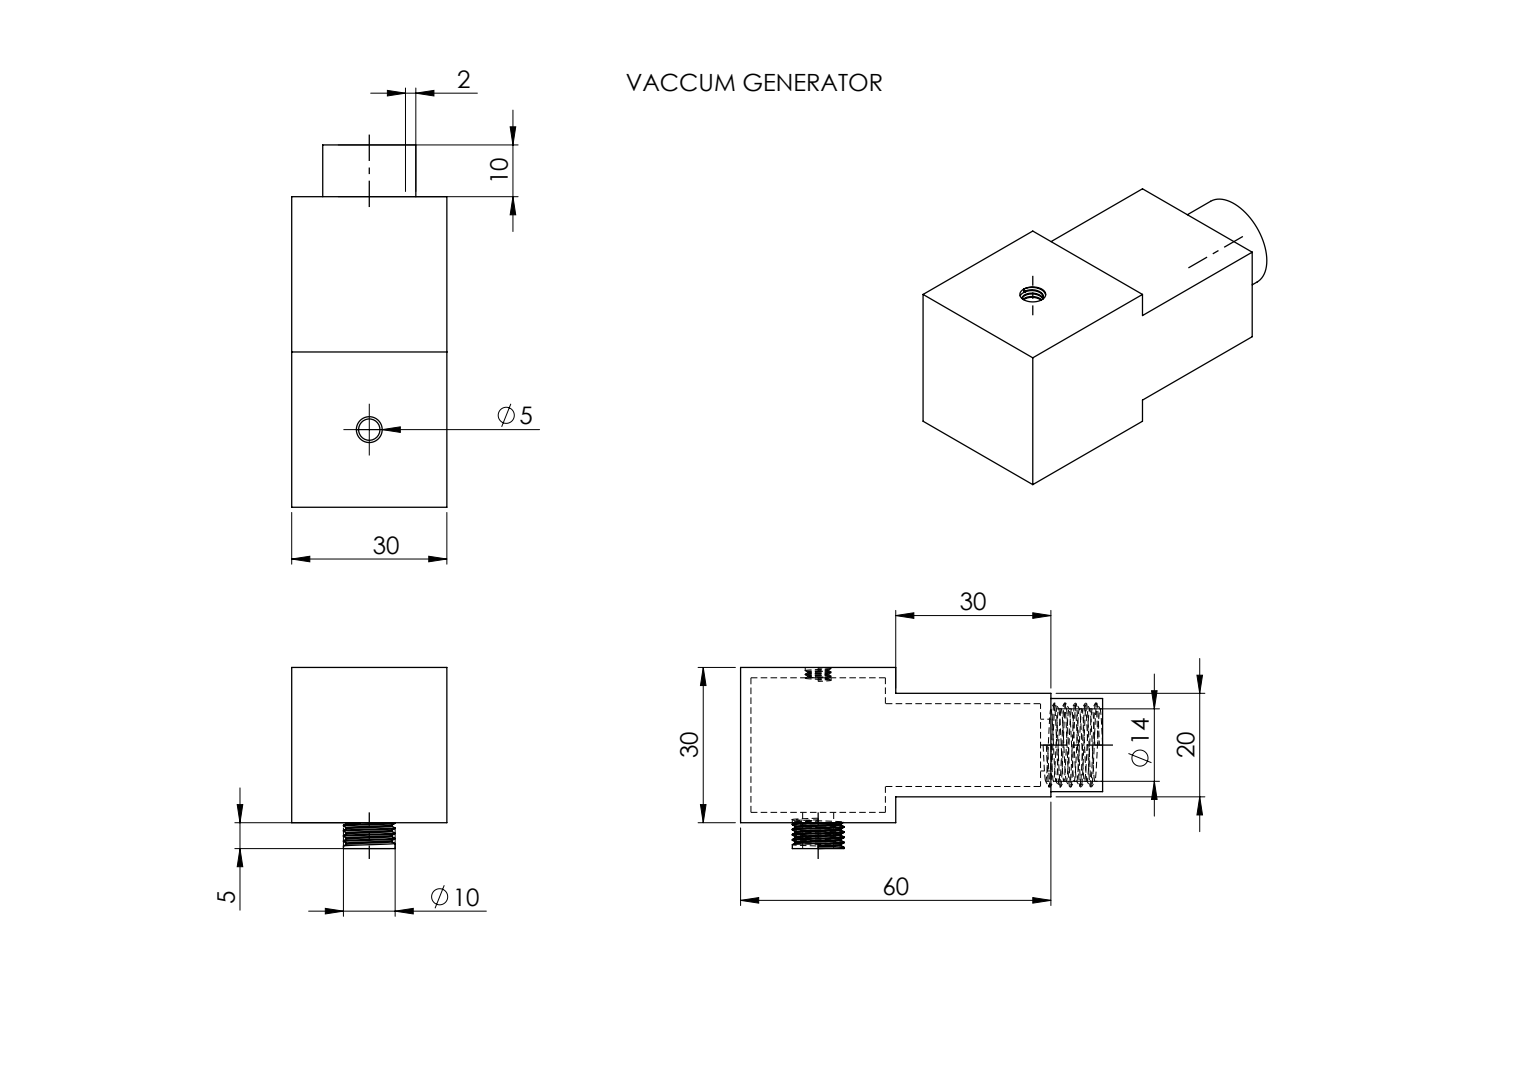
ISO-10303-21;
HEADER;
FILE_DESCRIPTION (('STEP AP214'),
    '1' );
FILE_NAME ('vaccum generator.step',
    '2026-10-01T14:18:43',
    ( '' ),
    ( '' ),
    'SwSTEP 2.0',
    'SolidWorks 2026',
    '' );
FILE_SCHEMA (( 'AUTOMOTIVE_DESIGN' ));
ENDSEC;

DATA;
#3=CARTESIAN_POINT ( 'NONE',  ( 103.1528011352953484, 93.43749999863440792, -3.152801135295366208 ) ) ;
#11=VERTEX_POINT ( 'NONE', #12909 ) ;
#21=VECTOR ( 'NONE', #21803, 1000.000000000000000 ) ;
#28=CARTESIAN_POINT ( 'NONE',  ( 104.9952793366501851, 116.8754121666685393, -49.82500000273120122 ) ) ;
#37=CARTESIAN_POINT ( 'NONE',  ( 102.0669872999999797, 123.3500000010924680, -9.794112055954760458E-15 ) ) ;
#38=LINE ( 'NONE', #22552, #12466 ) ;
#44=EDGE_CURVE ( 'NONE', #13519, #7822, #26113, .T. ) ;
#46=CARTESIAN_POINT ( 'NONE',  ( 93.00000000000001421, 112.2744378736303332, -50.10000000000000142 ) ) ;
#49=CARTESIAN_POINT ( 'NONE',  ( 97.93301269999999192, 123.9000000010924794, -0.8561741729129505041 ) ) ;
#53=CARTESIAN_POINT ( 'NONE',  ( 103.5355339059327235, 93.74999999726881583, 3.535533905932724874 ) ) ;
#67=( BOUNDED_CURVE ( )  B_SPLINE_CURVE ( 2, ( #19739, #26449, #6767, #8908, #2228, #15452, #13444, #6906, #10892, #17316, #24023, #2505, #15595, #2083, #2648, #15160, #20032, #19600, #512, #9193, #17887, #26593, #10752, #19463, #28160, #8627, #4357, #13014, #83, #8766, #26155, #15308, #18836, #13875, #8143, #13592, #5879, #15877, #16700, #11735, #22314, #20460, #11453, #942, #10262, #12398, #21119, #26883, #22601, #3070, #26736, #2788, #23265, #20986, #13733, #1606, #24872, #14549, #18972, #27680, #27543, #16017, #5355, #24587, #4929, #7329, #18022, #20174, #9613, #9328, #8000, #3738, #7180, #1467, #25399, #5069, #16837, #655, #16165, #22457, #2923, #10123, #18316, #14410, #27025, #11593, #20313, #7470, #800, #9469, #23126, #18171, #3601, #24731, #5211, #12261, #10683, #8842, #23398, #23956, #8558 ),
 .UNSPECIFIED., .F., .F. ) 
 B_SPLINE_CURVE_WITH_KNOTS ( ( 3, 2, 2, 2, 2, 2, 2, 2, 2, 2, 2, 2, 2, 2, 2, 2, 2, 2, 2, 2, 2, 2, 2, 2, 2, 2, 2, 2, 2, 2, 2, 2, 2, 2, 2, 2, 2, 2, 2, 2, 2, 2, 2, 2, 2, 2, 2, 2, 2, 2, 3 ),
 ( 0.000000000000000000, 0.02000000000000000042, 0.04000000000000000083, 0.05999999999999999778, 0.08000000000000000167, 0.1000000000000000056, 0.1199999999999999956, 0.1400000000000000133, 0.1600000000000000033, 0.1799999999999999933, 0.2000000000000000111, 0.2200000000000000011, 0.2399999999999999911, 0.2600000000000000089, 0.2800000000000000266, 0.2999999999999999889, 0.3200000000000000067, 0.3400000000000000244, 0.3599999999999999867, 0.3800000000000000044, 0.4000000000000000222, 0.4199999999999999845, 0.4400000000000000022, 0.4600000000000000200, 0.4799999999999999822, 0.5000000000000000000, 0.5200000000000000178, 0.5400000000000000355, 0.5600000000000000533, 0.5799999999999999600, 0.5999999999999999778, 0.6199999999999999956, 0.6400000000000000133, 0.6600000000000000311, 0.6800000000000000488, 0.6999999999999999556, 0.7199999999999999734, 0.7399999999999999911, 0.7600000000000000089, 0.7800000000000000266, 0.8000000000000000444, 0.8199999999999999512, 0.8399999999999999689, 0.8599999999999999867, 0.8800000000000000044, 0.9000000000000000222, 0.9200000000000000400, 0.9399999999999999467, 0.9599999999999999645, 0.9799999999999999822, 1.000000000000000000 ),
 .UNSPECIFIED. ) 
 CURVE ( )  GEOMETRIC_REPRESENTATION_ITEM ( )  RATIONAL_B_SPLINE_CURVE ( ( 1.000000000000000000, 0.9510565162951535312, 1.000000000000000000, 0.9510565162951535312, 1.000000000000000000, 0.9510565162951535312, 1.000000000000000000, 0.9510565162951535312, 1.000000000000000000, 0.9510565162951535312, 1.000000000000000000, 0.9510565162951535312, 1.000000000000000000, 0.9510565162951535312, 1.000000000000000000, 0.9510565162951535312, 1.000000000000000000, 0.9510565162951535312, 1.000000000000000000, 0.9510565162951535312, 1.000000000000000000, 0.9510565162951535312, 1.000000000000000000, 0.9510565162951535312, 1.000000000000000000, 0.9510565162951535312, 1.000000000000000000, 0.9510565162951535312, 1.000000000000000000, 0.9510565162951535312, 1.000000000000000000, 0.9510565162951535312, 1.000000000000000000, 0.9510565162951535312, 1.000000000000000000, 0.9510565162951535312, 1.000000000000000000, 0.9510565162951535312, 1.000000000000000000, 0.9510565162951535312, 1.000000000000000000, 0.9510565162951535312, 1.000000000000000000, 0.9510565162951535312, 1.000000000000000000, 0.9510565162951535312, 1.000000000000000000, 0.9510565162951535312, 1.000000000000000000, 0.9510565162951535312, 1.000000000000000000, 0.9510565162951535312, 1.000000000000000000, 0.9510565162951535312, 1.000000000000000000, 0.9510565162951535312, 1.000000000000000000, 0.9510565162951535312, 1.000000000000000000, 0.9510565162951535312, 1.000000000000000000, 0.9510565162951535312, 1.000000000000000000, 0.9510565162951535312, 1.000000000000000000, 0.9510565162951535312, 1.000000000000000000, 0.9510565162951535312, 1.000000000000000000, 0.9510565162951535312, 1.000000000000000000, 0.9510565162951535312, 1.000000000000000000, 0.9510565162951535312, 1.000000000000000000, 0.9510565162951535312, 1.000000000000000000, 0.9510565162951535312, 1.000000000000000000, 0.9510565162951535312, 1.000000000000000000, 0.9510565162951535312, 1.000000000000000000, 0.9510565162951535312, 1.000000000000000000, 0.9510565162951535312, 1.000000000000000000, 0.9510565162951535312, 1.000000000000000000, 0.9510565162951535312, 1.000000000000000000, 0.9510565162951535312, 1.000000000000000000, 0.9510565162951535312, 1.000000000000000000, 0.9510565162951535312, 1.000000000000000000, 0.9510565162951535312, 1.000000000000000000, 0.9510565162951535312, 1.000000000000000000 ) ) 
 REPRESENTATION_ITEM ( '' )  );
#71=EDGE_CURVE ( 'NONE', #7474, #9199, #1741, .T. ) ;
#83=CARTESIAN_POINT ( 'NONE',  ( 93.46109445667491400, 114.7507929638356785, -51.32500000273120122 ) ) ;
#86=CARTESIAN_POINT ( 'NONE',  ( 84.99999999999998579, 100.0000000000000000, -15.00000000000000533 ) ) ;
#87=CARTESIAN_POINT ( 'NONE',  ( 101.7677669529663547, 123.8000000021849587, 1.767766952966350891 ) ) ;
#93=CARTESIAN_POINT ( 'NONE',  ( 102.0669872999999797, 122.5500000010924850, -9.794112055954760458E-15 ) ) ;
#95=LINE ( 'NONE', #11320, #20973 ) ;
#101=CARTESIAN_POINT ( 'NONE',  ( 108.0825317500000011, 112.6261737610028320, -50.02500000273118275 ) ) ;
#116=EDGE_CURVE ( 'NONE', #24967, #25660, #21271, .T. ) ;
#120=CARTESIAN_POINT ( 'NONE',  ( 104.9999999999999716, 92.93749999999998579, 2.071067811865467956 ) ) ;
#125=CARTESIAN_POINT ( 'NONE',  ( 99.99999999999998579, 117.3602355696678643, -54.50000000000000000 ) ) ;
#129=CARTESIAN_POINT ( 'NONE',  ( 106.5389055433251002, 105.2492070361643215, -44.57500000273119412 ) ) ;
#130=CARTESIAN_POINT ( 'NONE',  ( 104.3262379212492590, 115.9545556584642867, -45.20000000546237828 ) ) ;
#133=CARTESIAN_POINT ( 'NONE',  ( 102.1631189606246295, 116.6573956140660897, -45.10000000546238397 ) ) ;
#134=CARTESIAN_POINT ( 'NONE',  ( 98.15313185440925281, 94.99999999863439371, 4.458734124999979898 ) ) ;
#142=CARTESIAN_POINT ( 'NONE',  ( 96.84719886470463734, 92.93749999863440792, 3.152801135295351997 ) ) ;
#155=UNCERTAINTY_MEASURE_WITH_UNIT (LENGTH_MEASURE( 1.000000000000000082E-05 ), #20072, 'distance_accuracy_value', 'NONE');
#159=CARTESIAN_POINT ( 'NONE',  ( 103.5355338419364699, 95.00000000000001421, -3.535533969929001596 ) ) ;
#171=CARTESIAN_POINT ( 'NONE',  ( 93.46109445667491400, 114.7507929638356785, -51.32500000273120122 ) ) ;
#179=CARTESIAN_POINT ( 'NONE',  ( 84.99999999999998579, 120.0000000000000000, -45.00000000000000711 ) ) ;
#182=EDGE_LOOP ( 'NONE', ( #354, #23980, #3469, #3062 ) ) ;
#187=CARTESIAN_POINT ( 'NONE',  ( 97.83688103937538472, 116.6573956140660897, -48.40000000000000568 ) ) ;
#189=FACE_OUTER_BOUND ( 'NONE', #22000, .T. ) ;
#192=CARTESIAN_POINT ( 'NONE',  ( 95.00000000000000000, 93.31249999726880162, -2.071067811865479058 ) ) ;
#196=ORIENTED_EDGE ( 'NONE', *, *, #21889, .T. ) ;
#210=VERTEX_POINT ( 'NONE', #12459 ) ;
#213=ORIENTED_EDGE ( 'NONE', *, *, #13961, .F. ) ;
#221=DIRECTION ( 'NONE',  ( 1.000000000000000000, 0.000000000000000000, 0.000000000000000000 ) ) ;
#225=CARTESIAN_POINT ( 'NONE',  ( 97.50000000000000000, 124.3184775928351655, 0.3826834323650784575 ) ) ;
#230=CARTESIAN_POINT ( 'NONE',  ( 101.0355339059327378, 122.4500000021849502, -2.499999999999997780 ) ) ;
#237=CARTESIAN_POINT ( 'NONE',  ( 91.91746824999998466, 107.3738262389971538, -51.02500000273119696 ) ) ;
#245=CARTESIAN_POINT ( 'NONE',  ( 112.9999999999999858, 120.0000000000000000, -43.00000000000000000 ) ) ;
#255=LINE ( 'NONE', #20201, #25320 ) ;
#264=DIRECTION ( 'NONE',  ( 0.000000000000000000, -1.000000000000000000, 0.000000000000000000 ) ) ;
#275=CARTESIAN_POINT ( 'NONE',  ( 102.4999999999999858, 123.0000000000000000, -8.724596124144689908E-15 ) ) ;
#276=ORIENTED_EDGE ( 'NONE', *, *, #2418, .F. ) ;
#286=CARTESIAN_POINT ( 'NONE',  ( 98.15313185440925281, 92.99999999863439371, 4.458734124999979898 ) ) ;
#288=EDGE_CURVE ( 'NONE', #11725, #11898, #16264, .T. ) ;
#312=CARTESIAN_POINT ( 'NONE',  ( 102.4976396683250925, 102.3130555110000159, -44.52500000273119696 ) ) ;
#314=FACE_OUTER_BOUND ( 'NONE', #8408, .T. ) ;
#322=CARTESIAN_POINT ( 'NONE',  ( 102.0669872999999797, 122.5500000010924850, -9.794112055954760458E-15 ) ) ;
#323=FACE_OUTER_BOUND ( 'NONE', #26669, .T. ) ;
#330=CARTESIAN_POINT ( 'NONE',  ( 95.00472066334982912, 116.8754121666685393, -51.67500000273118133 ) ) ;
#332=CARTESIAN_POINT ( 'NONE',  ( 101.4615807364564546, 122.8500000010924680, -1.461580736456474794 ) ) ;
#335=CARTESIAN_POINT ( 'NONE',  ( 96.46446609406726225, 92.24999999726880162, -3.535533905932738197 ) ) ;
#341=ORIENTED_EDGE ( 'NONE', *, *, #1476, .T. ) ;
#354=ORIENTED_EDGE ( 'NONE', *, *, #7968, .T. ) ;
#359=AXIS2_PLACEMENT_3D ( 'NONE', #24146, #26286, #22010 ) ;
#370=VERTEX_POINT ( 'NONE', #20912 ) ;
#372=CARTESIAN_POINT ( 'NONE',  ( 102.4999999999999858, 122.2813376356282191, 0.3865102666887284544 ) ) ;
#377=CARTESIAN_POINT ( 'NONE',  ( 99.99999999999998579, 122.9000000021849530, 2.499999999999978684 ) ) ;
#379=AXIS2_PLACEMENT_3D ( 'NONE', #4372, #22042, #19613 ) ;
#381=CARTESIAN_POINT ( 'NONE',  ( 84.99999999999998579, 99.99999999999998579, -45.00000000000000711 ) ) ;
#384=CARTESIAN_POINT ( 'NONE',  ( 99.99999999999998579, 118.4984768113314004, -53.62500000273119127 ) ) ;
#387=DIRECTION ( 'NONE',  ( 0.000000000000000000, 0.000000000000000000, -1.000000000000000000 ) ) ;
#419=CARTESIAN_POINT ( 'NONE',  ( 100.8031273896213378, 123.0000000000000000, 2.371931796629188405 ) ) ;
#420=CARTESIAN_POINT ( 'NONE',  ( 99.99999999999998579, 92.12499999726880162, -4.999999999999997335 ) ) ;
#427=CARTESIAN_POINT ( 'NONE',  ( 96.84719886470463734, 94.68749999863440792, -3.152801135295366208 ) ) ;
#429=CARTESIAN_POINT ( 'NONE',  ( 95.54126587499999346, 94.99999999863439371, -1.846868145590737864 ) ) ;
#434=DIRECTION ( 'NONE',  ( 0.000000000000000000, 1.000000000000000000, -1.156482317317871478E-16 ) ) ;
#446=EDGE_CURVE ( 'NONE', #27429, #27080, #21214, .T. ) ;
#455=CARTESIAN_POINT ( 'NONE',  ( 99.99999999999998579, 118.4984768113314004, -45.62500000273118417 ) ) ;
#464=CARTESIAN_POINT ( 'NONE',  ( 102.0669873000000081, 123.3000000010924850, 0.8561741729129311862 ) ) ;
#465=DIRECTION ( 'NONE',  ( 0.000000000000000000, 0.000000000000000000, 1.000000000000000000 ) ) ;
#471=VECTOR ( 'NONE', #27075, 1000.000000000000000 ) ;
#473=CARTESIAN_POINT ( 'NONE',  ( 107.0000000000000142, 110.0000000000000000, -47.00000000000000711 ) ) ;
#475=CARTESIAN_POINT ( 'NONE',  ( 101.0355339059327378, 123.1499999999999915, -2.499999999999997780 ) ) ;
#476=EDGE_CURVE ( 'NONE', #26599, #20388, #21898, .T. ) ;
#480=CARTESIAN_POINT ( 'NONE',  ( 104.9999999999999716, 94.81249999726880162, 2.071067811865467956 ) ) ;
#483=CARTESIAN_POINT ( 'NONE',  ( 108.0825317500000153, 110.0000000000000000, -52.37500000273119838 ) ) ;
#484=EDGE_CURVE ( 'NONE', #26503, #20101, #13985, .T. ) ;
#486=CARTESIAN_POINT ( 'NONE',  ( 102.4999999999999858, 123.1000000021849416, -9.847140817659276890E-15 ) ) ;
#490=( BOUNDED_CURVE ( )  B_SPLINE_CURVE ( 2, ( #3629, #3902, #12290, #3485, #23428, #25141, #19000, #10438, #9887 ),
 .UNSPECIFIED., .F., .F. ) 
 B_SPLINE_CURVE_WITH_KNOTS ( ( 3, 2, 2, 2, 3 ),
 ( 0.4500000000000003997, 0.4750000000000003664, 0.5000000000000004441, 0.5250000000000004663, 0.5500000000000004885 ),
 .UNSPECIFIED. ) 
 CURVE ( )  GEOMETRIC_REPRESENTATION_ITEM ( )  RATIONAL_B_SPLINE_CURVE ( ( 0.9999999999999987788, 0.9238795325112879597, 1.000000000000000000, 0.9238795325112867385, 1.000000000000000000, 0.9238795325112867385, 1.000000000000000000, 0.9238795325112854062, 1.000000000000001332 ) ) 
 REPRESENTATION_ITEM ( '' )  );
#493=EDGE_LOOP ( 'NONE', ( #21611, #13258, #8930, #18827, #22732, #24894, #25682, #24306 ) ) ;
#510=AXIS2_PLACEMENT_3D ( 'NONE', #5908, #18592, #16158 ) ;
#512=CARTESIAN_POINT ( 'NONE',  ( 106.5389055433251002, 105.2492070361643215, -52.32500000273119412 ) ) ;
#516=VECTOR ( 'NONE', #15597, 1000.000000000000000 ) ;
#519=CARTESIAN_POINT ( 'NONE',  ( 102.0669872999999797, 123.3500000010924680, -9.794112055954760458E-15 ) ) ;
#524=CARTESIAN_POINT ( 'NONE',  ( 93.00000000000000000, 110.0000000000000000, -52.50000000546237544 ) ) ;
#526=CARTESIAN_POINT ( 'NONE',  ( 108.0825317500000153, 110.0000000000000000, -46.12500000273119838 ) ) ;
#544=CARTESIAN_POINT ( 'NONE',  ( 102.4999999999999858, 123.9000000021849530, -9.847140817659276890E-15 ) ) ;
#545=DIRECTION ( 'NONE',  ( 0.000000000000000000, 0.000000000000000000, 1.000000000000000000 ) ) ;
#546=DIRECTION ( 'NONE',  ( 1.000000000000000000, 0.000000000000000000, -5.782411586589357392E-17 ) ) ;
#549=CARTESIAN_POINT ( 'NONE',  ( 102.4999999999999716, 124.5569999999781601, 1.035533905932722876 ) ) ;
#551=CARTESIAN_POINT ( 'NONE',  ( 95.00000000000000000, 94.43749999726878741, 2.071067811865463959 ) ) ;
#560=DIRECTION ( 'NONE',  ( 5.782411586589357392E-17, -0.000000000000000000, 1.000000000000000000 ) ) ;
#561=CARTESIAN_POINT ( 'NONE',  ( 84.99999999999998579, 102.0000000000000000, -43.00000000000000000 ) ) ;
#574=CARTESIAN_POINT ( 'NONE',  ( 99.99999999999998579, 93.25000000000000000, -4.999999999999997335 ) ) ;
#575=CARTESIAN_POINT ( 'NONE',  ( 104.4587341249999923, 94.62499999863439371, -1.846868145590737198 ) ) ;
#578=ORIENTED_EDGE ( 'NONE', *, *, #27721, .F. ) ;
#588=LINE ( 'NONE', #8843, #28012 ) ;
#592=DIRECTION ( 'NONE',  ( -5.782411586589357392E-17, 0.000000000000000000, -1.000000000000000000 ) ) ;
#597=CARTESIAN_POINT ( 'NONE',  ( 91.91746824999998466, 107.3738262389971538, -45.02500000273118985 ) ) ;
#598=CARTESIAN_POINT ( 'NONE',  ( 98.15313185440925281, 91.24999999863439371, 4.458734124999979898 ) ) ;
#602=VECTOR ( 'NONE', #8159, 1000.000000000000000 ) ;
#605=CARTESIAN_POINT ( 'NONE',  ( 104.4587341249999781, 90.56249999863440792, -6.938893903907228378E-15 ) ) ;
#606=EDGE_CURVE ( 'NONE', #15224, #13309, #67, .T. ) ;
#607=CARTESIAN_POINT ( 'NONE',  ( 99.99999999999998579, 123.7000000021849502, 2.499999999999978684 ) ) ;
#613=VERTEX_POINT ( 'NONE', #17102 ) ;
#614=CARTESIAN_POINT ( 'NONE',  ( 102.1631189606246295, 116.6573956140660897, -46.60000000000000142 ) ) ;
#616=CARTESIAN_POINT ( 'NONE',  ( 98.23223304703363112, 124.1000000000000085, -1.767766952966370209 ) ) ;
#622=( BOUNDED_CURVE ( )  B_SPLINE_CURVE ( 2, ( #23987, #4050, #21858, #21436, #25840, #8308, #4465, #8730, #16998 ),
 .UNSPECIFIED., .F., .T. ) 
 B_SPLINE_CURVE_WITH_KNOTS ( ( 3, 2, 2, 2, 3 ),
 ( 0.3500000000000003109, 0.3750000000000003331, 0.4000000000000003553, 0.4250000000000003775, 0.4500000000000003997 ),
 .UNSPECIFIED. ) 
 CURVE ( )  GEOMETRIC_REPRESENTATION_ITEM ( )  RATIONAL_B_SPLINE_CURVE ( ( 0.9999999999999990008, 0.9238795325112877377, 1.000000000000000000, 0.9238795325112867385, 1.000000000000000000, 0.9238795325112867385, 1.000000000000000000, 0.9238795325112855172, 1.000000000000001110 ) ) 
 REPRESENTATION_ITEM ( '' )  );
#623=CARTESIAN_POINT ( 'NONE',  ( 97.92893218813452449, 95.56249999726883004, 4.999999999999983125 ) ) ;
#626=CARTESIAN_POINT ( 'NONE',  ( 104.9952793366501709, 103.1245878333314465, -50.67500000273119554 ) ) ;
#628=DIRECTION ( 'NONE',  ( 0.000000000000000000, -1.000000000000000000, 0.000000000000000000 ) ) ;
#638=CARTESIAN_POINT ( 'NONE',  ( 99.99999999999998579, 91.31249999863440792, 4.458734124999981674 ) ) ;
#641=ORIENTED_EDGE ( 'NONE', *, *, #1027, .F. ) ;
#650=ORIENTED_EDGE ( 'NONE', *, *, #4627, .F. ) ;
#655=CARTESIAN_POINT ( 'NONE',  ( 104.9952793366501709, 103.1245878333314465, -46.42500000273119554 ) ) ;
#670=CARTESIAN_POINT ( 'NONE',  ( 96.84719886470463734, 92.68749999863440792, -3.152801135295366208 ) ) ;
#671=CARTESIAN_POINT ( 'NONE',  ( 108.0825317500000153, 110.0000000000000000, -48.12500000273119838 ) ) ;
#678=ORIENTED_EDGE ( 'NONE', *, *, #24104, .F. ) ;
#685=CYLINDRICAL_SURFACE ( 'NONE', #17971, 7.000000000000006217 ) ;
#689=AXIS2_PLACEMENT_3D ( 'NONE', #15191, #26185, #8519 ) ;
#693=CARTESIAN_POINT ( 'NONE',  ( 98.96446609406727646, 124.3569999999781430, 2.499999999999977796 ) ) ;
#697=DIRECTION ( 'NONE',  ( 0.000000000000000000, 0.000000000000000000, -1.000000000000000000 ) ) ;
#704=DIRECTION ( 'NONE',  ( 0.000000000000000000, 0.000000000000000000, 1.000000000000000000 ) ) ;
#706=CARTESIAN_POINT ( 'NONE',  ( 106.5389055433251002, 105.2492070361643215, -52.57500000273119412 ) ) ;
#716=CARTESIAN_POINT ( 'NONE',  ( 96.46446609406726225, 91.62500000000000000, 3.535533905932723986 ) ) ;
#723=CARTESIAN_POINT ( 'NONE',  ( 96.46446609406726225, 95.24999999726881583, -3.535533905932738197 ) ) ;
#724=B_SPLINE_CURVE_WITH_KNOTS ( 'NONE', 3,
 ( #27392, #24818, #7851, #20969 ),
 .UNSPECIFIED., .F., .F.,
 ( 4, 4 ),
 ( 0.000000000000000000, 1.000000000000000000 ),
 .UNSPECIFIED. ) ;
#730=LINE ( 'NONE', #20110, #16690 ) ;
#734=CARTESIAN_POINT ( 'NONE',  ( 107.0000000000000142, 110.0000000000000000, -49.50000000546238255 ) ) ;
#735=CARTESIAN_POINT ( 'NONE',  ( 101.8468681455907330, 91.49999999863440792, -4.458734124999994997 ) ) ;
#741=CARTESIAN_POINT ( 'NONE',  ( 93.00000000000000000, 110.0000000000000000, -52.50000000546237544 ) ) ;
#744=DIRECTION ( 'NONE',  ( -5.782411586589357392E-17, -0.000000000000000000, -1.000000000000000000 ) ) ;
#749=( BOUNDED_CURVE ( )  B_SPLINE_CURVE ( 2, ( #24281, #4762, #20290, #13422, #20439 ),
 .UNSPECIFIED., .F., .F. ) 
 B_SPLINE_CURVE_WITH_KNOTS ( ( 3, 2, 3 ),
 ( 0.000000000000000000, 0.02500000000000002220, 0.05000000000000004441 ),
 .UNSPECIFIED. ) 
 CURVE ( )  GEOMETRIC_REPRESENTATION_ITEM ( )  RATIONAL_B_SPLINE_CURVE ( ( 1.000000000000000000, 0.9238795325112867385, 1.000000000000000000, 0.9238795325112866275, 1.000000000000000222 ) ) 
 REPRESENTATION_ITEM ( '' )  );
#751=CARTESIAN_POINT ( 'NONE',  ( 97.50000000000000000, 123.4500000021849502, -1.035533905932742416 ) ) ;
#756=VERTEX_POINT ( 'NONE', #28095 ) ;
#757=CARTESIAN_POINT ( 'NONE',  ( 93.46109445667491400, 105.2492070361643215, -51.17500000273119554 ) ) ;
#760=CARTESIAN_POINT ( 'NONE',  ( 101.0355339059327378, 123.6500000000000199, 2.499999999999977796 ) ) ;
#761=CARTESIAN_POINT ( 'NONE',  ( 99.99999999999998579, 94.75000000000000000, 4.999999999999984013 ) ) ;
#765=CARTESIAN_POINT ( 'NONE',  ( 95.54126587499999346, 93.99999999863439371, -1.846868145590737864 ) ) ;
#767=CARTESIAN_POINT ( 'NONE',  ( 91.91746824999998466, 112.6261737610028320, -53.47500000273119980 ) ) ;
#776=CARTESIAN_POINT ( 'NONE',  ( 99.99999999999998579, 124.7999999999999972, -2.499999999999997780 ) ) ;
#783=CARTESIAN_POINT ( 'NONE',  ( 95.54126587500000767, 92.06249999863440792, -7.484931351350258973E-15 ) ) ;
#796=CARTESIAN_POINT ( 'NONE',  ( 99.99999999999998579, 91.62499999726880162, 4.999999999999984013 ) ) ;
#798=AXIS2_PLACEMENT_3D ( 'NONE', #21029, #12723, #5784 ) ;
#800=CARTESIAN_POINT ( 'NONE',  ( 93.46109445667491400, 114.7507929638356785, -45.32500000273119412 ) ) ;
#802=EDGE_CURVE ( 'NONE', #24847, #3863, #10819, .T. ) ;
#816=CARTESIAN_POINT ( 'NONE',  ( 99.99999999999998579, 118.4984768113314004, -47.62500000273119127 ) ) ;
#818=AXIS2_PLACEMENT_3D ( 'NONE', #8800, #11063, #545 ) ;
#821=CARTESIAN_POINT ( 'NONE',  ( 102.0710678118654613, 91.06249999726880162, -4.999999999999997335 ) ) ;
#823=ORIENTED_EDGE ( 'NONE', *, *, #16054, .F. ) ;
#850=EDGE_CURVE ( 'NONE', #21579, #8168, #25534, .T. ) ;
#855=DIRECTION ( 'NONE',  ( 1.000000000000000000, 0.000000000000000000, -5.782411586589357392E-17 ) ) ;
#856=CARTESIAN_POINT ( 'NONE',  ( 102.1049798866730214, 123.0000000000000284, -1.357224074530030800 ) ) ;
#857=EDGE_LOOP ( 'NONE', ( #26118, #7258, #9956, #20270 ) ) ;
#858=CARTESIAN_POINT ( 'NONE',  ( 102.0669872999999797, 124.1500000010924794, -9.794112055954760458E-15 ) ) ;
#865=CARTESIAN_POINT ( 'NONE',  ( 99.99999999999998579, 92.75000000000000000, 4.999999999999984013 ) ) ;
#867=VECTOR ( 'NONE', #8438, 1000.000000000000000 ) ;
#882=CARTESIAN_POINT ( 'NONE',  ( 93.00000000000000000, 110.0000000000000000, -50.50000000546237544 ) ) ;
#886=CARTESIAN_POINT ( 'NONE',  ( 99.99999999999998579, 124.3999999999999915, 2.499999999999978684 ) ) ;
#890=CARTESIAN_POINT ( 'NONE',  ( 104.9952793366501851, 116.8754121666685393, -45.82500000273119412 ) ) ;
#892=CARTESIAN_POINT ( 'NONE',  ( 104.4587341249999923, 91.49999999863440792, 1.846868145590726318 ) ) ;
#897=CARTESIAN_POINT ( 'NONE',  ( 102.3917468249999700, 122.9375000002731184, -9.833883627233146598E-15 ) ) ;
#905=CARTESIAN_POINT ( 'NONE',  ( 106.5389055433251002, 114.7507929638356785, -52.17500000273119554 ) ) ;
#913=CARTESIAN_POINT ( 'NONE',  ( 104.4587341249999781, 92.56249999863440792, -6.938893903907228378E-15 ) ) ;
#915=CARTESIAN_POINT ( 'NONE',  ( 108.0825317500000011, 107.3738262389971680, -48.47500000273118559 ) ) ;
#919=( BOUNDED_CURVE ( )  B_SPLINE_CURVE ( 2, ( #11916, #9919, #25049, #22918, #18636, #14478, #15162, #6218, #16897 ),
 .UNSPECIFIED., .F., .F. ) 
 B_SPLINE_CURVE_WITH_KNOTS ( ( 3, 2, 2, 2, 3 ),
 ( 0.2499999999999998335, 0.2916666666666665741, 0.3333333333333332593, 0.3750000000000000000, 0.4166666666666667407 ),
 .UNSPECIFIED. ) 
 CURVE ( )  GEOMETRIC_REPRESENTATION_ITEM ( )  RATIONAL_B_SPLINE_CURVE ( ( 1.000000000000000222, 0.9238795325112864054, 1.000000000000000000, 0.9238795325112867385, 1.000000000000000000, 0.9238795325112867385, 1.000000000000000000, 0.9238795325112866275, 1.000000000000000000 ) ) 
 REPRESENTATION_ITEM ( '' )  );
#923=VERTEX_POINT ( 'NONE', #159 ) ;
#926=DIRECTION ( 'NONE',  ( 0.000000000000000000, -1.000000000000000000, 0.000000000000000000 ) ) ;
#938=LINE ( 'NONE', #9609, #7507 ) ;
#942=CARTESIAN_POINT ( 'NONE',  ( 104.9952793366501709, 116.8754121666685393, -49.82500000273120122 ) ) ;
#953=CARTESIAN_POINT ( 'NONE',  ( 104.9999999999999716, 94.93749999726880162, -2.071067811865478170 ) ) ;
#955=FACE_OUTER_BOUND ( 'NONE', #4282, .T. ) ;
#957=CARTESIAN_POINT ( 'NONE',  ( 99.99999999999998579, 101.5015231886685854, -46.62500000273119838 ) ) ;
#966=( BOUNDED_CURVE ( )  B_SPLINE_CURVE ( 2, ( #4156, #10263, #18973, #1885, #12817, #21539, #27681, #2016, #10684, #19391, #25951 ),
 .UNSPECIFIED., .F., .F. ) 
 B_SPLINE_CURVE_WITH_KNOTS ( ( 3, 2, 2, 2, 2, 3 ),
 ( 0.3000000000000002109, 0.3200000000000002287, 0.3400000000000003020, 0.3600000000000002642, 0.3800000000000003375, 0.4000000000000003553 ),
 .UNSPECIFIED. ) 
 CURVE ( )  GEOMETRIC_REPRESENTATION_ITEM ( )  RATIONAL_B_SPLINE_CURVE ( ( 0.9999999999999994449, 0.9510565162951540863, 1.000000000000000000, 0.9510565162951535312, 1.000000000000000000, 0.9510565162951535312, 1.000000000000000000, 0.9510565162951535312, 1.000000000000000000, 0.9510565162951527540, 1.000000000000000888 ) ) 
 REPRESENTATION_ITEM ( '' )  );
#986=LINE ( 'NONE', #24204, #26829 ) ;
#997=CARTESIAN_POINT ( 'NONE',  ( 99.99999999999998579, 118.4984768113314004, -53.87500000273118417 ) ) ;
#1003=EDGE_CURVE ( 'NONE', #11898, #11725, #6213, .T. ) ;
#1004=EDGE_LOOP ( 'NONE', ( #28123, #4594, #14143, #20923 ) ) ;
#1005=CARTESIAN_POINT ( 'NONE',  ( 99.99999999999998579, 117.3602355696678643, -50.49999999999999289 ) ) ;
#1008=CARTESIAN_POINT ( 'NONE',  ( 104.9999999999999858, 93.00000000000000000, -6.938893903907228378E-15 ) ) ;
#1026=CARTESIAN_POINT ( 'NONE',  ( 98.15313185440923860, 92.62499999863439371, -4.458734124999994997 ) ) ;
#1027=EDGE_CURVE ( 'NONE', #12839, #23013, #730, .T. ) ;
#1033=CARTESIAN_POINT ( 'NONE',  ( 104.3262379212492590, 104.0454443415356991, -49.80000000546237970 ) ) ;
#1047=CARTESIAN_POINT ( 'NONE',  ( 104.9952793366501851, 116.8754121666685393, -46.07500000273119412 ) ) ;
#1054=CARTESIAN_POINT ( 'NONE',  ( 96.84719886470463734, 93.18749999863440792, 3.152801135295351997 ) ) ;
#1055=FACE_OUTER_BOUND ( 'NONE', #17673, .T. ) ;
#1056=CARTESIAN_POINT ( 'NONE',  ( 104.9952793366501709, 116.8754121666685393, -50.07500000273120122 ) ) ;
#1077=CARTESIAN_POINT ( 'NONE',  ( 99.99999999999998579, 122.9500000010924765, -2.066987299999998751 ) ) ;
#1082=CARTESIAN_POINT ( 'NONE',  ( 95.00000000000000000, 91.37499999726880162, -7.551217303480904118E-15 ) ) ;
#1087=FACE_OUTER_BOUND ( 'NONE', #25613, .T. ) ;
#1091=ORIENTED_EDGE ( 'NONE', *, *, #15947, .T. ) ;
#1104=CARTESIAN_POINT ( 'NONE',  ( 104.9999999999999716, 90.93749999726880162, -2.071067811865478170 ) ) ;
#1127=CARTESIAN_POINT ( 'NONE',  ( 97.71650635000000307, 124.8750000005462368, -9.540979117872439019E-15 ) ) ;
#1140=CARTESIAN_POINT ( 'NONE',  ( 104.4587341249999781, 95.31249999863440792, -6.938893903907228378E-15 ) ) ;
#1142=CARTESIAN_POINT ( 'NONE',  ( 97.93301269999999192, 123.7000000010924765, -0.8561741729129505041 ) ) ;
#1150=CARTESIAN_POINT ( 'NONE',  ( 104.9999999999999716, 91.06249999999997158, -2.071067811865478170 ) ) ;
#1167=CARTESIAN_POINT ( 'NONE',  ( 101.8468681455907330, 91.12499999863439371, 4.458734124999980786 ) ) ;
#1175=CARTESIAN_POINT ( 'NONE',  ( 102.1631189606246295, 116.6573956140660897, -49.10000000546237686 ) ) ;
#1176=CARTESIAN_POINT ( 'NONE',  ( 104.4587341249999923, 93.49999999863442213, 1.846868145590726318 ) ) ;
#1178=LINE ( 'NONE', #18689, #2546 ) ;
#1189=VERTEX_POINT ( 'NONE', #19650 ) ;
#1190=CARTESIAN_POINT ( 'NONE',  ( 108.0825317500000153, 110.0000000000000000, -48.37500000273119838 ) ) ;
#1192=DIRECTION ( 'NONE',  ( 0.000000000000000000, 0.000000000000000000, 1.000000000000000000 ) ) ;
#1197=CARTESIAN_POINT ( 'NONE',  ( 101.8468681455907330, 90.74999999863439371, -4.458734124999994997 ) ) ;
#1208=ORIENTED_EDGE ( 'NONE', *, *, #12780, .T. ) ;
#1211=CARTESIAN_POINT ( 'NONE',  ( 103.1528011352953484, 93.68749999863440792, -3.152801135295366208 ) ) ;
#1214=DIRECTION ( 'NONE',  ( 0.000000000000000000, -1.000000000000000000, 3.469446951953611231E-16 ) ) ;
#1216=VECTOR ( 'NONE', #28178, 999.9999999999998863 ) ;
#1220=CARTESIAN_POINT ( 'NONE',  ( 108.0825317500000153, 110.0000000000000000, -54.25000000273119838 ) ) ;
#1232=( NAMED_UNIT ( * ) SI_UNIT ( $, .STERADIAN. ) SOLID_ANGLE_UNIT ( ) );
#1239=CARTESIAN_POINT ( 'NONE',  ( 87.00000000000000000, 123.0000000000000000, 14.99999999999999112 ) ) ;
#1243=ORIENTED_EDGE ( 'NONE', *, *, #7208, .F. ) ;
#1251=ADVANCED_FACE ( 'NONE', ( #2837, #13927 ), #2972, .F. ) ;
#1254=CARTESIAN_POINT ( 'NONE',  ( 107.0000000000000142, 110.0000000000000000, -47.00000000000000711 ) ) ;
#1259=CARTESIAN_POINT ( 'NONE',  ( 102.4999999999999858, 123.0000000000000000, -9.847140817659276890E-15 ) ) ;
#1273=CARTESIAN_POINT ( 'NONE',  ( 97.50236033167492167, 117.6869444889999841, -47.77500000273119696 ) ) ;
#1275=CARTESIAN_POINT ( 'NONE',  ( 97.93301269999999192, 124.5000000010924879, -0.8561741729129505041 ) ) ;
#1281=DIRECTION ( 'NONE',  ( 0.000000000000000000, 1.000000000000000000, 0.000000000000000000 ) ) ;
#1287=VERTEX_POINT ( 'NONE', #1140 ) ;
#1305=CARTESIAN_POINT ( 'NONE',  ( 107.0000000000000142, 107.7255621263696526, -49.60000000546238397 ) ) ;
#1306=CARTESIAN_POINT ( 'NONE',  ( 95.54126587500000767, 93.06249999863440792, -7.484931351350258973E-15 ) ) ;
#1318=EDGE_CURVE ( 'NONE', #3280, #28194, #19784, .T. ) ;
#1322=EDGE_LOOP ( 'NONE', ( #4647, #13285, #16586, #4240 ) ) ;
#1323=CARTESIAN_POINT ( 'NONE',  ( 93.46109445667491400, 105.2492070361643215, -49.17500000273119554 ) ) ;
#1332=CARTESIAN_POINT ( 'NONE',  ( 104.4587341249999923, 92.49999999863442213, 1.846868145590726318 ) ) ;
#1335=DIRECTION ( 'NONE',  ( 0.000000000000000000, 0.000000000000000000, -1.000000000000000000 ) ) ;
#1349=ADVANCED_FACE ( 'NONE', ( #7672 ), #27789, .T. ) ;
#1351=DIRECTION ( 'NONE',  ( 1.000000000000000000, 0.000000000000000000, 0.000000000000000000 ) ) ;
#1352=ORIENTED_EDGE ( 'NONE', *, *, #16537, .F. ) ;
#1360=CARTESIAN_POINT ( 'NONE',  ( 95.67376207875072680, 115.9545556584642867, -54.30000000000001137 ) ) ;
#1362=DIRECTION ( 'NONE',  ( 0.000000000000000000, -0.000000000000000000, 1.000000000000000000 ) ) ;
#1373=CARTESIAN_POINT ( 'NONE',  ( 104.3262379212492590, 104.0454443415356991, -51.80000000546237970 ) ) ;
#1375=CARTESIAN_POINT ( 'NONE',  ( 102.0710678118654613, 91.68749999726880162, 4.999999999999974243 ) ) ;
#1381=ORIENTED_EDGE ( 'NONE', *, *, #16100, .T. ) ;
#1382=VECTOR ( 'NONE', #2864, 1000.000000000000000 ) ;
#1383=VERTEX_POINT ( 'NONE', #1545 ) ;
#1399=CARTESIAN_POINT ( 'NONE',  ( 99.99999999999998579, 124.7999999999999972, -2.499999999999997780 ) ) ;
#1411=DIRECTION ( 'NONE',  ( 5.782411586589357392E-17, 0.000000000000000000, 1.000000000000000000 ) ) ;
#1414=CARTESIAN_POINT ( 'NONE',  ( 91.91746824999998466, 112.6261737610028320, -51.47500000273119980 ) ) ;
#1415=CARTESIAN_POINT ( 'NONE',  ( 104.9999999999999716, 94.06250000000000000, -2.071067811865478170 ) ) ;
#1417=CARTESIAN_POINT ( 'NONE',  ( 99.99999999999998579, 123.3500000010924680, 2.066987299999980099 ) ) ;
#1430=ORIENTED_EDGE ( 'NONE', *, *, #18321, .F. ) ;
#1440=CARTESIAN_POINT ( 'NONE',  ( 95.54126587499999346, 93.74999999863439371, -1.846868145590737864 ) ) ;
#1444=CARTESIAN_POINT ( 'NONE',  ( 100.0000000000000000, 110.0000000000000000, -55.00000000000000711 ) ) ;
#1449=CARTESIAN_POINT ( 'NONE',  ( 99.99999999999998579, 102.6397644303321215, -46.00000000546238255 ) ) ;
#1450=CARTESIAN_POINT ( 'NONE',  ( 104.4587341249999923, 90.37499999863440792, -1.846868145590737198 ) ) ;
#1452=LINE ( 'NONE', #25516, #24843 ) ;
#1454=ORIENTED_EDGE ( 'NONE', *, *, #17510, .T. ) ;
#1456=CARTESIAN_POINT ( 'NONE',  ( 114.9999999999999858, 99.99999999999998579, -45.00000000000000711 ) ) ;
#1462=CARTESIAN_POINT ( 'NONE',  ( 108.0825317500000153, 110.0000000000000000, -44.37500000273119838 ) ) ;
#1463=( BOUNDED_CURVE ( )  B_SPLINE_CURVE ( 2, ( #3272, #22370, #11799, #20523, #11941, #1005, #20662, #22231, #2710, #12486, #18925 ),
 .UNSPECIFIED., .F., .F. ) 
 B_SPLINE_CURVE_WITH_KNOTS ( ( 3, 2, 2, 2, 2, 3 ),
 ( 0.4000000000000003553, 0.4200000000000002065, 0.4400000000000000577, 0.4599999999999999645, 0.4799999999999997602, 0.4999999999999996669 ),
 .UNSPECIFIED. ) 
 CURVE ( )  GEOMETRIC_REPRESENTATION_ITEM ( )  RATIONAL_B_SPLINE_CURVE ( ( 0.9999999999999992228, 0.9510565162951543083, 1.000000000000000000, 0.9510565162951535312, 1.000000000000000000, 0.9510565162951535312, 1.000000000000000000, 0.9510565162951535312, 1.000000000000000000, 0.9510565162951543083, 0.9999999999999992228 ) ) 
 REPRESENTATION_ITEM ( '' )  );
#1467=CARTESIAN_POINT ( 'NONE',  ( 95.00472066334981491, 103.1245878333314465, -46.82500000273118701 ) ) ;
#1476=EDGE_CURVE ( 'NONE', #8561, #27429, #3939, .T. ) ;
#1484=CARTESIAN_POINT ( 'NONE',  ( 97.93301270000000613, 123.8000000010924566, 0.8561741729129328515 ) ) ;
#1485=CARTESIAN_POINT ( 'NONE',  ( 99.99999999999998579, 95.31249999863440792, 4.458734124999981674 ) ) ;
#1502=CARTESIAN_POINT ( 'NONE',  ( 104.9999999999999716, 90.06249999999998579, -2.071067811865478170 ) ) ;
#1505=EDGE_CURVE ( 'NONE', #756, #13519, #5408, .T. ) ;
#1510=EDGE_CURVE ( 'NONE', #3788, #10198, #24708, .T. ) ;
#1512=CARTESIAN_POINT ( 'NONE',  ( 102.0669872999999797, 122.7500000010924737, -9.794112055954760458E-15 ) ) ;
#1514=DIRECTION ( 'NONE',  ( 1.000000000000000000, -0.000000000000000000, -5.782411586589357392E-17 ) ) ;
#1516=CARTESIAN_POINT ( 'NONE',  ( 103.5355339059327235, 93.99999999726881583, -3.535533905932738197 ) ) ;
#1524=ORIENTED_EDGE ( 'NONE', *, *, #2921, .T. ) ;
#1538=CARTESIAN_POINT ( 'NONE',  ( 98.23223304703363112, 123.3069999999781459, -1.767766952966370209 ) ) ;
#1540=CARTESIAN_POINT ( 'NONE',  ( 101.4615807364564546, 124.4500000010924765, -1.461580736456474794 ) ) ;
#1542=( BOUNDED_CURVE ( )  B_SPLINE_CURVE ( 2, ( #3779, #12436, #18609, #21027, #7771, #19010, #8743, #12991, #15573 ),
 .UNSPECIFIED., .F., .F. ) 
 B_SPLINE_CURVE_WITH_KNOTS ( ( 3, 2, 2, 2, 3 ),
 ( 0.1500000000000001332, 0.1750000000000001554, 0.2000000000000001776, 0.2250000000000001998, 0.2500000000000002220 ),
 .UNSPECIFIED. ) 
 CURVE ( )  GEOMETRIC_REPRESENTATION_ITEM ( )  RATIONAL_B_SPLINE_CURVE ( ( 0.9999999999999995559, 0.9238795325112871826, 1.000000000000000000, 0.9238795325112867385, 1.000000000000000000, 0.9238795325112867385, 1.000000000000000000, 0.9238795325112860723, 1.000000000000000666 ) ) 
 REPRESENTATION_ITEM ( '' )  );
#1545=CARTESIAN_POINT ( 'NONE',  ( 107.0000000000000142, 110.0000000000000000, -51.00000000000000711 ) ) ;
#1555=CARTESIAN_POINT ( 'NONE',  ( 95.00472066334982912, 103.1245878333314323, -51.07500000273118701 ) ) ;
#1556=CARTESIAN_POINT ( 'NONE',  ( 102.0710678118655039, 93.81250000000000000, 4.999999999999940492 ) ) ;
#1557=CARTESIAN_POINT ( 'NONE',  ( 99.99999999999998579, 124.5500000010924708, -2.066987299999998751 ) ) ;
#1558=DIRECTION ( 'NONE',  ( 0.000000000000000000, 0.000000000000000000, 1.000000000000000000 ) ) ;
#1579=CARTESIAN_POINT ( 'NONE',  ( 104.4587341249999781, 93.31249999863440792, -6.938893903907228378E-15 ) ) ;
#1588=CARTESIAN_POINT ( 'NONE',  ( 102.1631189606246295, 103.3426043859339103, -51.90000000546238113 ) ) ;
#1589=CARTESIAN_POINT ( 'NONE',  ( 104.4587341249999781, 94.56249999863440792, -6.938893903907228378E-15 ) ) ;
#1595=CARTESIAN_POINT ( 'NONE',  ( 101.8468681455907330, 91.12499999863439371, 4.458734124999979898 ) ) ;
#1597=ORIENTED_EDGE ( 'NONE', *, *, #44, .F. ) ;
#1602=CARTESIAN_POINT ( 'NONE',  ( 106.5389055433251002, 114.7507929638356785, -46.17500000273119554 ) ) ;
#1606=CARTESIAN_POINT ( 'NONE',  ( 99.99999999999998579, 101.5015231886685712, -48.62500000273119838 ) ) ;
#1608=CIRCLE ( 'NONE', #13387, 4.999999999999989342 ) ;
#1611=FACE_OUTER_BOUND ( 'NONE', #17106, .T. ) ;
#1619=DIRECTION ( 'NONE',  ( 1.000000000000000000, -0.000000000000000000, -5.782411586589357392E-17 ) ) ;
#1622=CARTESIAN_POINT ( 'NONE',  ( 101.4615807364564546, 124.2500000010924879, -1.461580736456474794 ) ) ;
#1634=VECTOR ( 'NONE', #11959, 1000.000000000000114 ) ;
#1647=DIRECTION ( 'NONE',  ( 0.000000000000000000, -1.000000000000000000, -0.000000000000000000 ) ) ;
#1653=EDGE_CURVE ( 'NONE', #19205, #1889, #9028, .T. ) ;
#1673=CARTESIAN_POINT ( 'NONE',  ( 87.00000000000000000, 97.00000000000000000, 14.99999999999999467 ) ) ;
#1674=CARTESIAN_POINT ( 'NONE',  ( 98.96446609406727646, 123.5569999999781459, 2.499999999999977796 ) ) ;
#1676=CARTESIAN_POINT ( 'NONE',  ( 100.8561741729129437, 123.4000000010924509, 2.066987299999979655 ) ) ;
#1685=DIRECTION ( 'NONE',  ( 0.000000000000000000, 0.000000000000000000, 1.000000000000000000 ) ) ;
#1688=CARTESIAN_POINT ( 'NONE',  ( 106.5389055433251002, 114.7507929638356785, -48.17500000273120264 ) ) ;
#1692=CARTESIAN_POINT ( 'NONE',  ( 97.93301270000000613, 123.9500000010924765, -9.540979117872439019E-15 ) ) ;
#1700=CARTESIAN_POINT ( 'NONE',  ( 102.0710678118654613, 94.81249999999998579, 4.999999999999983125 ) ) ;
#1708=( BOUNDED_CURVE ( )  B_SPLINE_CURVE ( 2, ( #10650, #19637, #12913, #120, #4534, #13197, #2408, #11068, #8945 ),
 .UNSPECIFIED., .F., .F. ) 
 B_SPLINE_CURVE_WITH_KNOTS ( ( 3, 2, 2, 2, 3 ),
 ( 0.5500000000000004885, 0.5750000000000003997, 0.6000000000000005329, 0.6250000000000005551, 0.6500000000000005773 ),
 .UNSPECIFIED. ) 
 CURVE ( )  GEOMETRIC_REPRESENTATION_ITEM ( )  RATIONAL_B_SPLINE_CURVE ( ( 0.9999999999999986677, 0.9238795325112880708, 1.000000000000000000, 0.9238795325112867385, 1.000000000000000000, 0.9238795325112867385, 1.000000000000000000, 0.9238795325112850731, 1.000000000000001776 ) ) 
 REPRESENTATION_ITEM ( '' )  );
#1714=CARTESIAN_POINT ( 'NONE',  ( 99.99999999999998579, 93.56249999863440792, -4.458734124999994997 ) ) ;
#1723=CARTESIAN_POINT ( 'NONE',  ( 96.84719886470463734, 94.18749999863440792, 3.152801135295351997 ) ) ;
#1726=CARTESIAN_POINT ( 'NONE',  ( 93.00000000000000000, 110.0000000000000000, -46.00000000000000711 ) ) ;
#1727=ORIENTED_EDGE ( 'NONE', *, *, #14552, .F. ) ;
#1730=CARTESIAN_POINT ( 'NONE',  ( 103.1528011352953484, 91.43749999863440792, -3.152801135295366208 ) ) ;
#1741=( BOUNDED_CURVE ( )  B_SPLINE_CURVE ( 2, ( #23362, #21084, #12781, #16798, #25630, #3703, #6111, #16665, #12365, #3834, #25361 ),
 .UNSPECIFIED., .F., .F. ) 
 B_SPLINE_CURVE_WITH_KNOTS ( ( 3, 2, 2, 2, 2, 3 ),
 ( 0.2000000000000001776, 0.2200000000000001676, 0.2400000000000001854, 0.2600000000000002309, 0.2800000000000002487, 0.3000000000000002109 ),
 .UNSPECIFIED. ) 
 CURVE ( )  GEOMETRIC_REPRESENTATION_ITEM ( )  RATIONAL_B_SPLINE_CURVE ( ( 0.9999999999999995559, 0.9510565162951539753, 1.000000000000000000, 0.9510565162951535312, 1.000000000000000000, 0.9510565162951535312, 1.000000000000000000, 0.9510565162951535312, 1.000000000000000000, 0.9510565162951529761, 1.000000000000000444 ) ) 
 REPRESENTATION_ITEM ( '' )  );
#1751=CARTESIAN_POINT ( 'NONE',  ( 102.1631189606246295, 116.6573956140660897, -46.60000000000000142 ) ) ;
#1759=ORIENTED_EDGE ( 'NONE', *, *, #25499, .F. ) ;
#1760=LINE ( 'NONE', #12550, #16351 ) ;
#1762=CARTESIAN_POINT ( 'NONE',  ( 104.4587341249999923, 94.49999999863439371, 1.846868145590726318 ) ) ;
#1765=CARTESIAN_POINT ( 'NONE',  ( 87.00000000000000000, 125.0000000000000000, -13.00000000000000888 ) ) ;
#1766=ORIENTED_EDGE ( 'NONE', *, *, #21989, .F. ) ;
#1775=CIRCLE ( 'NONE', #2235, 2.999999999999989786 ) ;
#1789=CARTESIAN_POINT ( 'NONE',  ( 102.4999999999999858, 123.0500000000000114, -1.035533905932742638 ) ) ;
#1805=CARTESIAN_POINT ( 'NONE',  ( 99.99999999999998579, 90.00000000000000000, -6.938893903907228378E-15 ) ) ;
#1810=CARTESIAN_POINT ( 'NONE',  ( 97.50000000000000000, 124.2000000000000028, -9.540979117872439019E-15 ) ) ;
#1813=CARTESIAN_POINT ( 'NONE',  ( 99.14382582708708469, 123.3000000010924708, 2.066987299999979655 ) ) ;
#1825=CARTESIAN_POINT ( 'NONE',  ( 91.91746824999998466, 107.3738262389971538, -47.27500000273118275 ) ) ;
#1830=CARTESIAN_POINT ( 'NONE',  ( 97.93301269999999192, 122.9000000010924936, -0.8561741729129505041 ) ) ;
#1834=ORIENTED_EDGE ( 'NONE', *, *, #7584, .T. ) ;
#1837=DIRECTION ( 'NONE',  ( 0.000000000000000000, -1.000000000000000000, 0.000000000000000000 ) ) ;
#1846=ADVANCED_FACE ( 'NONE', ( #10130 ), #18842, .F. ) ;
#1847=CARTESIAN_POINT ( 'NONE',  ( 99.99999999999998579, 117.3602355696678643, -47.00000000546238255 ) ) ;
#1853=CARTESIAN_POINT ( 'NONE',  ( 98.15313185440923860, 92.99999999863439371, 4.458734124999980786 ) ) ;
#1857=PRODUCT_CONTEXT ( 'NONE', #6415, 'mechanical' ) ;
#1862=CARTESIAN_POINT ( 'NONE',  ( 99.99999999999998579, 117.3602355696678501, -45.00000000546238255 ) ) ;
#1863=CARTESIAN_POINT ( 'NONE',  ( 103.1528011352953484, 94.18749999863440792, 3.152801135295352886 ) ) ;
#1866=CARTESIAN_POINT ( 'NONE',  ( 105.6631189606246295, 105.8855032339526758, -45.20000000000000284 ) ) ;
#1885=CARTESIAN_POINT ( 'NONE',  ( 95.67376207875072680, 104.0454443415356991, -51.70000000000001705 ) ) ;
#1889=VERTEX_POINT ( 'NONE', #21693 ) ;
#1891=DIRECTION ( 'NONE',  ( 0.000000000000000000, -1.000000000000000000, 3.469446951953611231E-16 ) ) ;
#1894=CARTESIAN_POINT ( 'NONE',  ( 108.0825317500000011, 107.3738262389971538, -50.22500000273118559 ) ) ;
#1903=CARTESIAN_POINT ( 'NONE',  ( 99.14382582708708469, 123.9000000010924794, 2.066987299999979655 ) ) ;
#1914=CARTESIAN_POINT ( 'NONE',  ( 105.6631189606246295, 105.8855032339526758, -51.20000000000000995 ) ) ;
#1916=CARTESIAN_POINT ( 'NONE',  ( 98.53841926354351699, 124.6500000010924651, -1.461580736456474794 ) ) ;
#1921=ORIENTED_EDGE ( 'NONE', *, *, #18755, .F. ) ;
#1929=PLANE ( 'NONE',  #20036 ) ;
#1945=EDGE_CURVE ( 'NONE', #5360, #20854, #20129, .T. ) ;
#1948=CARTESIAN_POINT ( 'NONE',  ( 102.4999999999999858, 123.1000000021849416, -9.847140817659276890E-15 ) ) ;
#1951=CARTESIAN_POINT ( 'NONE',  ( 105.6631189606246295, 105.8855032339526758, -47.70000000546237828 ) ) ;
#1952=ORIENTED_EDGE ( 'NONE', *, *, #18274, .F. ) ;
#1953=CARTESIAN_POINT ( 'NONE',  ( 97.50000000000000000, 123.4500000021849502, -1.035533905932742416 ) ) ;
#1961=CARTESIAN_POINT ( 'NONE',  ( 91.91746824999998466, 112.6261737610028320, -51.22500000273119980 ) ) ;
#1963=ORIENTED_EDGE ( 'NONE', *, *, #22425, .T. ) ;
#1991=CARTESIAN_POINT ( 'NONE',  ( 102.4976396683250925, 102.3130555110000159, -44.77500000273119696 ) ) ;
#1995=FACE_OUTER_BOUND ( 'NONE', #27457, .T. ) ;
#1996=CARTESIAN_POINT ( 'NONE',  ( 95.54126587499999346, 92.74999999863439371, -1.846868145590737864 ) ) ;
#2003=CARTESIAN_POINT ( 'NONE',  ( 95.54126587499999346, 94.74999999863440792, -1.846868145590737864 ) ) ;
#2004=ORIENTED_EDGE ( 'NONE', *, *, #25146, .F. ) ;
#2013=ADVANCED_FACE ( 'NONE', ( #23687 ), #17400, .F. ) ;
#2016=CARTESIAN_POINT ( 'NONE',  ( 104.3262379212492590, 104.0454443415356991, -51.29999999999999716 ) ) ;
#2022=EDGE_CURVE ( 'NONE', #19200, #27429, #21550, .T. ) ;
#2024=CARTESIAN_POINT ( 'NONE',  ( 97.71650635000000307, 124.8750000005462368, -9.540979117872439019E-15 ) ) ;
#2027=CARTESIAN_POINT ( 'NONE',  ( 106.5389055433251002, 105.2492070361643215, -52.32500000273119412 ) ) ;
#2034=ORIENTED_EDGE ( 'NONE', *, *, #20288, .F. ) ;
#2038=CYLINDRICAL_SURFACE ( 'NONE', #23496, 7.000000000000006217 ) ;
#2046=CARTESIAN_POINT ( 'NONE',  ( 93.00000000000001421, 107.7255621263696668, -53.90000000000000568 ) ) ;
#2056=VERTEX_POINT ( 'NONE', #9275 ) ;
#2057=ORIENTED_EDGE ( 'NONE', *, *, #17510, .F. ) ;
#2064=LINE ( 'NONE', #4200, #25387 ) ;
#2083=CARTESIAN_POINT ( 'NONE',  ( 95.00472066334981491, 103.1245878333314465, -52.82500000273118701 ) ) ;
#2086=CARTESIAN_POINT ( 'NONE',  ( 97.50000000000000000, 122.6500000021849530, -1.035533905932742416 ) ) ;
#2090=ORIENTED_EDGE ( 'NONE', *, *, #5433, .T. ) ;
#2091=FACE_OUTER_BOUND ( 'NONE', #20465, .T. ) ;
#2098=CARTESIAN_POINT ( 'NONE',  ( 93.46109445667491400, 105.2492070361643215, -50.92500000273119554 ) ) ;
#2120=ORIENTED_EDGE ( 'NONE', *, *, #20253, .T. ) ;
#2131=CARTESIAN_POINT ( 'NONE',  ( 99.99999999999998579, 118.4984768113314146, -45.87500000273119127 ) ) ;
#2135=DIRECTION ( 'NONE',  ( 5.782411586589357392E-17, -0.000000000000000000, 1.000000000000000000 ) ) ;
#2136=CARTESIAN_POINT ( 'NONE',  ( 104.4587341249999923, 93.24999999863439371, 1.846868145590726318 ) ) ;
#2137=AXIS2_PLACEMENT_3D ( 'NONE', #22959, #12369, #3421 ) ;
#2145=CARTESIAN_POINT ( 'NONE',  ( 95.54126587499999346, 91.87499999863439371, 1.846868145590722543 ) ) ;
#2150=DIRECTION ( 'NONE',  ( 0.000000000000000000, 0.000000000000000000, 1.000000000000000000 ) ) ;
#2166=CARTESIAN_POINT ( 'NONE',  ( 93.00000000000000000, 112.2744378736303190, -46.10000000000000142 ) ) ;
#2169=CARTESIAN_POINT ( 'NONE',  ( 93.46109445667491400, 105.2492070361643215, -50.92500000273119554 ) ) ;
#2177=FACE_OUTER_BOUND ( 'NONE', #4881, .T. ) ;
#2178=CARTESIAN_POINT ( 'NONE',  ( 101.4615807364564546, 123.4500000010924765, -1.461580736456474794 ) ) ;
#2189=CARTESIAN_POINT ( 'NONE',  ( 95.67376207875072680, 115.9545556584642867, -52.30000000000001137 ) ) ;
#2191=CARTESIAN_POINT ( 'NONE',  ( 97.93301270000000613, 123.9500000010924765, -9.540979117872439019E-15 ) ) ;
#2192=EDGE_CURVE ( 'NONE', #923, #14907, #3043, .T. ) ;
#2195=CARTESIAN_POINT ( 'NONE',  ( 103.5355339059327235, 92.74999999726881583, 3.535533905932724874 ) ) ;
#2221=EDGE_CURVE ( 'NONE', #7002, #12839, #26826, .T. ) ;
#2223=CARTESIAN_POINT ( 'NONE',  ( 97.83688103937537051, 103.3426043859339103, -46.10000000546238397 ) ) ;
#2228=CARTESIAN_POINT ( 'NONE',  ( 102.4976396683250925, 117.6869444889999841, -53.72500000273119980 ) ) ;
#2235=AXIS2_PLACEMENT_3D ( 'NONE', #6523, #264, #15201 ) ;
#2238=CARTESIAN_POINT ( 'NONE',  ( 98.53841926354351699, 122.8500000010924680, -1.461580736456474794 ) ) ;
#2245=CARTESIAN_POINT ( 'NONE',  ( 97.50236033167492167, 117.6869444889999841, -51.52500000273119696 ) ) ;
#2246=CARTESIAN_POINT ( 'NONE',  ( 108.0825317500000153, 110.0000000000000000, -44.37500000273119838 ) ) ;
#2249=CARTESIAN_POINT ( 'NONE',  ( 104.7293670624999748, 95.71874999795160477, -6.938893903907228378E-15 ) ) ;
#2259=VERTEX_POINT ( 'NONE', #9559 ) ;
#2269=CARTESIAN_POINT ( 'NONE',  ( 98.23223304703363112, 122.8000000021849587, 1.767766952966351557 ) ) ;
#2270=CARTESIAN_POINT ( 'NONE',  ( 99.99999999999998579, 123.6000000000000085, 2.499999999999978684 ) ) ;
#2277=DIRECTION ( 'NONE',  ( 0.000000000000000000, 0.000000000000000000, -1.000000000000000000 ) ) ;
#2281=CARTESIAN_POINT ( 'NONE',  ( 93.00000000000001421, 112.2744378736303332, -44.60000000546238397 ) ) ;
#2282=CARTESIAN_POINT ( 'NONE',  ( 95.54126587499999346, 91.87499999863439371, 1.846868145590722543 ) ) ;
#2287=VERTEX_POINT ( 'NONE', #24953 ) ;
#2290=CARTESIAN_POINT ( 'NONE',  ( 96.84719886470463734, 93.68749999863440792, -3.152801135295366208 ) ) ;
#2308=EDGE_CURVE ( 'NONE', #6173, #370, #16868, .T. ) ;
#2313=CARTESIAN_POINT ( 'NONE',  ( 84.99999999999998579, 125.0000000000000000, 14.99999999999999112 ) ) ;
#2331=CARTESIAN_POINT ( 'NONE',  ( 105.6631189606246295, 114.1144967660473242, -48.80000000000001137 ) ) ;
#2336=CARTESIAN_POINT ( 'NONE',  ( 103.5355339059327235, 95.74999999726881583, 3.535533905932724874 ) ) ;
#2338=EDGE_CURVE ( 'NONE', #27581, #18466, #22719, .T. ) ;
#2379=CARTESIAN_POINT ( 'NONE',  ( 97.93301269999999192, 123.8000000010924850, 0.8561741729129329626 ) ) ;
#2384=CARTESIAN_POINT ( 'NONE',  ( 108.0825317500000153, 110.0000000000000000, -54.25000000273119838 ) ) ;
#2387=CARTESIAN_POINT ( 'NONE',  ( 97.50236033167492167, 102.3130555110000159, -48.72500000273119269 ) ) ;
#2406=CARTESIAN_POINT ( 'NONE',  ( 99.99999999999998579, 90.00000000000000000, -6.938893903907228378E-15 ) ) ;
#2407=CIRCLE ( 'NONE', #6944, 2.499999999999995115 ) ;
#2408=CARTESIAN_POINT ( 'NONE',  ( 103.5355339059327235, 93.12500000000000000, -3.535533905932738197 ) ) ;
#2410=VERTEX_POINT ( 'NONE', #24605 ) ;
#2418=EDGE_CURVE ( 'NONE', #13118, #24171, #10114, .T. ) ;
#2419=CARTESIAN_POINT ( 'NONE',  ( 99.99999999999998579, 101.5015231886685712, -44.87500000273119838 ) ) ;
#2423=CARTESIAN_POINT ( 'NONE',  ( 97.64864547061532107, 122.9999999999999858, 0.8612512827582227137 ) ) ;
#2430=CARTESIAN_POINT ( 'NONE',  ( 99.99999999999998579, 94.06249999863440792, 4.458734124999981674 ) ) ;
#2452=CARTESIAN_POINT ( 'NONE',  ( 108.0825317500000011, 112.6261737610028320, -54.02500000273118275 ) ) ;
#2453=CARTESIAN_POINT ( 'NONE',  ( 99.99999999999998579, 124.0000000000000000, -2.499999999999997780 ) ) ;
#2458=CARTESIAN_POINT ( 'NONE',  ( 104.3262379212492590, 115.9545556584642867, -51.20000000546237118 ) ) ;
#2468=CARTESIAN_POINT ( 'NONE',  ( 94.33688103937537051, 114.1144967660473242, -52.20000000000000995 ) ) ;
#2470=CARTESIAN_POINT ( 'NONE',  ( 101.0355339059327378, 124.4500000000000028, 2.499999999999977796 ) ) ;
#2473=CARTESIAN_POINT ( 'NONE',  ( 95.00000000000000000, 94.31249999726880162, -2.071067811865479058 ) ) ;
#2477=CARTESIAN_POINT ( 'NONE',  ( 102.4999999999999858, 123.1500000021849672, -1.035533905932742638 ) ) ;
#2487=PLANE ( 'NONE',  #359 ) ;
#2495=ORIENTED_EDGE ( 'NONE', *, *, #12780, .F. ) ;
#2500=EDGE_LOOP ( 'NONE', ( #23716, #19526, #11070, #26522 ) ) ;
#2501=CARTESIAN_POINT ( 'NONE',  ( 87.00000000000000000, 118.0000000000000000, -13.00000000000000711 ) ) ;
#2504=CARTESIAN_POINT ( 'NONE',  ( 99.99999999999998579, 124.7999999999999972, -2.499999999999997780 ) ) ;
#2505=CARTESIAN_POINT ( 'NONE',  ( 91.91746824999998466, 107.3738262389971680, -53.02500000273119696 ) ) ;
#2507=CARTESIAN_POINT ( 'NONE',  ( 102.4999999999999716, 122.3500000021849701, -1.035533905932742638 ) ) ;
#2513=CARTESIAN_POINT ( 'NONE',  ( 98.53841926354351699, 123.6500000010924794, -1.461580736456474794 ) ) ;
#2521=CARTESIAN_POINT ( 'NONE',  ( 108.0825317500000011, 107.3738262389971538, -44.47500000273118559 ) ) ;
#2534=ADVANCED_FACE ( 'NONE', ( #10595 ), #21164, .F. ) ;
#2543=CARTESIAN_POINT ( 'NONE',  ( 99.99999999999998579, 123.7000000021849502, 2.499999999999978684 ) ) ;
#2546=VECTOR ( 'NONE', #16546, 1000.000000000000000 ) ;
#2547=EDGE_CURVE ( 'NONE', #7547, #15121, #21253, .T. ) ;
#2549=DIRECTION ( 'NONE',  ( -1.000000000000000000, 0.000000000000000000, 0.000000000000000000 ) ) ;
#2557=CARTESIAN_POINT ( 'NONE',  ( 91.91746824999998466, 107.3738262389971680, -47.27500000273118985 ) ) ;
#2558=CARTESIAN_POINT ( 'NONE',  ( 107.0000000000000142, 110.0000000000000000, -45.50000000546238255 ) ) ;
#2561=CARTESIAN_POINT ( 'NONE',  ( 97.80124048048590168, 123.0000000000000142, -1.224358067407148587 ) ) ;
#2562=LINE ( 'NONE', #15654, #15728 ) ;
#2571=CARTESIAN_POINT ( 'NONE',  ( 101.8468681455907330, 94.49999999863442213, -4.458734124999994997 ) ) ;
#2576=ORIENTED_EDGE ( 'NONE', *, *, #6335, .F. ) ;
#2579=ADVANCED_FACE ( 'NONE', ( #27726 ), #25713, .F. ) ;
#2584=VECTOR ( 'NONE', #16967, 1000.000000000000000 ) ;
#2592=CARTESIAN_POINT ( 'NONE',  ( 104.9999999999999858, 92.00000000000000000, -6.938893903907228378E-15 ) ) ;
#2596=CARTESIAN_POINT ( 'NONE',  ( 108.0825317500000011, 107.3738262389971538, -46.22500000273118559 ) ) ;
#2597=CARTESIAN_POINT ( 'NONE',  ( 99.99999999999998579, 123.6000000000000085, 2.499999999999978684 ) ) ;
#2603=DIRECTION ( 'NONE',  ( -0.000000000000000000, 1.000000000000000000, -0.000000000000000000 ) ) ;
#2604=CARTESIAN_POINT ( 'NONE',  ( 99.99999999999998579, 122.7500000010924879, -2.066987299999998751 ) ) ;
#2610=ORIENTED_EDGE ( 'NONE', *, *, #10957, .F. ) ;
#2611=CARTESIAN_POINT ( 'NONE',  ( 93.00000000000001421, 112.2744378736303332, -46.10000000000000142 ) ) ;
#2613=CARTESIAN_POINT ( 'NONE',  ( 101.7677669529663547, 123.8999999999999915, -1.767766952966370209 ) ) ;
#2617=CARTESIAN_POINT ( 'NONE',  ( 96.46446609406726225, 93.24999999726881583, -3.535533905932738197 ) ) ;
#2623=ORIENTED_EDGE ( 'NONE', *, *, #44, .T. ) ;
#2629=DIRECTION ( 'NONE',  ( 0.000000000000000000, 1.000000000000000000, -1.156482317317871478E-16 ) ) ;
#2631=EDGE_LOOP ( 'NONE', ( #21780, #2090, #21677 ) ) ;
#2633=CARTESIAN_POINT ( 'NONE',  ( 104.4587341249999923, 91.49999999863440792, 1.846868145590726318 ) ) ;
#2639=EDGE_LOOP ( 'NONE', ( #2576, #13038, #22128 ) ) ;
#2648=CARTESIAN_POINT ( 'NONE',  ( 97.50236033167492167, 102.3130555110000159, -52.72500000273119980 ) ) ;
#2654=EDGE_LOOP ( 'NONE', ( #25934, #10017, #11980, #12718 ) ) ;
#2657=CARTESIAN_POINT ( 'NONE',  ( 101.4615807364564546, 124.2500000010924879, -1.461580736456474794 ) ) ;
#2660=VECTOR ( 'NONE', #560, 1000.000000000000000 ) ;
#2665=CARTESIAN_POINT ( 'NONE',  ( 102.4976396683250925, 117.6869444889999841, -45.72500000273119269 ) ) ;
#2671=ORIENTED_EDGE ( 'NONE', *, *, #23773, .T. ) ;
#2672=ORIENTED_EDGE ( 'NONE', *, *, #14123, .F. ) ;
#2684=FACE_OUTER_BOUND ( 'NONE', #18957, .T. ) ;
#2685=AXIS2_PLACEMENT_3D ( 'NONE', #17965, #26674, #7121 ) ;
#2702=EDGE_CURVE ( 'NONE', #4367, #24513, #21664, .T. ) ;
#2710=CARTESIAN_POINT ( 'NONE',  ( 94.33688103937537051, 114.1144967660473242, -50.20000000000000995 ) ) ;
#2713=CARTESIAN_POINT ( 'NONE',  ( 96.46446609406726225, 92.37500000000000000, -3.535533905932738197 ) ) ;
#2720=CARTESIAN_POINT ( 'NONE',  ( 95.00000000000000000, 95.31249999726880162, -2.071067811865479058 ) ) ;
#2722=ORIENTED_EDGE ( 'NONE', *, *, #23773, .F. ) ;
#2735=CARTESIAN_POINT ( 'NONE',  ( 97.83688103937538472, 116.6573956140660897, -52.90000000546237402 ) ) ;
#2741=CIRCLE ( 'NONE', #3651, 9.000000000000007105 ) ;
#2753=CARTESIAN_POINT ( 'NONE',  ( 108.0825317500000153, 110.0000000000000000, -54.37500000273119838 ) ) ;
#2755=CARTESIAN_POINT ( 'NONE',  ( 102.4999999999999716, 123.8500000000000085, -1.035533905932742638 ) ) ;
#2757=CARTESIAN_POINT ( 'NONE',  ( 107.0000000000000142, 110.0000000000000000, -43.50000000546237544 ) ) ;
#2760=CARTESIAN_POINT ( 'NONE',  ( 99.99999999999998579, 93.62499999726881583, 4.999999999999984013 ) ) ;
#2763=CARTESIAN_POINT ( 'NONE',  ( 108.0825317500000011, 112.6261737610028320, -54.27500000273118985 ) ) ;
#2788=CARTESIAN_POINT ( 'NONE',  ( 91.91746824999998466, 107.3738262389971680, -49.02500000273119696 ) ) ;
#2794=CARTESIAN_POINT ( 'NONE',  ( 101.4615807364564546, 122.6500000010924794, -1.461580736456474794 ) ) ;
#2798=CARTESIAN_POINT ( 'NONE',  ( 103.5355338419364699, 95.00000000000001421, -3.535533969929001596 ) ) ;
#2800=CARTESIAN_POINT ( 'NONE',  ( 101.8468681455907330, 94.12499999863439371, 4.458734124999979898 ) ) ;
#2807=ORIENTED_EDGE ( 'NONE', *, *, #10525, .T. ) ;
#2823=( NAMED_UNIT ( * ) SI_UNIT ( $, .STERADIAN. ) SOLID_ANGLE_UNIT ( ) );
#2837=FACE_BOUND ( 'NONE', #27498, .T. ) ;
#2838=CARTESIAN_POINT ( 'NONE',  ( 102.3057342235964882, 122.9999999999999858, -0.9766400096817489107 ) ) ;
#2839=CARTESIAN_POINT ( 'NONE',  ( 101.4615807364564546, 124.2500000010924879, -1.461580736456474794 ) ) ;
#2846=CARTESIAN_POINT ( 'NONE',  ( 103.5355339059327235, 91.12500000000000000, -3.535533905932738197 ) ) ;
#2850=EDGE_LOOP ( 'NONE', ( #21299, #23566, #9122, #16662 ) ) ;
#2860=CARTESIAN_POINT ( 'NONE',  ( 107.5412658750000077, 110.0000000000000000, -43.81250000409678336 ) ) ;
#2863=CARTESIAN_POINT ( 'NONE',  ( 96.84719886470463734, 90.93749999863440792, 3.152801135295351997 ) ) ;
#2864=DIRECTION ( 'NONE',  ( -0.000000000000000000, 1.000000000000000000, -0.000000000000000000 ) ) ;
#2868=CARTESIAN_POINT ( 'NONE',  ( 107.0000000000000142, 112.2744378736303332, -53.40000000546237402 ) ) ;
#2871=CARTESIAN_POINT ( 'NONE',  ( 107.0000000000000142, 110.0000000000000000, -49.50000000546238255 ) ) ;
#2875=CARTESIAN_POINT ( 'NONE',  ( 99.99999999999998579, 95.12499999726881583, -4.999999999999997335 ) ) ;
#2884=CARTESIAN_POINT ( 'NONE',  ( 108.0825317500000011, 112.6261737610028320, -52.27500000273118985 ) ) ;
#2886=CARTESIAN_POINT ( 'NONE',  ( 99.99999999999998579, 124.7999999999999972, -2.499999999999997780 ) ) ;
#2893=CARTESIAN_POINT ( 'NONE',  ( 104.4587341249999923, 93.49999999863442213, 1.846868145590726318 ) ) ;
#2895=CARTESIAN_POINT ( 'NONE',  ( 97.50236033167492167, 117.6869444889999841, -53.77500000273119696 ) ) ;
#2903=DIRECTION ( 'NONE',  ( -5.782411586589357392E-17, -1.156482317317871478E-16, -1.000000000000000000 ) ) ;
#2907=CARTESIAN_POINT ( 'NONE',  ( 101.8468681455907330, 91.37499999863442213, 4.458734124999980786 ) ) ;
#2910=VERTEX_POINT ( 'NONE', #3855 ) ;
#2921=EDGE_CURVE ( 'NONE', #20854, #7547, #13184, .T. ) ;
#2923=CARTESIAN_POINT ( 'NONE',  ( 108.0825317500000153, 110.0000000000000000, -46.12500000273119838 ) ) ;
#2935=CARTESIAN_POINT ( 'NONE',  ( 102.4976396683250925, 102.3130555110000159, -44.52500000273119696 ) ) ;
#2938=DIRECTION ( 'NONE',  ( 0.000000000000000000, -1.000000000000000000, 0.000000000000000000 ) ) ;
#2940=CARTESIAN_POINT ( 'NONE',  ( 97.92893218813452449, 91.18749999726880162, -4.999999999999997335 ) ) ;
#2957=CARTESIAN_POINT ( 'NONE',  ( 101.0355339059327378, 124.7569999999781629, -2.499999999999997780 ) ) ;
#2972=PLANE ( 'NONE',  #9401 ) ;
#2980=AXIS2_PLACEMENT_3D ( 'NONE', #8296, #4034, #16985 ) ;
#2981=CARTESIAN_POINT ( 'NONE',  ( 96.46446609406726225, 94.62500000000000000, 3.535533905932723986 ) ) ;
#2984=CARTESIAN_POINT ( 'NONE',  ( 96.46446609406726225, 90.62500000000000000, 3.535533905932723986 ) ) ;
#2985=DIRECTION ( 'NONE',  ( 0.000000000000000000, 4.625929269271485914E-16, 1.000000000000000000 ) ) ;
#2994=ORIENTED_EDGE ( 'NONE', *, *, #17554, .F. ) ;
#3011=CARTESIAN_POINT ( 'NONE',  ( 97.50236033167492167, 102.3130555110000159, -46.72500000273119269 ) ) ;
#3012=CARTESIAN_POINT ( 'NONE',  ( 100.0000000000000000, 110.0000000000000000, -55.00000000000000711 ) ) ;
#3017=ORIENTED_EDGE ( 'NONE', *, *, #12292, .T. ) ;
#3020=CARTESIAN_POINT ( 'NONE',  ( 98.23223304703363112, 123.4000000021849530, -1.767766952966370209 ) ) ;
#3023=AXIS2_PLACEMENT_3D ( 'NONE', #19045, #7939, #21194 ) ;
#3027=CARTESIAN_POINT ( 'NONE',  ( 95.00472066334982912, 116.8754121666685393, -53.67500000273118843 ) ) ;
#3030=CARTESIAN_POINT ( 'NONE',  ( 99.99999999999998579, 123.2000000000000028, -2.499999999999997780 ) ) ;
#3036=CARTESIAN_POINT ( 'NONE',  ( 96.84719886470463734, 92.18749999863440792, 3.152801135295351997 ) ) ;
#3038=CARTESIAN_POINT ( 'NONE',  ( 102.4976396683250925, 102.3130555110000159, -50.77500000273119696 ) ) ;
#3043=CIRCLE ( 'NONE', #20812, 4.999999999999989342 ) ;
#3046=CARTESIAN_POINT ( 'NONE',  ( 101.7677669529663547, 124.5000000000000000, 1.767766952966350891 ) ) ;
#3059=ORIENTED_EDGE ( 'NONE', *, *, #11234, .F. ) ;
#3062=ORIENTED_EDGE ( 'NONE', *, *, #25549, .T. ) ;
#3065=EDGE_LOOP ( 'NONE', ( #7385, #8947, #22450, #3017 ) ) ;
#3070=CARTESIAN_POINT ( 'NONE',  ( 91.91746824999998466, 112.6261737610028320, -49.22500000273119269 ) ) ;
#3104=CARTESIAN_POINT ( 'NONE',  ( 93.00000000000002842, 112.2744378736303474, -48.10000000000000142 ) ) ;
#3126=CARTESIAN_POINT ( 'NONE',  ( 101.5628473693180069, 123.0000000000000000, 1.972588198814292593 ) ) ;
#3134=CARTESIAN_POINT ( 'NONE',  ( 99.99999999999998579, 94.25000000000000000, -4.999999999999997335 ) ) ;
#3136=VECTOR ( 'NONE', #19620, 999.9999999999998863 ) ;
#3145=ORIENTED_EDGE ( 'NONE', *, *, #25061, .T. ) ;
#3152=CARTESIAN_POINT ( 'NONE',  ( 104.4587341249999923, 92.24999999863439371, 1.846868145590726318 ) ) ;
#3158=CARTESIAN_POINT ( 'NONE',  ( 102.4976396683250925, 102.3130555110000159, -48.52500000273119696 ) ) ;
#3159=CARTESIAN_POINT ( 'NONE',  ( 104.4587341249999781, 90.56249999863440792, -6.938893903907228378E-15 ) ) ;
#3165=CARTESIAN_POINT ( 'NONE',  ( 98.23223304703363112, 123.6000000021849416, 1.767766952966351557 ) ) ;
#3167=ORIENTED_EDGE ( 'NONE', *, *, #13236, .F. ) ;
#3172=CARTESIAN_POINT ( 'NONE',  ( 99.99999999999998579, 101.5015231886685854, -46.87500000273119838 ) ) ;
#3175=CARTESIAN_POINT ( 'NONE',  ( 99.99999999999998579, 90.00000000000000000, -6.938893903907228378E-15 ) ) ;
#3181=CARTESIAN_POINT ( 'NONE',  ( 104.4587341249999781, 91.56249999863440792, -6.938893903907228378E-15 ) ) ;
#3182=PLANE ( 'NONE',  #8234 ) ;
#3183=CARTESIAN_POINT ( 'NONE',  ( 91.91746824999998466, 107.3738262389971680, -51.27500000273119696 ) ) ;
#3184=DIRECTION ( 'NONE',  ( 0.000000000000000000, -1.000000000000000000, -0.000000000000000000 ) ) ;
#3192=CARTESIAN_POINT ( 'NONE',  ( 95.54126587499999346, 90.99999999863439371, -1.846868145590737864 ) ) ;
#3201=CARTESIAN_POINT ( 'NONE',  ( 102.0669873000000081, 122.8000000010924708, -0.8561741729129508371 ) ) ;
#3205=CARTESIAN_POINT ( 'NONE',  ( 96.46446609406726225, 91.49999999726880162, 3.535533905932723986 ) ) ;
#3207=ADVANCED_FACE ( 'NONE', ( #323 ), #17413, .F. ) ;
#3213=ORIENTED_EDGE ( 'NONE', *, *, #2418, .T. ) ;
#3220=ADVANCED_FACE ( 'NONE', ( #28116 ), #21564, .F. ) ;
#3221=CARTESIAN_POINT ( 'NONE',  ( 104.9999999999999858, 94.87499999726881583, -6.938893903907228378E-15 ) ) ;
#3223=CARTESIAN_POINT ( 'NONE',  ( 99.99999999999998579, 92.12499999726880162, -4.999999999999997335 ) ) ;
#3224=CARTESIAN_POINT ( 'NONE',  ( 91.91746824999998466, 112.6261737610028320, -45.22500000273119980 ) ) ;
#3225=CARTESIAN_POINT ( 'NONE',  ( 99.99999999999998579, 123.2000000000000028, -2.499999999999997780 ) ) ;
#3239=CARTESIAN_POINT ( 'NONE',  ( 102.0669872999999797, 122.7500000010924737, -9.794112055954760458E-15 ) ) ;
#3242=ADVANCED_FACE ( 'NONE', ( #15548 ), #6718, .F. ) ;
#3244=CARTESIAN_POINT ( 'NONE',  ( 94.33688103937537051, 114.1144967660473242, -48.20000000000000995 ) ) ;
#3246=VECTOR ( 'NONE', #5356, 1000.000000000000000 ) ;
#3252=FILL_AREA_STYLE ('',( #15779 ) ) ;
#3254=CARTESIAN_POINT ( 'NONE',  ( 97.83688103937537051, 103.3426043859339103, -47.60000000000000142 ) ) ;
#3272=CARTESIAN_POINT ( 'NONE',  ( 107.0000000000000142, 110.0000000000000000, -51.00000000000000711 ) ) ;
#3275=CARTESIAN_POINT ( 'NONE',  ( 96.46446609406726225, 91.37500000000000000, -3.535533905932738197 ) ) ;
#3276=CARTESIAN_POINT ( 'NONE',  ( 87.00000000000000000, 102.0000000000000142, -15.00000000000000711 ) ) ;
#3280=VERTEX_POINT ( 'NONE', #10981 ) ;
#3297=CARTESIAN_POINT ( 'NONE',  ( 102.1631189606246295, 116.6573956140660897, -53.10000000546238397 ) ) ;
#3299=CARTESIAN_POINT ( 'NONE',  ( 104.3262379212492590, 104.0454443415356991, -47.80000000546237970 ) ) ;
#3300=CARTESIAN_POINT ( 'NONE',  ( 95.54126587499999346, 92.12499999863437949, 1.846868145590722543 ) ) ;
#3312=ORIENTED_EDGE ( 'NONE', *, *, #1027, .T. ) ;
#3313=CARTESIAN_POINT ( 'NONE',  ( 104.9952793366501851, 103.1245878333314323, -44.67500000273118843 ) ) ;
#3316=DIRECTION ( 'NONE',  ( 5.782411586589357392E-17, -0.000000000000000000, 1.000000000000000000 ) ) ;
#3320=CARTESIAN_POINT ( 'NONE',  ( 99.99999999999998579, 93.81249999863440792, -4.458734124999994997 ) ) ;
#3333=CARTESIAN_POINT ( 'NONE',  ( 99.99999999999998579, 93.31249999863440792, 4.458734124999981674 ) ) ;
#3336=CYLINDRICAL_SURFACE ( 'NONE', #25938, 9.000000000000007105 ) ;
#3338=DIRECTION ( 'NONE',  ( -0.000000000000000000, 1.000000000000000000, -0.000000000000000000 ) ) ;
#3349=CARTESIAN_POINT ( 'NONE',  ( 99.99999999999998579, 90.25000000000000000, -4.999999999999997335 ) ) ;
#3361=DIRECTION ( 'NONE',  ( 0.000000000000000000, 0.000000000000000000, 1.000000000000000000 ) ) ;
#3363=ORIENTED_EDGE ( 'NONE', *, *, #15545, .T. ) ;
#3375=CARTESIAN_POINT ( 'NONE',  ( 99.99999999999998579, 117.3602355696678643, -48.49999999999999289 ) ) ;
#3380=CARTESIAN_POINT ( 'NONE',  ( 101.7677669529663547, 123.0999999999999943, -1.767766952966370209 ) ) ;
#3399=EDGE_CURVE ( 'NONE', #8723, #14157, #38, .T. ) ;
#3400=CARTESIAN_POINT ( 'NONE',  ( 100.8561741729129153, 123.5000000010924737, -2.066987299999999195 ) ) ;
#3410=EDGE_CURVE ( 'NONE', #2056, #3788, #24873, .T. ) ;
#3411=AXIS2_PLACEMENT_3D ( 'NONE', #10151, #18732, #5632 ) ;
#3421=DIRECTION ( 'NONE',  ( 0.000000000000000000, 0.000000000000000000, 1.000000000000000000 ) ) ;
#3426=CARTESIAN_POINT ( 'NONE',  ( 99.99999999999998579, 91.06249999863440792, 4.458734124999981674 ) ) ;
#3432=CARTESIAN_POINT ( 'NONE',  ( 93.00000000000000000, 112.2744378736303190, -52.60000000546237686 ) ) ;
#3433=VECTOR ( 'NONE', #27349, 1000.000000000000000 ) ;
#3435=CARTESIAN_POINT ( 'NONE',  ( 94.33688103937537051, 105.8855032339526758, -50.30000000546237970 ) ) ;
#3436=CARTESIAN_POINT ( 'NONE',  ( 104.4587341249999923, 91.37499999863439371, -1.846868145590737198 ) ) ;
#3440=EDGE_CURVE ( 'NONE', #5694, #9247, #27121, .T. ) ;
#3441=EDGE_LOOP ( 'NONE', ( #21249, #25162, #12942, #26071 ) ) ;
#3445=CARTESIAN_POINT ( 'NONE',  ( 96.46446609406726225, 91.37500000000000000, -3.535533905932738197 ) ) ;
#3452=CARTESIAN_POINT ( 'NONE',  ( 104.9952793366501851, 103.1245878333314323, -48.67500000273119554 ) ) ;
#3459=CARTESIAN_POINT ( 'NONE',  ( 95.54126587499999346, 92.99999999863439371, -1.846868145590737864 ) ) ;
#3469=ORIENTED_EDGE ( 'NONE', *, *, #802, .F. ) ;
#3473=CARTESIAN_POINT ( 'NONE',  ( 104.9999999999999858, 90.87499999726880162, -6.938893903907228378E-15 ) ) ;
#3475=EDGE_CURVE ( 'NONE', #24171, #14907, #20413, .T. ) ;
#3477=CARTESIAN_POINT ( 'NONE',  ( 100.0000000000000000, 110.0000000000000000, -55.00000000000000711 ) ) ;
#3481=EDGE_LOOP ( 'NONE', ( #8727, #14805 ) ) ;
#3484=EDGE_LOOP ( 'NONE', ( #27907, #10636, #20606, #21114 ) ) ;
#3485=CARTESIAN_POINT ( 'NONE',  ( 95.00000000000000000, 92.43750000000000000, -2.071067811865479058 ) ) ;
#3486=DIRECTION ( 'NONE',  ( 0.000000000000000000, 1.000000000000000000, 0.000000000000000000 ) ) ;
#3495=ORIENTED_EDGE ( 'NONE', *, *, #4985, .T. ) ;
#3531=CARTESIAN_POINT ( 'NONE',  ( 101.7677669529663547, 123.1069999999781572, -1.767766952966370209 ) ) ;
#3543=CARTESIAN_POINT ( 'NONE',  ( 84.99999999999998579, 100.0000000000000000, -13.00000000000000533 ) ) ;
#3546=CARTESIAN_POINT ( 'NONE',  ( 106.5389055433251002, 105.2492070361643215, -50.57500000273120122 ) ) ;
#3547=FACE_OUTER_BOUND ( 'NONE', #8301, .T. ) ;
#3548=CARTESIAN_POINT ( 'NONE',  ( 101.4615807364564546, 123.6500000010924651, -1.461580736456474794 ) ) ;
#3554=FACE_OUTER_BOUND ( 'NONE', #2631, .T. ) ;
#3572=CARTESIAN_POINT ( 'NONE',  ( 104.4587341249999923, 93.37499999863440792, -1.846868145590737198 ) ) ;
#3573=( BOUNDED_CURVE ( )  B_SPLINE_CURVE ( 2, ( #15155, #8905, #17593 ),
 .UNSPECIFIED., .F., .T. ) 
 B_SPLINE_CURVE_WITH_KNOTS ( ( 3, 3 ),
 ( 0.8250000005912483392, 0.8500000000000007550 ),
 .UNSPECIFIED. ) 
 CURVE ( )  GEOMETRIC_REPRESENTATION_ITEM ( )  RATIONAL_B_SPLINE_CURVE ( ( 1.000000000000000000, 0.9238795325112844070, 1.000000000000002442 ) ) 
 REPRESENTATION_ITEM ( '' )  );
#3580=CARTESIAN_POINT ( 'NONE',  ( 93.00000000000001421, 107.7255621263696668, -46.40000000546238113 ) ) ;
#3581=CARTESIAN_POINT ( 'NONE',  ( 104.4587341249999781, 95.56249999863440792, -6.938893903907228378E-15 ) ) ;
#3585=AXIS2_PLACEMENT_3D ( 'NONE', #2384, #11042, #25894 ) ;
#3587=ORIENTED_EDGE ( 'NONE', *, *, #2192, .F. ) ;
#3597=CARTESIAN_POINT ( 'NONE',  ( 95.00472066334982912, 103.1245878333314323, -45.07500000273119412 ) ) ;
#3601=CARTESIAN_POINT ( 'NONE',  ( 93.46109445667491400, 105.2492070361643215, -44.92500000273119554 ) ) ;
#3615=VERTEX_POINT ( 'NONE', #14259 ) ;
#3617=CARTESIAN_POINT ( 'NONE',  ( 98.53841926354351699, 123.8500000010924680, 1.461580736456455920 ) ) ;
#3618=CARTESIAN_POINT ( 'NONE',  ( 95.54126587499999346, 92.99999999863439371, -1.846868145590737864 ) ) ;
#3621=LINE ( 'NONE', #1765, #27610 ) ;
#3629=CARTESIAN_POINT ( 'NONE',  ( 99.99999999999998579, 92.25000000000000000, -4.999999999999997335 ) ) ;
#3635=ADVANCED_FACE ( 'NONE', ( #9422 ), #27120, .F. ) ;
#3651=AXIS2_PLACEMENT_3D ( 'NONE', #1444, #7844, #18682 ) ;
#3673=CARTESIAN_POINT ( 'NONE',  ( 97.50000000000000000, 124.9500000000000028, -1.035533905932742416 ) ) ;
#3685=CARTESIAN_POINT ( 'NONE',  ( 91.91746824999999887, 110.0000000000000000, -47.37500000273119838 ) ) ;
#3687=CARTESIAN_POINT ( 'NONE',  ( 98.53841926354351699, 123.2500000010924737, 1.461580736456455920 ) ) ;
#3691=ORIENTED_EDGE ( 'NONE', *, *, #8997, .F. ) ;
#3693=EDGE_CURVE ( 'NONE', #4535, #20388, #22882, .T. ) ;
#3698=AXIS2_PLACEMENT_3D ( 'NONE', #7625, #16317, #4471 ) ;
#3703=CARTESIAN_POINT ( 'NONE',  ( 99.99999999999998579, 117.3602355696678643, -52.50000000000000000 ) ) ;
#3711=CARTESIAN_POINT ( 'NONE',  ( 95.54126587499999346, 93.87499999863439371, 1.846868145590722543 ) ) ;
#3712=CARTESIAN_POINT ( 'NONE',  ( 106.5389055433251002, 105.2492070361643215, -52.57500000273119412 ) ) ;
#3720=CARTESIAN_POINT ( 'NONE',  ( 94.33688103937537051, 114.1144967660473242, -48.70000000546237828 ) ) ;
#3721=CARTESIAN_POINT ( 'NONE',  ( 95.54126587499999346, 92.99999999863439371, -1.846868145590737864 ) ) ;
#3727=CARTESIAN_POINT ( 'NONE',  ( 101.8468681455907330, 91.49999999863440792, -4.458734124999994997 ) ) ;
#3730=ORIENTED_EDGE ( 'NONE', *, *, #288, .F. ) ;
#3731=CARTESIAN_POINT ( 'NONE',  ( 99.99999999999998579, 90.00000000000000000, -6.938893903907228378E-15 ) ) ;
#3734=CARTESIAN_POINT ( 'NONE',  ( 106.5389055433251002, 105.2492070361643215, -48.57500000273119412 ) ) ;
#3736=FACE_OUTER_BOUND ( 'NONE', #14946, .T. ) ;
#3738=CARTESIAN_POINT ( 'NONE',  ( 91.91746824999998466, 107.3738262389971680, -47.02500000273118985 ) ) ;
#3743=CYLINDRICAL_SURFACE ( 'NONE', #4130, 4.999999999999989342 ) ;
#3755=CARTESIAN_POINT ( 'NONE',  ( 97.93301270000000613, 124.5000000010924879, -0.8561741729129506151 ) ) ;
#3767=ORIENTED_EDGE ( 'NONE', *, *, #27102, .T. ) ;
#3774=FACE_OUTER_BOUND ( 'NONE', #5831, .T. ) ;
#3779=CARTESIAN_POINT ( 'NONE',  ( 99.99999999999998579, 90.75000000000000000, 4.999999999999984013 ) ) ;
#3780=CARTESIAN_POINT ( 'NONE',  ( 102.1631189606246295, 103.3426043859339103, -51.90000000546238113 ) ) ;
#3782=DIRECTION ( 'NONE',  ( 0.000000000000000000, 0.000000000000000000, -1.000000000000000000 ) ) ;
#3788=VERTEX_POINT ( 'NONE', #9983 ) ;
#3798=DIRECTION ( 'NONE',  ( -0.000000000000000000, 1.000000000000000000, -0.000000000000000000 ) ) ;
#3803=CARTESIAN_POINT ( 'NONE',  ( 101.0355339059327378, 124.7500000000000142, -2.499999999999997780 ) ) ;
#3805=CARTESIAN_POINT ( 'NONE',  ( 98.53841926354351699, 124.0500000010924708, 1.461580736456455920 ) ) ;
#3810=VERTEX_POINT ( 'NONE', #1456 ) ;
#3811=CARTESIAN_POINT ( 'NONE',  ( 98.23223304703363112, 123.6000000021849416, 1.767766952966351557 ) ) ;
#3815=DIRECTION ( 'NONE',  ( -0.000000000000000000, 1.000000000000000000, -0.000000000000000000 ) ) ;
#3818=CARTESIAN_POINT ( 'NONE',  ( 91.91746824999998466, 107.3738262389971538, -49.27500000273118985 ) ) ;
#3820=CARTESIAN_POINT ( 'NONE',  ( 100.8561741729129153, 124.5000000010924737, -2.066987299999999195 ) ) ;
#3832=ORIENTED_EDGE ( 'NONE', *, *, #13926, .T. ) ;
#3834=CARTESIAN_POINT ( 'NONE',  ( 93.00000000000000000, 112.2744378736303190, -52.10000000000000142 ) ) ;
#3837=LINE ( 'NONE', #18674, #6926 ) ;
#3839=CARTESIAN_POINT ( 'NONE',  ( 102.4999999999999858, 122.3500000021849701, -1.035533905932742638 ) ) ;
#3843=DIRECTION ( 'NONE',  ( -0.000000000000000000, 1.000000000000000000, -0.000000000000000000 ) ) ;
#3851=CARTESIAN_POINT ( 'NONE',  ( 102.1631189606246295, 103.3426043859339103, -49.90000000546238113 ) ) ;
#3852=CARTESIAN_POINT ( 'NONE',  ( 99.99999999999998579, 93.81249999863440792, -4.458734124999994997 ) ) ;
#3853=CARTESIAN_POINT ( 'NONE',  ( 107.0000000000000142, 110.0000000000000000, -55.00000000000000711 ) ) ;
#3855=CARTESIAN_POINT ( 'NONE',  ( 99.99999999999998579, 124.1000000021849416, -2.499999999999997780 ) ) ;
#3858=VECTOR ( 'NONE', #3338, 1000.000000000000000 ) ;
#3859=CARTESIAN_POINT ( 'NONE',  ( 104.4587341249999923, 91.24999999863439371, 1.846868145590726318 ) ) ;
#3862=CARTESIAN_POINT ( 'NONE',  ( 99.99999999999998579, 94.62499999726881583, 4.999999999999984013 ) ) ;
#3863=VERTEX_POINT ( 'NONE', #12247 ) ;
#3866=ORIENTED_EDGE ( 'NONE', *, *, #18381, .F. ) ;
#3880=CARTESIAN_POINT ( 'NONE',  ( 99.99999999999998579, 117.3602355696678643, -46.50000000000000711 ) ) ;
#3891=CARTESIAN_POINT ( 'NONE',  ( 98.15313185440923860, 94.24999999863439371, 4.458734124999980786 ) ) ;
#3902=CARTESIAN_POINT ( 'NONE',  ( 97.92893218813449607, 92.31249999999997158, -4.999999999999971578 ) ) ;
#3905=CARTESIAN_POINT ( 'NONE',  ( 97.93301269999999192, 124.0000000010924879, 0.8561741729129329626 ) ) ;
#3908=ADVANCED_FACE ( 'NONE', ( #27396 ), #23953, .T. ) ;
#3926=DIRECTION ( 'NONE',  ( -0.000000000000000000, 1.000000000000000000, -0.000000000000000000 ) ) ;
#3939=CIRCLE ( 'NONE', #3023, 2.499999999999995115 ) ;
#3941=EDGE_CURVE ( 'NONE', #3615, #25660, #21527, .T. ) ;
#3946=CARTESIAN_POINT ( 'NONE',  ( 101.0355339059327378, 123.9500000000000028, -2.499999999999997780 ) ) ;
#3948=CARTESIAN_POINT ( 'NONE',  ( 102.0669873000000081, 123.5000000010924737, 0.8561741729129311862 ) ) ;
#3952=ORIENTED_EDGE ( 'NONE', *, *, #17696, .F. ) ;
#3961=CARTESIAN_POINT ( 'NONE',  ( 108.0825317500000011, 112.6261737610028320, -48.27500000273119696 ) ) ;
#3981=ADVANCED_FACE ( 'NONE', ( #8403 ), #25003, .F. ) ;
#3983=CARTESIAN_POINT ( 'NONE',  ( 101.7677669529663547, 122.4000000021849530, -1.767766952966370209 ) ) ;
#3995=CARTESIAN_POINT ( 'NONE',  ( 99.99999999999998579, 95.62499999726881583, 4.999999999999984013 ) ) ;
#3996=CARTESIAN_POINT ( 'NONE',  ( 96.84719886470463734, 93.18749999863440792, 3.152801135295351997 ) ) ;
#3999=CARTESIAN_POINT ( 'NONE',  ( 99.99999999999998579, 102.6397644303321215, -45.50000000000000000 ) ) ;
#4000=ORIENTED_EDGE ( 'NONE', *, *, #10677, .T. ) ;
#4009=VERTEX_POINT ( 'NONE', #3862 ) ;
#4021=AXIS2_PLACEMENT_3D ( 'NONE', #3543, #1411, #25063 ) ;
#4025=CARTESIAN_POINT ( 'NONE',  ( 106.5389055433251002, 114.7507929638356785, -51.92500000273119554 ) ) ;
#4032=ORIENTED_EDGE ( 'NONE', *, *, #3440, .F. ) ;
#4034=DIRECTION ( 'NONE',  ( 0.000000000000000000, 0.000000000000000000, 1.000000000000000000 ) ) ;
#4047=CARTESIAN_POINT ( 'NONE',  ( 93.00000000000001421, 107.7255621263696668, -51.89999999999999858 ) ) ;
#4050=CARTESIAN_POINT ( 'NONE',  ( 102.0710678118654755, 92.68749999726881583, 4.999999999999961808 ) ) ;
#4062=CARTESIAN_POINT ( 'NONE',  ( 99.99999999999998579, 90.00000000000000000, -6.938893903907228378E-15 ) ) ;
#4063=CARTESIAN_POINT ( 'NONE',  ( 99.99999999999998579, 89.99899999999999523, -9.540979117872439019E-15 ) ) ;
#4064=( GEOMETRIC_REPRESENTATION_CONTEXT ( 3 ) GLOBAL_UNCERTAINTY_ASSIGNED_CONTEXT ( ( #8332 ) ) GLOBAL_UNIT_ASSIGNED_CONTEXT ( ( #17603, #22887, #1232 ) ) REPRESENTATION_CONTEXT ( 'NONE', 'WORKASPACE' ) );
#4084=CARTESIAN_POINT ( 'NONE',  ( 98.23223304703363112, 123.4000000021849530, -1.767766952966370209 ) ) ;
#4088=CARTESIAN_POINT ( 'NONE',  ( 95.67376207875072680, 104.0454443415356991, -48.20000000546237118 ) ) ;
#4089=CARTESIAN_POINT ( 'NONE',  ( 97.50000000000000000, 123.5500000021849587, 1.035533905932725096 ) ) ;
#4098=CARTESIAN_POINT ( 'NONE',  ( 91.91746824999999887, 110.0000000000000000, -51.12500000273119127 ) ) ;
#4115=CARTESIAN_POINT ( 'NONE',  ( 105.6631189606246295, 114.1144967660473242, -47.30000000546237260 ) ) ;
#4120=CARTESIAN_POINT ( 'NONE',  ( 97.50000000000000000, 122.6500000021849530, -1.035533905932742416 ) ) ;
#4130=AXIS2_PLACEMENT_3D ( 'NONE', #7589, #9998, #9866 ) ;
#4133=CARTESIAN_POINT ( 'NONE',  ( 104.4587341249999923, 94.24999999863439371, 1.846868145590726318 ) ) ;
#4139=( GEOMETRIC_REPRESENTATION_CONTEXT ( 3 ) GLOBAL_UNCERTAINTY_ASSIGNED_CONTEXT ( ( #155 ) ) GLOBAL_UNIT_ASSIGNED_CONTEXT ( ( #20072, #13771, #2823 ) ) REPRESENTATION_CONTEXT ( 'NONE', 'WORKASPACE' ) );
#4140=CARTESIAN_POINT ( 'NONE',  ( 95.54126587500000767, 90.81249999863440792, -7.484931351350258973E-15 ) ) ;
#4156=CARTESIAN_POINT ( 'NONE',  ( 93.00000000000000000, 110.0000000000000000, -52.00000000000000711 ) ) ;
#4166=CARTESIAN_POINT ( 'NONE',  ( 99.99999999999998579, 118.4984768113314004, -53.62500000273119127 ) ) ;
#4167=CARTESIAN_POINT ( 'NONE',  ( 87.00000000000000000, 123.0000000000000000, -13.00000000000000888 ) ) ;
#4172=VERTEX_POINT ( 'NONE', #8235 ) ;
#4177=EDGE_LOOP ( 'NONE', ( #21455, #8984, #5874, #7678 ) ) ;
#4180=CARTESIAN_POINT ( 'NONE',  ( 84.99999999999998579, 120.0000000000000000, -45.00000000000000711 ) ) ;
#4182=CARTESIAN_POINT ( 'NONE',  ( 95.67376207875072680, 104.0454443415356991, -47.70000000000000995 ) ) ;
#4184=CARTESIAN_POINT ( 'NONE',  ( 102.0669872999999939, 123.5000000010924595, 0.8561741729129311862 ) ) ;
#4186=CARTESIAN_POINT ( 'NONE',  ( 102.1631189606246295, 103.3426043859339103, -43.90000000546237402 ) ) ;
#4199=CARTESIAN_POINT ( 'NONE',  ( 107.0000000000000142, 110.0000000000000000, -53.00000000000000711 ) ) ;
#4200=CARTESIAN_POINT ( 'NONE',  ( 84.99999999999998579, 123.0000000000000000, -13.00000000000000888 ) ) ;
#4202=CARTESIAN_POINT ( 'NONE',  ( 94.33688103937537051, 105.8855032339526758, -49.80000000000000426 ) ) ;
#4204=EDGE_LOOP ( 'NONE', ( #24878, #14436, #9981, #9822 ) ) ;
#4213=CARTESIAN_POINT ( 'NONE',  ( 93.00000000000000000, 110.0000000000000000, -46.50000000546238255 ) ) ;
#4220=CARTESIAN_POINT ( 'NONE',  ( 101.0355339059327378, 122.9500000021849502, 2.499999999999977796 ) ) ;
#4225=ORIENTED_EDGE ( 'NONE', *, *, #5130, .T. ) ;
#4229=VECTOR ( 'NONE', #1619, 1000.000000000000000 ) ;
#4234=CARTESIAN_POINT ( 'NONE',  ( 106.5389055433251002, 105.2492070361643215, -50.32500000273120122 ) ) ;
#4240=ORIENTED_EDGE ( 'NONE', *, *, #11098, .F. ) ;
#4248=AXIS2_PLACEMENT_3D ( 'NONE', #23430, #3486, #1362 ) ;
#4263=CARTESIAN_POINT ( 'NONE',  ( 102.4976396683250925, 117.6869444889999841, -47.97500000273119269 ) ) ;
#4269=CARTESIAN_POINT ( 'NONE',  ( 96.84719886470463734, 94.93749999863440792, 3.152801135295351997 ) ) ;
#4272=CARTESIAN_POINT ( 'NONE',  ( 102.1631189606246295, 103.3426043859339103, -45.40000000000001279 ) ) ;
#4273=ADVANCED_FACE ( 'NONE', ( #17486 ), #21925, .T. ) ;
#4277=CARTESIAN_POINT ( 'NONE',  ( 98.15313185440925281, 94.62499999863439371, -4.458734124999994997 ) ) ;
#4282=EDGE_LOOP ( 'NONE', ( #16873, #26377, #18015 ) ) ;
#4292=EDGE_CURVE ( 'NONE', #3863, #13215, #24052, .T. ) ;
#4298=LINE ( 'NONE', #21690, #22804 ) ;
#4305=CARTESIAN_POINT ( 'NONE',  ( 95.00472066334982912, 103.1245878333314323, -52.82500000273118701 ) ) ;
#4306=CARTESIAN_POINT ( 'NONE',  ( 107.0000000000000142, 110.0000000000000000, -55.00000000000000711 ) ) ;
#4320=CARTESIAN_POINT ( 'NONE',  ( 94.33688103937537051, 114.1144967660473242, -50.20000000000000995 ) ) ;
#4323=CARTESIAN_POINT ( 'NONE',  ( 99.14382582708707048, 123.0000000010925021, -2.066987299999999195 ) ) ;
#4329=ORIENTED_EDGE ( 'NONE', *, *, #8782, .F. ) ;
#4330=ORIENTED_EDGE ( 'NONE', *, *, #20686, .T. ) ;
#4339=DIRECTION ( 'NONE',  ( -0.000000000000000000, 1.000000000000000000, -0.000000000000000000 ) ) ;
#4341=CARTESIAN_POINT ( 'NONE',  ( 99.99999999999998579, 91.75000000000000000, 4.999999999999984013 ) ) ;
#4353=CARTESIAN_POINT ( 'NONE',  ( 99.99999999999998579, 125.0000000000000000, 2.499999999999985789 ) ) ;
#4357=CARTESIAN_POINT ( 'NONE',  ( 97.50236033167492167, 117.6869444889999841, -51.52500000273119696 ) ) ;
#4361=CARTESIAN_POINT ( 'NONE',  ( 97.50000000000000000, 122.7500000021849615, 1.035533905932725096 ) ) ;
#4367=VERTEX_POINT ( 'NONE', #3239 ) ;
#4368=CARTESIAN_POINT ( 'NONE',  ( 97.93301270000000613, 123.7500000010924879, -9.540979117872439019E-15 ) ) ;
#4372=CARTESIAN_POINT ( 'NONE',  ( 100.0000000000000000, 110.0000000000000000, -55.00000000000000711 ) ) ;
#4375=CARTESIAN_POINT ( 'NONE',  ( 91.91746824999999887, 110.0000000000000000, -49.12500000273119838 ) ) ;
#4388=ADVANCED_FACE ( 'NONE', ( #7074 ), #685, .F. ) ;
#4395=( BOUNDED_CURVE ( )  B_SPLINE_CURVE ( 2, ( #18183, #7340, #5364, #20476, #3221, #953, #2798 ),
 .UNSPECIFIED., .F., .T. ) 
 B_SPLINE_CURVE_WITH_KNOTS ( ( 3, 2, 2, 3 ),
 ( 0.7500000000000006661, 0.7750000000000004663, 0.8000000000000002665, 0.8250000005912483392 ),
 .UNSPECIFIED. ) 
 CURVE ( )  GEOMETRIC_REPRESENTATION_ITEM ( )  RATIONAL_B_SPLINE_CURVE ( ( 0.9999999999999980016, 0.9238795325112887369, 1.000000000000000000, 0.9238795325112867385, 1.000000000000000000, 0.9238795325112867385, 1.000000000000000000 ) ) 
 REPRESENTATION_ITEM ( '' )  );
#4398=CARTESIAN_POINT ( 'NONE',  ( 99.99999999999998579, 122.9000000021849530, 2.499999999999978684 ) ) ;
#4407=CARTESIAN_POINT ( 'NONE',  ( 95.00472066334981491, 116.8754121666685393, -47.67500000273120975 ) ) ;
#4411=CARTESIAN_POINT ( 'NONE',  ( 97.83688103937538472, 116.6573956140660897, -44.90000000546237402 ) ) ;
#4412=CARTESIAN_POINT ( 'NONE',  ( 95.54126587499999346, 93.74999999863439371, -1.846868145590737864 ) ) ;
#4413=CIRCLE ( 'NONE', #2137, 2.499999999999995115 ) ;
#4421=CARTESIAN_POINT ( 'NONE',  ( 101.8468681455907330, 93.49999999863442213, -4.458734124999994997 ) ) ;
#4444=DIRECTION ( 'NONE',  ( 1.000000000000000000, -0.000000000000000000, -5.782411586589357392E-17 ) ) ;
#4446=CARTESIAN_POINT ( 'NONE',  ( 91.91746824999999887, 110.0000000000000000, -49.12500000273119838 ) ) ;
#4453=CYLINDRICAL_SURFACE ( 'NONE', #13603, 4.999999999999989342 ) ;
#4463=CARTESIAN_POINT ( 'NONE',  ( 107.0000000000000142, 107.7255621263696526, -53.10000000000000142 ) ) ;
#4465=CARTESIAN_POINT ( 'NONE',  ( 103.5355339059327235, 92.99999999726881583, -3.535533905932738197 ) ) ;
#4469=CARTESIAN_POINT ( 'NONE',  ( 95.00000000000000000, 92.31249999726880162, -2.071067811865479058 ) ) ;
#4471=DIRECTION ( 'NONE',  ( 0.000000000000000000, 0.000000000000000000, -1.000000000000000000 ) ) ;
#4485=LINE ( 'NONE', #25860, #22307 ) ;
#4488=ORIENTED_EDGE ( 'NONE', *, *, #21320, .F. ) ;
#4504=CARTESIAN_POINT ( 'NONE',  ( 102.4999999999999716, 123.1500000021849672, -1.035533905932742638 ) ) ;
#4509=CARTESIAN_POINT ( 'NONE',  ( 102.0669872999999939, 124.1000000010924964, 0.8561741729129311862 ) ) ;
#4514=LINE ( 'NONE', #9624, #14211 ) ;
#4516=CARTESIAN_POINT ( 'NONE',  ( 95.00472066334982912, 103.1245878333314323, -45.07500000273119412 ) ) ;
#4528=COLOUR_RGB ( '', 0.08235294, 0.09019608, 0.10196078) ;
#4530=VECTOR ( 'NONE', #23690, 1000.000000000000000 ) ;
#4534=CARTESIAN_POINT ( 'NONE',  ( 104.9999999999999858, 93.00000000000000000, -6.938893903907228378E-15 ) ) ;
#4535=VERTEX_POINT ( 'NONE', #27332 ) ;
#4545=CARTESIAN_POINT ( 'NONE',  ( 95.00472066334981491, 116.8754121666685393, -45.67500000273119554 ) ) ;
#4550=CARTESIAN_POINT ( 'NONE',  ( 101.0337790074118658, 123.0000000000000000, -2.280707637605766891 ) ) ;
#4558=CARTESIAN_POINT ( 'NONE',  ( 98.15313185440925281, 94.99999999863439371, 4.458734124999979898 ) ) ;
#4579=CARTESIAN_POINT ( 'NONE',  ( 103.5355339059327235, 92.12500000000000000, -3.535533905932738197 ) ) ;
#4583=CARTESIAN_POINT ( 'NONE',  ( 102.4976396683250925, 102.3130555110000159, -50.52500000273119696 ) ) ;
#4594=ORIENTED_EDGE ( 'NONE', *, *, #11950, .F. ) ;
#4599=CARTESIAN_POINT ( 'NONE',  ( 94.33688103937537051, 114.1144967660473242, -48.20000000000000995 ) ) ;
#4602=CARTESIAN_POINT ( 'NONE',  ( 101.7677669529663547, 123.0999999999999943, -1.767766952966370209 ) ) ;
#4608=CARTESIAN_POINT ( 'NONE',  ( 99.99999999999998579, 92.12499999726880162, -4.999999999999997335 ) ) ;
#4625=CARTESIAN_POINT ( 'NONE',  ( 104.3262379212492590, 104.0454443415356991, -49.30000000000000426 ) ) ;
#4627=EDGE_CURVE ( 'NONE', #11152, #4858, #10052, .T. ) ;
#4645=CARTESIAN_POINT ( 'NONE',  ( 101.7677669529663547, 122.4000000021849530, -1.767766952966370209 ) ) ;
#4647=ORIENTED_EDGE ( 'NONE', *, *, #484, .T. ) ;
#4651=CARTESIAN_POINT ( 'NONE',  ( 101.7677669529663547, 122.4000000021849530, -1.767766952966370209 ) ) ;
#4658=CARTESIAN_POINT ( 'NONE',  ( 102.4976396683250925, 117.6869444889999841, -53.72500000273119980 ) ) ;
#4676=CARTESIAN_POINT ( 'NONE',  ( 99.99999999999998579, 124.1000000021849416, -2.499999999999997780 ) ) ;
#4687=CARTESIAN_POINT ( 'NONE',  ( 102.1631189606246295, 116.6573956140660897, -54.60000000000000853 ) ) ;
#4695=CARTESIAN_POINT ( 'NONE',  ( 98.57518772780328220, 123.0000000000000284, -2.059818896815785561 ) ) ;
#4702=CARTESIAN_POINT ( 'NONE',  ( 100.0000000000000000, 110.0000000000000000, -55.00000000000000711 ) ) ;
#4704=CARTESIAN_POINT ( 'NONE',  ( 99.99999999999998579, 93.56249999863440792, -4.458734124999994997 ) ) ;
#4710=CARTESIAN_POINT ( 'NONE',  ( 99.99999999999998579, 95.62499999726881583, 4.999999999999984013 ) ) ;
#4729=CARTESIAN_POINT ( 'NONE',  ( 106.5389055433251002, 114.7507929638356785, -47.92500000273120264 ) ) ;
#4737=( BOUNDED_CURVE ( )  B_SPLINE_CURVE ( 2, ( #5623, #6037, #14703, #27703, #27422, #18587, #23287, #27292, #12556 ),
 .UNSPECIFIED., .F., .F. ) 
 B_SPLINE_CURVE_WITH_KNOTS ( ( 3, 2, 2, 2, 3 ),
 ( 0.6500000000000005773, 0.6750000000000005995, 0.7000000000000006217, 0.7250000000000006439, 0.7500000000000006661 ),
 .UNSPECIFIED. ) 
 CURVE ( )  GEOMETRIC_REPRESENTATION_ITEM ( )  RATIONAL_B_SPLINE_CURVE ( ( 0.9999999999999983347, 0.9238795325112884038, 1.000000000000000000, 0.9238795325112867385, 1.000000000000000000, 0.9238795325112867385, 1.000000000000000000, 0.9238795325112847401, 1.000000000000001998 ) ) 
 REPRESENTATION_ITEM ( '' )  );
#4746=CARTESIAN_POINT ( 'NONE',  ( 97.50236033167492167, 102.3130555110000159, -50.97500000273119980 ) ) ;
#4748=CARTESIAN_POINT ( 'NONE',  ( 97.50000000000000000, 123.3499999999999943, -1.035533905932742416 ) ) ;
#4752=CARTESIAN_POINT ( 'NONE',  ( 104.9999999999999858, 93.87499999726881583, -6.938893903907228378E-15 ) ) ;
#4762=CARTESIAN_POINT ( 'NONE',  ( 104.9999999999999716, 90.93749999726880162, -2.071067811865478170 ) ) ;
#4765=CARTESIAN_POINT ( 'NONE',  ( 104.4587341249999781, 91.56249999863440792, -6.938893903907228378E-15 ) ) ;
#4768=ORIENTED_EDGE ( 'NONE', *, *, #13826, .T. ) ;
#4782=EDGE_CURVE ( 'NONE', #9459, #3810, #28017, .T. ) ;
#4789=VECTOR ( 'NONE', #16854, 1000.000000000000000 ) ;
#4793=CARTESIAN_POINT ( 'NONE',  ( 97.93301270000000613, 122.9500000010924765, -9.540979117872439019E-15 ) ) ;
#4796=EDGE_CURVE ( 'NONE', #923, #7889, #3573, .T. ) ;
#4830=CARTESIAN_POINT ( 'NONE',  ( 99.99999999999998579, 94.12499999726881583, -4.999999999999997335 ) ) ;
#4843=CARTESIAN_POINT ( 'NONE',  ( 99.91426332765584561, 123.0000000000000142, -2.514867278806395490 ) ) ;
#4850=CARTESIAN_POINT ( 'NONE',  ( 99.99999999999998579, 94.56249999863440792, -4.458734124999994997 ) ) ;
#4855=FACE_OUTER_BOUND ( 'NONE', #14463, .T. ) ;
#4858=VERTEX_POINT ( 'NONE', #4353 ) ;
#4870=AXIS2_PLACEMENT_3D ( 'NONE', #16199, #16481, #27470 ) ;
#4875=CARTESIAN_POINT ( 'NONE',  ( 106.5389055433251002, 105.2492070361643215, -44.32500000273119412 ) ) ;
#4881=EDGE_LOOP ( 'NONE', ( #7112, #20946, #1430, #23796, #19657, #22088 ) ) ;
#4885=CARTESIAN_POINT ( 'NONE',  ( 99.99999999999998579, 123.3000000021849587, -2.499999999999997780 ) ) ;
#4891=CARTESIAN_POINT ( 'NONE',  ( 108.0825317500000011, 107.3738262389971538, -52.47500000273118559 ) ) ;
#4893=CARTESIAN_POINT ( 'NONE',  ( 102.0669872999999797, 122.7500000010924737, -9.794112055954760458E-15 ) ) ;
#4897=CARTESIAN_POINT ( 'NONE',  ( 99.99999999999998579, 94.12499999726881583, -4.999999999999997335 ) ) ;
#4902=CARTESIAN_POINT ( 'NONE',  ( 102.4976396683250925, 117.6869444889999841, -53.97500000273119980 ) ) ;
#4907=( BOUNDED_CURVE ( )  B_SPLINE_CURVE ( 2, ( #9815, #13793, #15937, #24788, #14363, #11513, #2981, #11801, #9389 ),
 .UNSPECIFIED., .F., .F. ) 
 B_SPLINE_CURVE_WITH_KNOTS ( ( 3, 2, 2, 2, 3 ),
 ( 0.8500000000000007550, 0.8750000000000008882, 0.9000000000000009104, 0.9250000000000009326, 0.9500000000000009548 ),
 .UNSPECIFIED. ) 
 CURVE ( )  GEOMETRIC_REPRESENTATION_ITEM ( )  RATIONAL_B_SPLINE_CURVE ( ( 0.9999999999999976685, 0.9238795325112890700, 1.000000000000000000, 0.9238795325112867385, 1.000000000000000000, 0.9238795325112867385, 1.000000000000000000, 0.9238795325112837409, 1.000000000000003109 ) ) 
 REPRESENTATION_ITEM ( '' )  );
#4929=CARTESIAN_POINT ( 'NONE',  ( 102.4976396683250925, 117.6869444889999841, -47.72500000273119269 ) ) ;
#4931=CARTESIAN_POINT ( 'NONE',  ( 109.0000000000000142, 110.0000000000000000, -45.00000000000000711 ) ) ;
#4937=CARTESIAN_POINT ( 'NONE',  ( 102.4999999999999716, 122.3500000021849701, -1.035533905932742638 ) ) ;
#4943=CARTESIAN_POINT ( 'NONE',  ( 93.46109445667491400, 114.7507929638356785, -45.32500000273119412 ) ) ;
#4945=CARTESIAN_POINT ( 'NONE',  ( 96.84719886470463734, 91.93749999863440792, 3.152801135295351997 ) ) ;
#4946=CARTESIAN_POINT ( 'NONE',  ( 97.83688103937538472, 116.6573956140660897, -48.90000000546238113 ) ) ;
#4948=CARTESIAN_POINT ( 'NONE',  ( 96.46446609406726225, 91.49999999726880162, 3.535533905932723986 ) ) ;
#4950=VERTEX_POINT ( 'NONE', #2501 ) ;
#4951=ORIENTED_EDGE ( 'NONE', *, *, #4782, .T. ) ;
#4979=DIRECTION ( 'NONE',  ( -0.8660254037844418162, -0.4999999999999947264, 0.000000000000000000 ) ) ;
#4982=CARTESIAN_POINT ( 'NONE',  ( 93.46109445667491400, 114.7507929638356785, -53.57500000273119412 ) ) ;
#4983=CARTESIAN_POINT ( 'NONE',  ( 101.4086053019245099, 123.0000000000000000, -2.070951898149314907 ) ) ;
#4985=EDGE_CURVE ( 'NONE', #7822, #24826, #6464, .T. ) ;
#4994=CARTESIAN_POINT ( 'NONE',  ( 97.92893218813452449, 93.68750000000000000, 4.999999999999983125 ) ) ;
#4995=AXIS2_PLACEMENT_3D ( 'NONE', #17155, #21165, #17295 ) ;
#4996=CARTESIAN_POINT ( 'NONE',  ( 101.8468681455907330, 94.74999999863440792, -4.458734124999994997 ) ) ;
#5000=ORIENTED_EDGE ( 'NONE', *, *, #2221, .T. ) ;
#5011=CARTESIAN_POINT ( 'NONE',  ( 98.15313185440923860, 91.99999999863439371, 4.458734124999980786 ) ) ;
#5017=CARTESIAN_POINT ( 'NONE',  ( 107.0000000000000142, 110.0000000000000000, -53.50000000546238255 ) ) ;
#5018=CARTESIAN_POINT ( 'NONE',  ( 101.8468681455907330, 92.37499999863440792, 4.458734124999979898 ) ) ;
#5024=CARTESIAN_POINT ( 'NONE',  ( 96.46446609406726225, 91.62500000000000000, 3.535533905932723986 ) ) ;
#5028=ORIENTED_EDGE ( 'NONE', *, *, #18718, .F. ) ;
#5032=CARTESIAN_POINT ( 'NONE',  ( 102.4976396683250925, 102.3130555110000159, -52.77500000273119696 ) ) ;
#5039=CARTESIAN_POINT ( 'NONE',  ( 96.46446609406726225, 93.49999999726881583, 3.535533905932723986 ) ) ;
#5042=CARTESIAN_POINT ( 'NONE',  ( 99.99999999999998579, 118.4984768113314146, -49.87500000273118417 ) ) ;
#5044=CARTESIAN_POINT ( 'NONE',  ( 101.0355339059327235, 123.2500000021849615, -2.499999999999998668 ) ) ;
#5048=CARTESIAN_POINT ( 'NONE',  ( 84.99999999999998579, 95.00000000000000000, 14.99999999999999467 ) ) ;
#5056=ORIENTED_EDGE ( 'NONE', *, *, #71, .T. ) ;
#5069=CARTESIAN_POINT ( 'NONE',  ( 99.99999999999998579, 101.5015231886685712, -46.62500000273119838 ) ) ;
#5078=ORIENTED_EDGE ( 'NONE', *, *, #17322, .T. ) ;
#5084=CARTESIAN_POINT ( 'NONE',  ( 95.54126587499999346, 92.87499999863440792, 1.846868145590722543 ) ) ;
#5085=CARTESIAN_POINT ( 'NONE',  ( 91.91746824999998466, 112.6261737610028320, -47.22500000273119269 ) ) ;
#5087=CARTESIAN_POINT ( 'NONE',  ( 107.0000000000000142, 110.0000000000000000, -49.50000000546238255 ) ) ;
#5107=CARTESIAN_POINT ( 'NONE',  ( 99.99999999999998579, 89.99899999999999523, 2.499999999999985789 ) ) ;
#5108=CARTESIAN_POINT ( 'NONE',  ( 96.46446609406726225, 94.49999999726881583, 3.535533905932723986 ) ) ;
#5111=DIRECTION ( 'NONE',  ( 5.782411586589357392E-17, -0.000000000000000000, 1.000000000000000000 ) ) ;
#5119=CARTESIAN_POINT ( 'NONE',  ( 102.4976396683250925, 117.6869444889999841, -51.97500000273119980 ) ) ;
#5121=CARTESIAN_POINT ( 'NONE',  ( 99.99999999999998579, 123.1500000010924794, 2.066987299999980099 ) ) ;
#5128=CARTESIAN_POINT ( 'NONE',  ( 103.5355339059327235, 92.12500000000000000, -3.535533905932738197 ) ) ;
#5130=EDGE_CURVE ( 'NONE', #14907, #1287, #938, .T. ) ;
#5136=VECTOR ( 'NONE', #14065, 1000.000000000000000 ) ;
#5148=CARTESIAN_POINT ( 'NONE',  ( 84.99999999999998579, 120.0000000000000000, -43.00000000000000000 ) ) ;
#5149=CARTESIAN_POINT ( 'NONE',  ( 103.1528011352953484, 92.43749999863440792, -3.152801135295366208 ) ) ;
#5156=CARTESIAN_POINT ( 'NONE',  ( 91.91746824999999887, 110.0000000000000000, -45.12500000273119838 ) ) ;
#5157=CARTESIAN_POINT ( 'NONE',  ( 95.54126587500000767, 92.06249999863440792, -7.484931351350258973E-15 ) ) ;
#5158=DIRECTION ( 'NONE',  ( 0.000000000000000000, 0.000000000000000000, -1.000000000000000000 ) ) ;
#5161=VECTOR ( 'NONE', #22435, 1000.000000000000000 ) ;
#5163=ORIENTED_EDGE ( 'NONE', *, *, #24104, .T. ) ;
#5167=ORIENTED_EDGE ( 'NONE', *, *, #7425, .T. ) ;
#5170=EDGE_CURVE ( 'NONE', #21081, #21036, #490, .T. ) ;
#5172=CARTESIAN_POINT ( 'NONE',  ( 105.6631189606246295, 114.1144967660473242, -46.80000000000001137 ) ) ;
#5174=CARTESIAN_POINT ( 'NONE',  ( 98.96446609406727646, 124.3499999999999943, 2.499999999999977796 ) ) ;
#5181=CARTESIAN_POINT ( 'NONE',  ( 96.84719886470463734, 94.18749999863440792, 3.152801135295351997 ) ) ;
#5183=CARTESIAN_POINT ( 'NONE',  ( 95.00472066334981491, 103.1245878333314465, -49.07500000273119412 ) ) ;
#5184=ADVANCED_FACE ( 'NONE', ( #21147 ), #5911, .T. ) ;
#5189=CARTESIAN_POINT ( 'NONE',  ( 102.4999999999999858, 124.6500000000000057, -1.035533905932742638 ) ) ;
#5205=EDGE_LOOP ( 'NONE', ( #2807, #11369, #18826, #27889 ) ) ;
#5208=CARTESIAN_POINT ( 'NONE',  ( 99.99999999999998579, 89.99899999999999523, -2.500000000000004885 ) ) ;
#5211=CARTESIAN_POINT ( 'NONE',  ( 97.50236033167492167, 102.3130555110000159, -44.72500000273119980 ) ) ;
#5212=DIRECTION ( 'NONE',  ( 0.000000000000000000, -1.000000000000000000, 3.469446951953611231E-16 ) ) ;
#5231=ORIENTED_EDGE ( 'NONE', *, *, #20288, .T. ) ;
#5244=VECTOR ( 'NONE', #10779, 1000.000000000000000 ) ;
#5245=PLANE ( 'NONE',  #22570 ) ;
#5248=CARTESIAN_POINT ( 'NONE',  ( 98.96446609406727646, 124.0569999999781459, -2.499999999999997780 ) ) ;
#5252=CARTESIAN_POINT ( 'NONE',  ( 84.99999999999998579, 100.0000000000000000, -15.00000000000000533 ) ) ;
#5272=CARTESIAN_POINT ( 'NONE',  ( 102.0710678118654613, 93.18749999999998579, -4.999999999999997335 ) ) ;
#5291=CARTESIAN_POINT ( 'NONE',  ( 95.54126587500000767, 91.81249999863440792, -7.484931351350258973E-15 ) ) ;
#5296=CARTESIAN_POINT ( 'NONE',  ( 97.50000000000000000, 123.3999999999999915, -9.540979117872439019E-15 ) ) ;
#5298=CARTESIAN_POINT ( 'NONE',  ( 106.5389055433251002, 105.2492070361643215, -48.32500000273119412 ) ) ;
#5299=CARTESIAN_POINT ( 'NONE',  ( 103.1528011352953484, 92.68749999863440792, -3.152801135295366208 ) ) ;
#5300=VECTOR ( 'NONE', #5371, 1000.000000000000000 ) ;
#5304=ORIENTED_EDGE ( 'NONE', *, *, #17554, .T. ) ;
#5309=ADVANCED_FACE ( 'NONE', ( #21289 ), #19030, .T. ) ;
#5315=CARTESIAN_POINT ( 'NONE',  ( 97.83688103937537051, 103.3426043859339103, -45.60000000000000853 ) ) ;
#5324=CARTESIAN_POINT ( 'NONE',  ( 95.54126587500000767, 92.06249999863440792, -7.484931351350258973E-15 ) ) ;
#5337=CARTESIAN_POINT ( 'NONE',  ( 95.54126587499999346, 92.12499999863440792, 1.846868145590722543 ) ) ;
#5355=CARTESIAN_POINT ( 'NONE',  ( 106.5389055433251002, 114.7507929638356785, -47.92500000273120264 ) ) ;
#5356=DIRECTION ( 'NONE',  ( 0.000000000000000000, 1.000000000000000000, -1.156482317317871478E-16 ) ) ;
#5360=VERTEX_POINT ( 'NONE', #1254 ) ;
#5364=CARTESIAN_POINT ( 'NONE',  ( 103.5355339059327235, 94.74999999726881583, 3.535533905932724874 ) ) ;
#5367=CARTESIAN_POINT ( 'NONE',  ( 104.9952793366501851, 116.8754121666685393, -47.82500000273119412 ) ) ;
#5371=DIRECTION ( 'NONE',  ( 0.000000000000000000, -1.000000000000000000, 0.000000000000000000 ) ) ;
#5384=CARTESIAN_POINT ( 'NONE',  ( 87.00000000000000000, 102.0000000000000142, -13.00000000000000533 ) ) ;
#5391=CARTESIAN_POINT ( 'NONE',  ( 97.50000000000000000, 124.9569999999781658, -1.035533905932742416 ) ) ;
#5392=AXIS2_PLACEMENT_3D ( 'NONE', #15036, #15174, #17609 ) ;
#5395=CARTESIAN_POINT ( 'NONE',  ( 93.00000000000000000, 110.0000000000000000, -48.00000000000000711 ) ) ;
#5408=( BOUNDED_CURVE ( )  B_SPLINE_CURVE ( 2, ( #27891, #8352, #23611, #4088, #12752, #18776, #14485, #21475, #1951, #16495, #25189 ),
 .UNSPECIFIED., .F., .F. ) 
 B_SPLINE_CURVE_WITH_KNOTS ( ( 3, 2, 2, 2, 2, 3 ),
 ( 0.4999999999999996669, 0.5199999999999996847, 0.5399999999999998135, 0.5599999999999998312, 0.5799999999999998490, 0.5999999999999998668 ),
 .UNSPECIFIED. ) 
 CURVE ( )  GEOMETRIC_REPRESENTATION_ITEM ( )  RATIONAL_B_SPLINE_CURVE ( ( 1.000000000000000888, 0.9510565162951527540, 1.000000000000000000, 0.9510565162951535312, 1.000000000000000000, 0.9510565162951535312, 1.000000000000000000, 0.9510565162951535312, 1.000000000000000000, 0.9510565162951537532, 0.9999999999999997780 ) ) 
 REPRESENTATION_ITEM ( '' )  );
#5410=CARTESIAN_POINT ( 'NONE',  ( 99.14382582708707048, 123.6000000010924680, -2.066987299999999195 ) ) ;
#5418=CARTESIAN_POINT ( 'NONE',  ( 102.0710678118654613, 91.18749999999998579, -4.999999999999997335 ) ) ;
#5424=VERTEX_POINT ( 'NONE', #5384 ) ;
#5433=EDGE_CURVE ( 'NONE', #1189, #15184, #1608, .T. ) ;
#5434=CARTESIAN_POINT ( 'NONE',  ( 102.1631189606246295, 103.3426043859339103, -49.90000000546238113 ) ) ;
#5435=CARTESIAN_POINT ( 'NONE',  ( 104.4587341249999923, 90.37499999863440792, -1.846868145590737198 ) ) ;
#5439=CARTESIAN_POINT ( 'NONE',  ( 107.0000000000000142, 110.0000000000000000, -53.50000000546238255 ) ) ;
#5441=CARTESIAN_POINT ( 'NONE',  ( 107.0000000000000142, 110.0000000000000000, -51.50000000546237544 ) ) ;
#5442=CARTESIAN_POINT ( 'NONE',  ( 97.50000000000000000, 124.3000000021849587, -9.540979117872439019E-15 ) ) ;
#5455=CARTESIAN_POINT ( 'NONE',  ( 108.0825317500000011, 107.3738262389971538, -46.47500000273117848 ) ) ;
#5463=CARTESIAN_POINT ( 'NONE',  ( 99.99999999999998579, 92.31249999863440792, 4.458734124999981674 ) ) ;
#5464=FACE_OUTER_BOUND ( 'NONE', #9049, .T. ) ;
#5470=FACE_BOUND ( 'NONE', #18443, .T. ) ;
#5489=CARTESIAN_POINT ( 'NONE',  ( 107.0000000000000142, 110.0000000000000000, -55.00000000000000711 ) ) ;
#5494=CARTESIAN_POINT ( 'NONE',  ( 104.9999999999999858, 90.00000000000000000, -6.938893903907228378E-15 ) ) ;
#5535=FACE_OUTER_BOUND ( 'NONE', #18126, .T. ) ;
#5539=CARTESIAN_POINT ( 'NONE',  ( 105.6631189606246295, 105.8855032339526758, -47.20000000000000284 ) ) ;
#5547=EDGE_CURVE ( 'NONE', #11898, #8127, #6302, .T. ) ;
#5550=CARTESIAN_POINT ( 'NONE',  ( 99.99999999999998579, 125.0000000000000000, -9.540979117872439019E-15 ) ) ;
#5552=CARTESIAN_POINT ( 'NONE',  ( 96.46446609406726225, 90.62500000000000000, 3.535533905932723986 ) ) ;
#5553=CARTESIAN_POINT ( 'NONE',  ( 101.3296865857814311, 123.0000000000000000, 2.137053098915790539 ) ) ;
#5561=CARTESIAN_POINT ( 'NONE',  ( 104.9999999999999858, 90.43749999863440792, -6.938893903907228378E-15 ) ) ;
#5575=DIRECTION ( 'NONE',  ( -0.000000000000000000, -0.000000000000000000, 1.000000000000000000 ) ) ;
#5578=CARTESIAN_POINT ( 'NONE',  ( 104.4587341249999923, 91.24999999863439371, 1.846868145590726318 ) ) ;
#5585=CARTESIAN_POINT ( 'NONE',  ( 95.67376207875072680, 104.0454443415356991, -48.20000000546237828 ) ) ;
#5586=CARTESIAN_POINT ( 'NONE',  ( 99.99999999999998579, 90.56249999863440792, -4.458734124999994997 ) ) ;
#5599=CARTESIAN_POINT ( 'NONE',  ( 106.5389055433251002, 105.2492070361643215, -44.57500000273119412 ) ) ;
#5605=CARTESIAN_POINT ( 'NONE',  ( 95.54126587499999346, 93.12499999863439371, 1.846868145590722543 ) ) ;
#5606=CARTESIAN_POINT ( 'NONE',  ( 84.99999999999998579, 100.0000000000000000, -15.00000000000000533 ) ) ;
#5623=CARTESIAN_POINT ( 'NONE',  ( 99.99999999999998579, 93.25000000000000000, -4.999999999999997335 ) ) ;
#5632=DIRECTION ( 'NONE',  ( 0.000000000000000000, 4.625929269271485914E-16, 1.000000000000000000 ) ) ;
#5637=LINE ( 'NONE', #21297, #21902 ) ;
#5640=( LENGTH_UNIT ( ) NAMED_UNIT ( * ) SI_UNIT ( .MILLI., .METRE. ) );
#5644=CARTESIAN_POINT ( 'NONE',  ( 95.67376207875072680, 104.0454443415356991, -52.20000000546237828 ) ) ;
#5653=ORIENTED_EDGE ( 'NONE', *, *, #5170, .F. ) ;
#5662=ADVANCED_FACE ( 'NONE', ( #23142 ), #8579, .F. ) ;
#5671=CARTESIAN_POINT ( 'NONE',  ( 97.50000000000000000, 123.4500000000000028, 1.035533905932725096 ) ) ;
#5687=CARTESIAN_POINT ( 'NONE',  ( 104.9952793366501851, 103.1245878333314323, -46.67500000273118843 ) ) ;
#5688=CARTESIAN_POINT ( 'NONE',  ( 103.5355339059327235, 94.12500000000000000, -3.535533905932738197 ) ) ;
#5689=CARTESIAN_POINT ( 'NONE',  ( 100.8561741729129295, 124.2000000010924907, 2.066987299999979211 ) ) ;
#5693=EDGE_CURVE ( 'NONE', #2287, #24513, #14168, .T. ) ;
#5694=VERTEX_POINT ( 'NONE', #10841 ) ;
#5706=VERTEX_POINT ( 'NONE', #15258 ) ;
#5715=CARTESIAN_POINT ( 'NONE',  ( 95.54126587500000767, 93.81249999863440792, -7.484931351350258973E-15 ) ) ;
#5724=CARTESIAN_POINT ( 'NONE',  ( 93.00000000000000000, 110.0000000000000000, -48.50000000546238255 ) ) ;
#5725=CARTESIAN_POINT ( 'NONE',  ( 103.1528011352953484, 93.68749999863440792, -3.152801135295366208 ) ) ;
#5732=CARTESIAN_POINT ( 'NONE',  ( 99.99999999999998579, 91.06249999863440792, 4.458734124999981674 ) ) ;
#5734=VERTEX_POINT ( 'NONE', #605 ) ;
#5738=CARTESIAN_POINT ( 'NONE',  ( 97.50236033167492167, 117.6869444889999841, -49.77500000273119696 ) ) ;
#5753=DIRECTION ( 'NONE',  ( 0.000000000000000000, 1.000000000000000000, 0.000000000000000000 ) ) ;
#5757=CARTESIAN_POINT ( 'NONE',  ( 101.4615807364564546, 124.0500000010924850, 1.461580736456455476 ) ) ;
#5758=CARTESIAN_POINT ( 'NONE',  ( 96.84719886470463734, 93.93749999863440792, -3.152801135295366208 ) ) ;
#5769=DIRECTION ( 'NONE',  ( 5.782411586589357392E-17, -0.000000000000000000, 1.000000000000000000 ) ) ;
#5772=CARTESIAN_POINT ( 'NONE',  ( 97.83688103937537051, 103.3426043859339103, -44.10000000546238397 ) ) ;
#5784=DIRECTION ( 'NONE',  ( 0.000000000000000000, 0.000000000000000000, 1.000000000000000000 ) ) ;
#5805=CARTESIAN_POINT ( 'NONE',  ( 107.0000000000000142, 110.0000000000000000, -49.00000000000000711 ) ) ;
#5809=CARTESIAN_POINT ( 'NONE',  ( 97.50000000000000000, 125.0184775906502068, 0.3826834323650784575 ) ) ;
#5816=CARTESIAN_POINT ( 'NONE',  ( 102.4999999999999716, 123.9500000021849502, -1.035533905932742638 ) ) ;
#5820=CARTESIAN_POINT ( 'NONE',  ( 99.99999999999998579, 90.00000000000000000, -6.938893903907228378E-15 ) ) ;
#5824=CARTESIAN_POINT ( 'NONE',  ( 102.4976396683250925, 102.3130555110000159, -48.77500000273119696 ) ) ;
#5827=CARTESIAN_POINT ( 'NONE',  ( 97.93301270000000613, 122.9500000010924765, -9.540979117872439019E-15 ) ) ;
#5831=EDGE_LOOP ( 'NONE', ( #3312, #12341, #14432, #5000 ) ) ;
#5835=CARTESIAN_POINT ( 'NONE',  ( 95.00000000000000000, 94.50000000000000000, -7.551217303480904118E-15 ) ) ;
#5849=CARTESIAN_POINT ( 'NONE',  ( 102.4976396683250925, 117.6869444889999841, -49.97500000273119269 ) ) ;
#5858=CARTESIAN_POINT ( 'NONE',  ( 93.00000000000001421, 107.7255621263696668, -50.40000000546238823 ) ) ;
#5859=CARTESIAN_POINT ( 'NONE',  ( 95.54126587499999346, 90.74999999863439371, -1.846868145590737864 ) ) ;
#5863=EDGE_CURVE ( 'NONE', #21579, #9459, #19692, .T. ) ;
#5864=VECTOR ( 'NONE', #4979, 999.9999999999998863 ) ;
#5868=ORIENTED_EDGE ( 'NONE', *, *, #16537, .T. ) ;
#5869=EDGE_CURVE ( 'NONE', #23013, #11839, #17552, .T. ) ;
#5874=ORIENTED_EDGE ( 'NONE', *, *, #6004, .F. ) ;
#5875=CARTESIAN_POINT ( 'NONE',  ( 95.00472066334982912, 116.8754121666685393, -47.67500000273120264 ) ) ;
#5879=CARTESIAN_POINT ( 'NONE',  ( 102.4976396683250925, 102.3130555110000159, -50.52500000273119696 ) ) ;
#5880=AXIS2_PLACEMENT_3D ( 'NONE', #11450, #7178, #7467 ) ;
#5899=CARTESIAN_POINT ( 'NONE',  ( 95.54126587500000767, 93.06249999863440792, -7.484931351350258973E-15 ) ) ;
#5908=CARTESIAN_POINT ( 'NONE',  ( 99.99999999999998579, 90.00000000000000000, -6.938893903907228378E-15 ) ) ;
#5911=PLANE ( 'NONE',  #3411 ) ;
#5915=CARTESIAN_POINT ( 'NONE',  ( 95.67376207875072680, 104.0454443415356991, -44.20000000546236407 ) ) ;
#5919=ORIENTED_EDGE ( 'NONE', *, *, #20742, .T. ) ;
#5925=FACE_OUTER_BOUND ( 'NONE', #4204, .T. ) ;
#5935=EDGE_CURVE ( 'NONE', #27080, #8561, #17072, .T. ) ;
#5939=CARTESIAN_POINT ( 'NONE',  ( 95.67376207875072680, 115.9545556584642867, -48.30000000000001137 ) ) ;
#5941=LINE ( 'NONE', #11133, #24366 ) ;
#5944=CARTESIAN_POINT ( 'NONE',  ( 101.0355339059327378, 123.6500000000000199, 2.499999999999977796 ) ) ;
#5952=CARTESIAN_POINT ( 'NONE',  ( 98.96446609406727646, 123.6500000021849530, 2.499999999999977796 ) ) ;
#5958=CARTESIAN_POINT ( 'NONE',  ( 108.0825317500000153, 110.0000000000000000, -46.37500000273119838 ) ) ;
#5960=CARTESIAN_POINT ( 'NONE',  ( 99.99999999999998579, 122.9500000010924765, -2.066987299999998751 ) ) ;
#5968=CARTESIAN_POINT ( 'NONE',  ( 104.9999999999999716, 94.93750000000000000, 2.071067811865467956 ) ) ;
#5984=DIRECTION ( 'NONE',  ( 0.000000000000000000, 0.000000000000000000, -1.000000000000000000 ) ) ;
#5993=CARTESIAN_POINT ( 'NONE',  ( 104.3262379212492590, 104.0454443415356991, -51.80000000546238681 ) ) ;
#5994=CARTESIAN_POINT ( 'NONE',  ( 99.99999999999998579, 91.06249999863440792, 4.458734124999981674 ) ) ;
#6002=VERTEX_POINT ( 'NONE', #8670 ) ;
#6004=EDGE_CURVE ( 'NONE', #24017, #21579, #6395, .T. ) ;
#6009=CARTESIAN_POINT ( 'NONE',  ( 108.0825317500000153, 110.0000000000000000, -50.37500000273119127 ) ) ;
#6020=DIRECTION ( 'NONE',  ( 1.000000000000000000, 0.000000000000000000, 0.000000000000000000 ) ) ;
#6034=LINE ( 'NONE', #25554, #8916 ) ;
#6037=CARTESIAN_POINT ( 'NONE',  ( 97.92893218813448186, 93.31249999999998579, -4.999999999999963585 ) ) ;
#6054=ORIENTED_EDGE ( 'NONE', *, *, #3941, .F. ) ;
#6055=ORIENTED_EDGE ( 'NONE', *, *, #10957, .T. ) ;
#6059=CARTESIAN_POINT ( 'NONE',  ( 97.83688103937537051, 103.3426043859339103, -52.10000000546238397 ) ) ;
#6080=CARTESIAN_POINT ( 'NONE',  ( 98.23223304703363112, 123.5000000000000000, 1.767766952966351557 ) ) ;
#6082=CARTESIAN_POINT ( 'NONE',  ( 102.0669872999999797, 123.5500000010924708, -9.794112055954760458E-15 ) ) ;
#6094=CARTESIAN_POINT ( 'NONE',  ( 91.91746824999998466, 107.3738262389971538, -51.27500000273119696 ) ) ;
#6111=CARTESIAN_POINT ( 'NONE',  ( 97.83688103937538472, 116.6573956140660897, -52.40000000000000568 ) ) ;
#6116=CARTESIAN_POINT ( 'NONE',  ( 93.00000000000000000, 110.0000000000000000, -55.00000000000000711 ) ) ;
#6126=EDGE_CURVE ( 'NONE', #25694, #5706, #24758, .T. ) ;
#6129=CARTESIAN_POINT ( 'NONE',  ( 103.1528011352953484, 91.18749999863440792, 3.152801135295352886 ) ) ;
#6148=CARTESIAN_POINT ( 'NONE',  ( 84.99999999999998579, 95.00000000000000000, 14.99999999999999467 ) ) ;
#6158=CARTESIAN_POINT ( 'NONE',  ( 91.91746824999998466, 112.6261737610028320, -53.22500000273119269 ) ) ;
#6167=CARTESIAN_POINT ( 'NONE',  ( 97.93301270000000613, 124.5500000010924850, -9.540979117872439019E-15 ) ) ;
#6173=VERTEX_POINT ( 'NONE', #10932 ) ;
#6178=CARTESIAN_POINT ( 'NONE',  ( 94.33688103937537051, 105.8855032339526758, -51.80000000000000426 ) ) ;
#6181=CARTESIAN_POINT ( 'NONE',  ( 101.4615807364564546, 124.4500000010924765, -1.461580736456474794 ) ) ;
#6193=CARTESIAN_POINT ( 'NONE',  ( 96.46446609406726225, 92.24999999726880162, -3.535533905932738197 ) ) ;
#6194=CARTESIAN_POINT ( 'NONE',  ( 105.6631189606246295, 105.8855032339526758, -51.70000000546237828 ) ) ;
#6198=CARTESIAN_POINT ( 'NONE',  ( 99.99999999999998579, 93.75000000000000000, 4.999999999999984013 ) ) ;
#6213=CIRCLE ( 'NONE', #11648, 5.000000000000004441 ) ;
#6218=CARTESIAN_POINT ( 'NONE',  ( 98.96446609406726225, 124.0499999999999829, -2.499999999999998668 ) ) ;
#6219=CARTESIAN_POINT ( 'NONE',  ( 98.96446609406727646, 124.3499999999999943, 2.499999999999977796 ) ) ;
#6221=CARTESIAN_POINT ( 'NONE',  ( 99.14382582708708469, 124.6000000010924822, -2.066987299999998751 ) ) ;
#6226=CARTESIAN_POINT ( 'NONE',  ( 97.50000000000000000, 124.2500000021849758, -1.035533905932742416 ) ) ;
#6233=CARTESIAN_POINT ( 'NONE',  ( 91.91746824999999887, 110.0000000000000000, -45.37500000273119838 ) ) ;
#6263=CARTESIAN_POINT ( 'NONE',  ( 95.54126587500000767, 94.81249999863440792, -7.484931351350258973E-15 ) ) ;
#6291=CARTESIAN_POINT ( 'NONE',  ( 93.00000000000000000, 110.0000000000000000, -46.00000000000000711 ) ) ;
#6293=CARTESIAN_POINT ( 'NONE',  ( 108.0825317500000011, 107.3738262389971538, -52.22500000273118559 ) ) ;
#6302=LINE ( 'NONE', #21562, #4789 ) ;
#6313=CARTESIAN_POINT ( 'NONE',  ( 97.83688103937537051, 103.3426043859339103, -49.60000000000000853 ) ) ;
#6330=( GEOMETRIC_REPRESENTATION_CONTEXT ( 3 ) GLOBAL_UNCERTAINTY_ASSIGNED_CONTEXT ( ( #7784 ) ) GLOBAL_UNIT_ASSIGNED_CONTEXT ( ( #5640, #12024, #27441 ) ) REPRESENTATION_CONTEXT ( 'NONE', 'WORKASPACE' ) );
#6332=CARTESIAN_POINT ( 'NONE',  ( 95.67376207875072680, 104.0454443415356991, -49.70000000000000995 ) ) ;
#6335=EDGE_CURVE ( 'NONE', #20101, #7889, #20784, .T. ) ;
#6351=CARTESIAN_POINT ( 'NONE',  ( 99.99999999999998579, 122.5000000021849615, -2.499999999999997780 ) ) ;
#6367=CARTESIAN_POINT ( 'NONE',  ( 93.46109445667491400, 114.7507929638356785, -51.32500000273120122 ) ) ;
#6379=EDGE_CURVE ( 'NONE', #13072, #11653, #16212, .T. ) ;
#6388=( BOUNDED_SURFACE ( )  B_SPLINE_SURFACE ( 1, 2, ( 
 ( #22335, #1104, #9771, #821, #22476, #2940, #18480, #27187, #7199, #24465, #4948, #20334, #13612, #11472, #9489, #19708, #24132, #15561, #10994, #26270, #4608, #13264, #335, #4469, #21721, #15418, #6591, #9023, #26703, #26124, #2195, #6876, #17715, #22138, #24270, #23990, #24409, #7011, #2617, #192, #24557, #13411, #5039, #26559, #2760, #10857, #53, #6732, #4752, #26417, #9297, #8874, #4897, #15707, #21997, #2473, #19568, #19849, #11279, #15272, #22284, #20000, #8733, #480, #13127, #17566, #17426, #13561, #9162, #17993, #21862, #17854, #11423, #20142, #11134, #623, #7152, #15848, #2336, #22853, #18139 ),
 ( #22422, #27275, #20851, #1197, #13984, #20715, #26993, #18287, #20430, #11992, #7588, #9865, #11851, #16135, #13704, #18572, #3181, #14272, #26852, #25118, #16281, #20279, #7730, #20573, #5324, #9583, #3036, #18705, #5463, #15987, #27408, #1332, #913, #24982, #22990, #12125, #11704, #24841, #7299, #3459, #24701, #5605, #1054, #9726, #16421, #14132, #9997, #2893, #11562, #7869, #16564, #22711, #3320, #25255, #18429, #765, #27137, #9438, #5181, #13844, #22568, #7439, #24363, #20097, #24508, #575, #15517, #4996, #23941, #22094, #22235, #429, #6827, #9256, #9114, #17809, #17948, #26512, #21815, #24225, #20234 ) ),
 .UNSPECIFIED., .F., .F., .F. ) 
 B_SPLINE_SURFACE_WITH_KNOTS ( ( 2, 2 ),
 ( 3, 2, 2, 2, 2, 2, 2, 2, 2, 2, 2, 2, 2, 2, 2, 2, 2, 2, 2, 2, 2, 2, 2, 2, 2, 2, 2, 2, 2, 2, 2, 2, 2, 2, 2, 2, 2, 2, 2, 2, 3 ),
 ( 0.000000000000000000, 1.000000000000000000 ),
 ( 0.000000000000000000, 0.02500000000000000139, 0.05000000000000000278, 0.07499999999999999722, 0.1000000000000000056, 0.1250000000000000000, 0.1499999999999999944, 0.1749999999999999889, 0.2000000000000000111, 0.2250000000000000056, 0.2500000000000000000, 0.2750000000000000222, 0.2999999999999999889, 0.3250000000000000111, 0.3499999999999999778, 0.3750000000000000000, 0.4000000000000000222, 0.4249999999999999889, 0.4500000000000000111, 0.4749999999999999778, 0.5000000000000000000, 0.5250000000000000222, 0.5500000000000000444, 0.5749999999999999556, 0.5999999999999999778, 0.6250000000000000000, 0.6500000000000000222, 0.6750000000000000444, 0.6999999999999999556, 0.7249999999999999778, 0.7500000000000000000, 0.7750000000000000222, 0.8000000000000000444, 0.8249999999999999556, 0.8499999999999999778, 0.8750000000000000000, 0.9000000000000000222, 0.9250000000000000444, 0.9499999999999999556, 0.9749999999999999778, 1.000000000000000000 ),
 .UNSPECIFIED. ) 
 GEOMETRIC_REPRESENTATION_ITEM ( )  RATIONAL_B_SPLINE_SURFACE ( (
 ( 1.000000000000000000, 0.9238795325112867385, 1.000000000000000000, 0.9238795325112867385, 1.000000000000000000, 0.9238795325112867385, 1.000000000000000000, 0.9238795325112867385, 1.000000000000000000, 0.9238795325112867385, 1.000000000000000000, 0.9238795325112867385, 1.000000000000000000, 0.9238795325112867385, 1.000000000000000000, 0.9238795325112867385, 1.000000000000000000, 0.9238795325112867385, 1.000000000000000000, 0.9238795325112867385, 1.000000000000000000, 0.9238795325112867385, 1.000000000000000000, 0.9238795325112867385, 1.000000000000000000, 0.9238795325112867385, 1.000000000000000000, 0.9238795325112867385, 1.000000000000000000, 0.9238795325112867385, 1.000000000000000000, 0.9238795325112867385, 1.000000000000000000, 0.9238795325112867385, 1.000000000000000000, 0.9238795325112867385, 1.000000000000000000, 0.9238795325112867385, 1.000000000000000000, 0.9238795325112867385, 1.000000000000000000, 0.9238795325112867385, 1.000000000000000000, 0.9238795325112867385, 1.000000000000000000, 0.9238795325112867385, 1.000000000000000000, 0.9238795325112867385, 1.000000000000000000, 0.9238795325112867385, 1.000000000000000000, 0.9238795325112867385, 1.000000000000000000, 0.9238795325112867385, 1.000000000000000000, 0.9238795325112867385, 1.000000000000000000, 0.9238795325112867385, 1.000000000000000000, 0.9238795325112867385, 1.000000000000000000, 0.9238795325112867385, 1.000000000000000000, 0.9238795325112867385, 1.000000000000000000, 0.9238795325112867385, 1.000000000000000000, 0.9238795325112867385, 1.000000000000000000, 0.9238795325112867385, 1.000000000000000000, 0.9238795325112867385, 1.000000000000000000, 0.9238795325112867385, 1.000000000000000000, 0.9238795325112867385, 1.000000000000000000, 0.9238795325112867385, 1.000000000000000000, 0.9238795325112867385, 1.000000000000000000),
 ( 1.000000000000000000, 0.9238795325112867385, 1.000000000000000000, 0.9238795325112867385, 1.000000000000000000, 0.9238795325112867385, 1.000000000000000000, 0.9238795325112867385, 1.000000000000000000, 0.9238795325112867385, 1.000000000000000000, 0.9238795325112867385, 1.000000000000000000, 0.9238795325112867385, 1.000000000000000000, 0.9238795325112867385, 1.000000000000000000, 0.9238795325112867385, 1.000000000000000000, 0.9238795325112867385, 1.000000000000000000, 0.9238795325112867385, 1.000000000000000000, 0.9238795325112867385, 1.000000000000000000, 0.9238795325112867385, 1.000000000000000000, 0.9238795325112867385, 1.000000000000000000, 0.9238795325112867385, 1.000000000000000000, 0.9238795325112867385, 1.000000000000000000, 0.9238795325112867385, 1.000000000000000000, 0.9238795325112867385, 1.000000000000000000, 0.9238795325112867385, 1.000000000000000000, 0.9238795325112867385, 1.000000000000000000, 0.9238795325112867385, 1.000000000000000000, 0.9238795325112867385, 1.000000000000000000, 0.9238795325112867385, 1.000000000000000000, 0.9238795325112867385, 1.000000000000000000, 0.9238795325112867385, 1.000000000000000000, 0.9238795325112867385, 1.000000000000000000, 0.9238795325112867385, 1.000000000000000000, 0.9238795325112867385, 1.000000000000000000, 0.9238795325112867385, 1.000000000000000000, 0.9238795325112867385, 1.000000000000000000, 0.9238795325112867385, 1.000000000000000000, 0.9238795325112867385, 1.000000000000000000, 0.9238795325112867385, 1.000000000000000000, 0.9238795325112867385, 1.000000000000000000, 0.9238795325112867385, 1.000000000000000000, 0.9238795325112867385, 1.000000000000000000, 0.9238795325112867385, 1.000000000000000000, 0.9238795325112867385, 1.000000000000000000, 0.9238795325112867385, 1.000000000000000000, 0.9238795325112867385, 1.000000000000000000) ) ) 
 REPRESENTATION_ITEM ( '' )  SURFACE ( )  );
#6395=LINE ( 'NONE', #15204, #26184 ) ;
#6399=LINE ( 'NONE', #6668, #28146 ) ;
#6402=AXIS2_PLACEMENT_3D ( 'NONE', #8150, #22854, #16565 ) ;
#6404=DIRECTION ( 'NONE',  ( 1.000000000000000000, 0.000000000000000000, 0.000000000000000000 ) ) ;
#6405=CARTESIAN_POINT ( 'NONE',  ( 96.84719886470463734, 93.93749999863440792, 3.152801135295351997 ) ) ;
#6406=CARTESIAN_POINT ( 'NONE',  ( 95.00000000000000000, 93.37499999726881583, -7.551217303480904118E-15 ) ) ;
#6411=CARTESIAN_POINT ( 'NONE',  ( 101.8468681455907330, 95.12499999863439371, 4.458734124999979898 ) ) ;
#6415=APPLICATION_CONTEXT ( 'automotive_design' ) ;
#6430=CARTESIAN_POINT ( 'NONE',  ( 102.4999999999999858, 123.0000000000000000, -8.724596124144689908E-15 ) ) ;
#6444=DIRECTION ( 'NONE',  ( -0.000000000000000000, 1.000000000000000000, -0.000000000000000000 ) ) ;
#6447=LINE ( 'NONE', #24260, #27017 ) ;
#6450=ORIENTED_EDGE ( 'NONE', *, *, #25620, .T. ) ;
#6451=CARTESIAN_POINT ( 'NONE',  ( 97.83688103937538472, 116.6573956140660897, -50.40000000000000568 ) ) ;
#6453=CARTESIAN_POINT ( 'NONE',  ( 97.93301269999999192, 123.1000000010924822, -0.8561741729129505041 ) ) ;
#6456=CARTESIAN_POINT ( 'NONE',  ( 104.3262379212492590, 104.0454443415356991, -43.80000000546237970 ) ) ;
#6464=( BOUNDED_CURVE ( )  B_SPLINE_CURVE ( 2, ( #4213, #15017, #23738, #12870, #2223, #10887, #10746, #19457, #28155, #26010, #19595 ),
 .UNSPECIFIED., .F., .T. ) 
 B_SPLINE_CURVE_WITH_KNOTS ( ( 3, 2, 2, 2, 2, 3 ),
 ( 0.6999999999999998446, 0.7199999999999998623, 0.7399999999999998801, 0.7600000000000000089, 0.7800000000000000266, 0.8000000000000000444 ),
 .UNSPECIFIED. ) 
 CURVE ( )  GEOMETRIC_REPRESENTATION_ITEM ( )  RATIONAL_B_SPLINE_CURVE ( ( 1.000000000000000222, 0.9510565162951533091, 1.000000000000000000, 0.9510565162951535312, 1.000000000000000000, 0.9510565162951535312, 1.000000000000000000, 0.9510565162951535312, 1.000000000000000000, 0.9510565162951535312, 1.000000000000000000 ) ) 
 REPRESENTATION_ITEM ( '' )  );
#6471=CARTESIAN_POINT ( 'NONE',  ( 104.4587341249999781, 90.31249999863440792, -6.938893903907228378E-15 ) ) ;
#6486=DIRECTION ( 'NONE',  ( -0.000000000000000000, 1.000000000000000000, -0.000000000000000000 ) ) ;
#6489=CARTESIAN_POINT ( 'NONE',  ( 99.99999999999998579, 123.7000000021849502, 2.499999999999978684 ) ) ;
#6494=CARTESIAN_POINT ( 'NONE',  ( 101.4615807364564546, 124.0500000010924850, 1.461580736456455476 ) ) ;
#6501=CARTESIAN_POINT ( 'NONE',  ( 95.00472066334982912, 116.8754121666685393, -49.42500000273118133 ) ) ;
#6510=EDGE_CURVE ( 'NONE', #5706, #7474, #24539, .T. ) ;
#6522=CARTESIAN_POINT ( 'NONE',  ( 101.0355339059327235, 122.9500000021849502, 2.499999999999977796 ) ) ;
#6523=CARTESIAN_POINT ( 'NONE',  ( 99.99999999999998579, 90.00000000000000000, -6.938893903907228378E-15 ) ) ;
#6531=CARTESIAN_POINT ( 'NONE',  ( 108.0825317500000153, 110.0000000000000000, -44.37500000273119838 ) ) ;
#6536=CARTESIAN_POINT ( 'NONE',  ( 96.84719886470463734, 92.93749999863440792, 3.152801135295351997 ) ) ;
#6542=CARTESIAN_POINT ( 'NONE',  ( 103.1528011352953484, 94.43749999863440792, -3.152801135295366208 ) ) ;
#6548=EDGE_LOOP ( 'NONE', ( #22161, #16522, #12528, #3866 ) ) ;
#6567=CARTESIAN_POINT ( 'NONE',  ( 93.46109445667491400, 114.7507929638356785, -49.32500000273120122 ) ) ;
#6568=CARTESIAN_POINT ( 'NONE',  ( 101.0355339059327235, 123.9500000000000028, -2.499999999999996447 ) ) ;
#6574=CARTESIAN_POINT ( 'NONE',  ( 94.33688103937537051, 114.1144967660473242, -50.70000000546238539 ) ) ;
#6577=ADVANCED_FACE ( 'NONE', ( #10483 ), #21615, .F. ) ;
#6583=ORIENTED_EDGE ( 'NONE', *, *, #25568, .F. ) ;
#6584=CARTESIAN_POINT ( 'NONE',  ( 104.3262379212492590, 115.9545556584642867, -48.70000000000000284 ) ) ;
#6591=CARTESIAN_POINT ( 'NONE',  ( 96.46446609406726225, 92.49999999726880162, 3.535533905932723986 ) ) ;
#6606=CARTESIAN_POINT ( 'NONE',  ( 107.0000000000000000, 107.7255621263696241, -49.10000000000000853 ) ) ;
#6622=DIRECTION ( 'NONE',  ( 0.000000000000000000, -1.000000000000000000, 0.000000000000000000 ) ) ;
#6623=ADVANCED_FACE ( 'NONE', ( #2091 ), #9103, .F. ) ;
#6626=CARTESIAN_POINT ( 'NONE',  ( 98.96446609406727646, 124.1500000021849672, -2.499999999999997780 ) ) ;
#6632=CARTESIAN_POINT ( 'NONE',  ( 101.7677669529663547, 123.0000000021849615, 1.767766952966350891 ) ) ;
#6639=CARTESIAN_POINT ( 'NONE',  ( 91.91746824999998466, 107.3738262389971538, -49.02500000273119696 ) ) ;
#6641=CARTESIAN_POINT ( 'NONE',  ( 107.0000000000000142, 110.0000000000000000, -49.00000000000000711 ) ) ;
#6656=FACE_OUTER_BOUND ( 'NONE', #18420, .T. ) ;
#6668=CARTESIAN_POINT ( 'NONE',  ( 105.0000000000000000, 110.0000000000000000, 15.00099999999999412 ) ) ;
#6673=CARTESIAN_POINT ( 'NONE',  ( 96.84719886470463734, 91.68749999863440792, -3.152801135295366208 ) ) ;
#6680=CARTESIAN_POINT ( 'NONE',  ( 104.4587341249999923, 92.24999999863439371, 1.846868145590726318 ) ) ;
#6686=CARTESIAN_POINT ( 'NONE',  ( 95.00000000000000000, 95.43749999726878741, 2.071067811865463959 ) ) ;
#6714=ORIENTED_EDGE ( 'NONE', *, *, #26414, .T. ) ;
#6717=CARTESIAN_POINT ( 'NONE',  ( 114.9999999999999858, 125.0000000000000000, -15.00000000000001066 ) ) ;
#6718=PLANE ( 'NONE',  #17949 ) ;
#6720=ORIENTED_EDGE ( 'NONE', *, *, #802, .T. ) ;
#6725=CARTESIAN_POINT ( 'NONE',  ( 99.99999999999998579, 117.3602355696678501, -50.49999999999999289 ) ) ;
#6727=CARTESIAN_POINT ( 'NONE',  ( 102.0669872999999939, 124.3000000010924566, 0.8561741729129311862 ) ) ;
#6732=CARTESIAN_POINT ( 'NONE',  ( 104.9999999999999716, 93.81249999726880162, 2.071067811865467956 ) ) ;
#6742=CARTESIAN_POINT ( 'NONE',  ( 104.9999999999999716, 94.93750000000000000, 2.071067811865467956 ) ) ;
#6750=AXIS2_PLACEMENT_3D ( 'NONE', #25302, #3926, #3361 ) ;
#6761=ORIENTED_EDGE ( 'NONE', *, *, #10331, .T. ) ;
#6767=CARTESIAN_POINT ( 'NONE',  ( 106.5389055433251002, 114.7507929638356785, -53.92500000273119554 ) ) ;
#6769=CARTESIAN_POINT ( 'NONE',  ( 98.23223304703363112, 122.8000000021849587, 1.767766952966351557 ) ) ;
#6773=CARTESIAN_POINT ( 'NONE',  ( 99.99999999999998579, 123.3000000021849587, -2.499999999999997780 ) ) ;
#6781=CARTESIAN_POINT ( 'NONE',  ( 95.00472066334982912, 116.8754121666685393, -53.42500000273118843 ) ) ;
#6802=CARTESIAN_POINT ( 'NONE',  ( 84.99999999999998579, 100.0000000000000000, -15.00000000000000533 ) ) ;
#6812=LINE ( 'NONE', #23928, #12188 ) ;
#6816=CARTESIAN_POINT ( 'NONE',  ( 100.1038569895340657, 123.0000000000000284, 2.502009621290390839 ) ) ;
#6821=ORIENTED_EDGE ( 'NONE', *, *, #21889, .F. ) ;
#6823=AXIS2_PLACEMENT_3D ( 'NONE', #28141, #1647, #19163 ) ;
#6826=CARTESIAN_POINT ( 'NONE',  ( 95.54126587500000767, 92.81249999863440792, -7.484931351350258973E-15 ) ) ;
#6827=CARTESIAN_POINT ( 'NONE',  ( 95.54126587500000767, 95.06249999863440792, -7.484931351350258973E-15 ) ) ;
#6841=VECTOR ( 'NONE', #17538, 1000.000000000000000 ) ;
#6849=CARTESIAN_POINT ( 'NONE',  ( 105.6631189606246295, 114.1144967660473242, -53.30000000546237970 ) ) ;
#6860=CIRCLE ( 'NONE', #15974, 9.000000000000007105 ) ;
#6864=CARTESIAN_POINT ( 'NONE',  ( 100.0000000000000000, 110.0000000000000000, -55.00000000000000711 ) ) ;
#6869=CARTESIAN_POINT ( 'NONE',  ( 107.0000000000000142, 112.2744378736303332, -46.90000000000001279 ) ) ;
#6876=CARTESIAN_POINT ( 'NONE',  ( 104.9999999999999716, 92.81249999726880162, 2.071067811865467956 ) ) ;
#6882=ORIENTED_EDGE ( 'NONE', *, *, #1003, .F. ) ;
#6891=CARTESIAN_POINT ( 'NONE',  ( 103.1528011352953484, 90.68749999863440792, -3.152801135295366208 ) ) ;
#6897=VERTEX_POINT ( 'NONE', #25437 ) ;
#6906=CARTESIAN_POINT ( 'NONE',  ( 95.00472066334981491, 116.8754121666685393, -53.42500000273118843 ) ) ;
#6909=DIRECTION ( 'NONE',  ( 0.000000000000000000, 0.000000000000000000, 1.000000000000000000 ) ) ;
#6912=ORIENTED_EDGE ( 'NONE', *, *, #23294, .F. ) ;
#6913=CARTESIAN_POINT ( 'NONE',  ( 100.8561741729129153, 123.5000000010924737, -2.066987299999999195 ) ) ;
#6920=CARTESIAN_POINT ( 'NONE',  ( 108.0825317500000153, 110.0000000000000000, -52.12500000273119838 ) ) ;
#6926=VECTOR ( 'NONE', #27375, 1000.000000000000114 ) ;
#6944=AXIS2_PLACEMENT_3D ( 'NONE', #5550, #7377, #704 ) ;
#6954=CARTESIAN_POINT ( 'NONE',  ( 99.99999999999998579, 101.5015231886685712, -46.87500000273119838 ) ) ;
#6958=CARTESIAN_POINT ( 'NONE',  ( 100.3882422504498493, 123.0000000000000000, 2.474292135181528351 ) ) ;
#6967=CARTESIAN_POINT ( 'NONE',  ( 103.1528011352953484, 94.18749999863440792, 3.152801135295352886 ) ) ;
#6981=EDGE_LOOP ( 'NONE', ( #25937, #23499, #17064, #16760 ) ) ;
#6991=CARTESIAN_POINT ( 'NONE',  ( 108.0825317500000153, 110.0000000000000000, -44.12500000273119127 ) ) ;
#6992=DIRECTION ( 'NONE',  ( 1.000000000000000000, 0.000000000000000000, 0.000000000000000000 ) ) ;
#6993=LINE ( 'NONE', #15540, #16637 ) ;
#7002=VERTEX_POINT ( 'NONE', #15248 ) ;
#7006=CARTESIAN_POINT ( 'NONE',  ( 97.50236033167492167, 102.3130555110000159, -52.97500000273119980 ) ) ;
#7008=CARTESIAN_POINT ( 'NONE',  ( 102.4999999999999716, 124.5500000000000114, 1.035533905932722876 ) ) ;
#7011=CARTESIAN_POINT ( 'NONE',  ( 97.92893218813452449, 93.18749999726878741, -4.999999999999997335 ) ) ;
#7014=CARTESIAN_POINT ( 'NONE',  ( 102.4976396683250925, 117.6869444889999841, -51.97500000273119980 ) ) ;
#7018=ORIENTED_EDGE ( 'NONE', *, *, #26568, .T. ) ;
#7022=FACE_OUTER_BOUND ( 'NONE', #16990, .T. ) ;
#7027=ORIENTED_EDGE ( 'NONE', *, *, #16450, .T. ) ;
#7041=EDGE_CURVE ( 'NONE', #8293, #27581, #18710, .T. ) ;
#7048=CARTESIAN_POINT ( 'NONE',  ( 98.23223304703363112, 122.8000000021849587, 1.767766952966351557 ) ) ;
#7056=CARTESIAN_POINT ( 'NONE',  ( 91.91746824999998466, 107.3738262389971538, -45.02500000273118985 ) ) ;
#7060=CARTESIAN_POINT ( 'NONE',  ( 102.1631189606246295, 116.6573956140660897, -49.10000000546237686 ) ) ;
#7065=EDGE_CURVE ( 'NONE', #19120, #19945, #15539, .T. ) ;
#7066=ORIENTED_EDGE ( 'NONE', *, *, #1945, .T. ) ;
#7074=FACE_OUTER_BOUND ( 'NONE', #14902, .T. ) ;
#7092=CARTESIAN_POINT ( 'NONE',  ( 99.99999999999998579, 110.0000000000000000, -45.00000000000000711 ) ) ;
#7096=CARTESIAN_POINT ( 'NONE',  ( 93.46109445667491400, 105.2492070361643215, -53.17500000273119554 ) ) ;
#7097=CARTESIAN_POINT ( 'NONE',  ( 98.69444032418647339, 123.0000000000000426, -2.137373984154804063 ) ) ;
#7098=CARTESIAN_POINT ( 'NONE',  ( 102.0669872999999939, 123.3000000010924850, 0.8561741729129311862 ) ) ;
#7106=CARTESIAN_POINT ( 'NONE',  ( 102.0710678118654613, 92.81249999999998579, 4.999999999999983125 ) ) ;
#7112=ORIENTED_EDGE ( 'NONE', *, *, #25532, .T. ) ;
#7121=DIRECTION ( 'NONE',  ( 1.000000000000000000, 0.000000000000000000, 0.000000000000000000 ) ) ;
#7129=CARTESIAN_POINT ( 'NONE',  ( 91.91746824999998466, 112.6261737610028320, -47.22500000273119269 ) ) ;
#7130=CARTESIAN_POINT ( 'NONE',  ( 96.84719886470463734, 91.93749999863440792, -3.152801135295366208 ) ) ;
#7134=VERTEX_POINT ( 'NONE', #4167 ) ;
#7137=CARTESIAN_POINT ( 'NONE',  ( 99.99999999999998579, 91.75000000000000000, 4.999999999999984013 ) ) ;
#7146=CARTESIAN_POINT ( 'NONE',  ( 99.99999999999998579, 102.6397644303321215, -45.50000000000000000 ) ) ;
#7152=CARTESIAN_POINT ( 'NONE',  ( 99.99999999999998579, 95.62499999726881583, 4.999999999999984013 ) ) ;
#7155=CARTESIAN_POINT ( 'NONE',  ( 99.99999999999998579, 101.5015231886685712, -48.87500000273119838 ) ) ;
#7165=CARTESIAN_POINT ( 'NONE',  ( 99.99999999999998579, 91.81249999863440792, -4.458734124999994997 ) ) ;
#7177=CARTESIAN_POINT ( 'NONE',  ( 95.00000000000000000, 91.43749999726880162, 2.071067811865463959 ) ) ;
#7178=DIRECTION ( 'NONE',  ( -5.782411586589357392E-17, -0.000000000000000000, -1.000000000000000000 ) ) ;
#7180=CARTESIAN_POINT ( 'NONE',  ( 93.46109445667491400, 105.2492070361643215, -46.92500000273119554 ) ) ;
#7182=CARTESIAN_POINT ( 'NONE',  ( 99.99999999999998579, 89.99899999999999523, -2.500000000000004885 ) ) ;
#7185=ORIENTED_EDGE ( 'NONE', *, *, #19222, .T. ) ;
#7193=CARTESIAN_POINT ( 'NONE',  ( 95.54126587500000767, 93.81249999863440792, -7.484931351350258973E-15 ) ) ;
#7195=CARTESIAN_POINT ( 'NONE',  ( 102.4976396683250925, 102.3130555110000159, -46.52500000273119696 ) ) ;
#7197=CARTESIAN_POINT ( 'NONE',  ( 97.50000000000000000, 124.6500000010924651, -9.540979117872439019E-15 ) ) ;
#7199=CARTESIAN_POINT ( 'NONE',  ( 95.00000000000000000, 91.37499999726880162, -7.551217303480904118E-15 ) ) ;
#7208=EDGE_CURVE ( 'NONE', #613, #2910, #27676, .T. ) ;
#7221=CARTESIAN_POINT ( 'NONE',  ( 97.50000000000000000, 124.2569999999781487, 1.035533905932725096 ) ) ;
#7222=ADVANCED_FACE ( 'NONE', ( #20257 ), #18406, .F. ) ;
#7236=CARTESIAN_POINT ( 'NONE',  ( 106.5389055433251002, 114.7507929638356785, -52.17500000273119554 ) ) ;
#7237=CARTESIAN_POINT ( 'NONE',  ( 97.70296704779451602, 123.0000000000000000, 0.9970373613995330286 ) ) ;
#7239=CARTESIAN_POINT ( 'NONE',  ( 102.0669872999999797, 123.3500000010924680, -9.794112055954760458E-15 ) ) ;
#7248=CARTESIAN_POINT ( 'NONE',  ( 96.46446609406726225, 92.62500000000000000, 3.535533905932723986 ) ) ;
#7254=ORIENTED_EDGE ( 'NONE', *, *, #2702, .F. ) ;
#7256=ADVANCED_FACE ( 'NONE', ( #24533 ), #20015, .T. ) ;
#7258=ORIENTED_EDGE ( 'NONE', *, *, #26612, .T. ) ;
#7266=FACE_OUTER_BOUND ( 'NONE', #1004, .T. ) ;
#7268=CARTESIAN_POINT ( 'NONE',  ( 104.9999999999999716, 91.93749999999998579, 2.071067811865467956 ) ) ;
#7274=CARTESIAN_POINT ( 'NONE',  ( 95.67376207875072680, 104.0454443415356991, -52.20000000546237828 ) ) ;
#7291=CARTESIAN_POINT ( 'NONE',  ( 104.9952793366501851, 103.1245878333314323, -50.67500000273119554 ) ) ;
#7294=CYLINDRICAL_SURFACE ( 'NONE', #16697, 7.000000000000006217 ) ;
#7299=CARTESIAN_POINT ( 'NONE',  ( 96.84719886470463734, 92.93749999863440792, -3.152801135295366208 ) ) ;
#7302=CARTESIAN_POINT ( 'NONE',  ( 91.91746824999998466, 112.6261737610028320, -51.47500000273119980 ) ) ;
#7308=LINE ( 'NONE', #9308, #25628 ) ;
#7313=CARTESIAN_POINT ( 'NONE',  ( 95.54126587499999346, 91.99999999863439371, -1.846868145590737864 ) ) ;
#7327=AXIS2_PLACEMENT_3D ( 'NONE', #8384, #21648, #15062 ) ;
#7329=CARTESIAN_POINT ( 'NONE',  ( 99.99999999999998579, 118.4984768113314146, -47.62500000273119127 ) ) ;
#7330=DIRECTION ( 'NONE',  ( -0.000000000000000000, -0.000000000000000000, -1.000000000000000000 ) ) ;
#7340=CARTESIAN_POINT ( 'NONE',  ( 102.0710678118655039, 94.68749999726880162, 4.999999999999940492 ) ) ;
#7348=ORIENTED_EDGE ( 'NONE', *, *, #25688, .F. ) ;
#7349=VERTEX_POINT ( 'NONE', #20614 ) ;
#7359=CARTESIAN_POINT ( 'NONE',  ( 101.7677669529663547, 124.0000000021849615, -1.767766952966370209 ) ) ;
#7364=CARTESIAN_POINT ( 'NONE',  ( 97.50000000000000000, 124.1569999999781544, -1.035533905932742416 ) ) ;
#7368=CARTESIAN_POINT ( 'NONE',  ( 102.0669872999999797, 122.5500000010924850, -9.794112055954760458E-15 ) ) ;
#7377=DIRECTION ( 'NONE',  ( 0.000000000000000000, 1.000000000000000000, 0.000000000000000000 ) ) ;
#7380=CARTESIAN_POINT ( 'NONE',  ( 97.92893218813452449, 90.68750000000000000, 4.999999999999991118 ) ) ;
#7381=CARTESIAN_POINT ( 'NONE',  ( 98.24352329449848753, 123.0000000000000426, -1.784664002384159565 ) ) ;
#7385=ORIENTED_EDGE ( 'NONE', *, *, #5869, .T. ) ;
#7389=CARTESIAN_POINT ( 'NONE',  ( 102.0710678118654613, 92.18749999999998579, -4.999999999999997335 ) ) ;
#7395=ORIENTED_EDGE ( 'NONE', *, *, #6004, .T. ) ;
#7397=VECTOR ( 'NONE', #15069, 1000.000000000000000 ) ;
#7399=ORIENTED_EDGE ( 'NONE', *, *, #5935, .F. ) ;
#7407=CYLINDRICAL_SURFACE ( 'NONE', #2685, 7.000000000000006217 ) ;
#7408=CARTESIAN_POINT ( 'NONE',  ( 103.1528011352953484, 91.18749999863440792, 3.152801135295352886 ) ) ;
#7415=CARTESIAN_POINT ( 'NONE',  ( 108.0825317500000011, 107.3738262389971538, -48.22500000273118559 ) ) ;
#7416=CARTESIAN_POINT ( 'NONE',  ( 101.8468681455907330, 91.74999999863439371, -4.458734124999994997 ) ) ;
#7421=EDGE_LOOP ( 'NONE', ( #7757, #22225, #341 ) ) ;
#7425=EDGE_CURVE ( 'NONE', #26599, #19519, #27462, .T. ) ;
#7427=ORIENTED_EDGE ( 'NONE', *, *, #476, .F. ) ;
#7431=CARTESIAN_POINT ( 'NONE',  ( 93.46109445667491400, 114.7507929638356785, -53.57500000273119412 ) ) ;
#7439=CARTESIAN_POINT ( 'NONE',  ( 101.8468681455907330, 94.37499999863440792, 4.458734124999979898 ) ) ;
#7441=CARTESIAN_POINT ( 'NONE',  ( 108.0825317500000011, 112.6261737610028320, -48.27500000273119696 ) ) ;
#7442=ORIENTED_EDGE ( 'NONE', *, *, #16267, .F. ) ;
#7449=ADVANCED_FACE ( 'NONE', ( #955 ), #7633, .F. ) ;
#7454=CARTESIAN_POINT ( 'NONE',  ( 98.15313185440923860, 92.24999999863439371, 4.458734124999980786 ) ) ;
#7463=LINE ( 'NONE', #1220, #9148 ) ;
#7467=DIRECTION ( 'NONE',  ( -1.000000000000000000, 0.000000000000000000, 0.000000000000000000 ) ) ;
#7470=CARTESIAN_POINT ( 'NONE',  ( 95.00472066334981491, 116.8754121666685393, -45.42500000273118843 ) ) ;
#7474=VERTEX_POINT ( 'NONE', #4199 ) ;
#7475=ORIENTED_EDGE ( 'NONE', *, *, #8912, .F. ) ;
#7485=CARTESIAN_POINT ( 'NONE',  ( 106.5389055433251002, 105.2492070361643215, -48.32500000273119412 ) ) ;
#7487=VECTOR ( 'NONE', #15972, 1000.000000000000000 ) ;
#7505=CARTESIAN_POINT ( 'NONE',  ( 93.00000000000000000, 110.0000000000000000, -48.00000000000000711 ) ) ;
#7507=VECTOR ( 'NONE', #11874, 999.9999999999998863 ) ;
#7511=CARTESIAN_POINT ( 'NONE',  ( 99.99999999999998579, 124.8069999999781459, -2.499999999999997780 ) ) ;
#7528=CARTESIAN_POINT ( 'NONE',  ( 97.93301270000000613, 124.5500000010924850, -9.540979117872439019E-15 ) ) ;
#7532=EDGE_LOOP ( 'NONE', ( #16291, #16269, #18731, #1759 ) ) ;
#7537=CARTESIAN_POINT ( 'NONE',  ( 95.00000000000000000, 91.43750000000001421, -2.071067811865479058 ) ) ;
#7543=ORIENTED_EDGE ( 'NONE', *, *, #25688, .T. ) ;
#7547=VERTEX_POINT ( 'NONE', #19442 ) ;
#7555=CARTESIAN_POINT ( 'NONE',  ( 95.54126587499999346, 92.74999999863439371, -1.846868145590737864 ) ) ;
#7560=CARTESIAN_POINT ( 'NONE',  ( 98.23223304703363112, 123.5000000000000000, 1.767766952966351557 ) ) ;
#7562=CARTESIAN_POINT ( 'NONE',  ( 99.99999999999998579, 117.3602355696678501, -51.00000000546238255 ) ) ;
#7563=CARTESIAN_POINT ( 'NONE',  ( 95.54126587499999346, 90.99999999863439371, -1.846868145590737864 ) ) ;
#7569=EDGE_CURVE ( 'NONE', #15184, #12415, #12240, .T. ) ;
#7579=CARTESIAN_POINT ( 'NONE',  ( 97.50236033167492167, 117.6869444889999841, -45.77500000273119696 ) ) ;
#7581=AXIS2_PLACEMENT_3D ( 'NONE', #1805, #3798, #15021 ) ;
#7584=EDGE_CURVE ( 'NONE', #10198, #12623, #23162, .T. ) ;
#7588=CARTESIAN_POINT ( 'NONE',  ( 96.84719886470463734, 91.18749999863440792, 3.152801135295351997 ) ) ;
#7589=CARTESIAN_POINT ( 'NONE',  ( 99.99999999999998579, 90.00000000000000000, -6.938893903907228378E-15 ) ) ;
#7590=CARTESIAN_POINT ( 'NONE',  ( 91.91746824999999887, 110.0000000000000000, -51.37500000273119127 ) ) ;
#7599=FACE_OUTER_BOUND ( 'NONE', #182, .T. ) ;
#7600=LINE ( 'NONE', #10006, #602 ) ;
#7605=CARTESIAN_POINT ( 'NONE',  ( 95.54126587499999346, 94.12499999863439371, 1.846868145590722543 ) ) ;
#7612=CARTESIAN_POINT ( 'NONE',  ( 99.99999999999998579, 90.00000000000000000, -2.999999999999996447 ) ) ;
#7618=EDGE_CURVE ( 'NONE', #8183, #21036, #1760, .T. ) ;
#7624=CARTESIAN_POINT ( 'NONE',  ( 93.00000000000000000, 112.2744378736303190, -44.60000000546238397 ) ) ;
#7625=CARTESIAN_POINT ( 'NONE',  ( 84.99999999999998579, 125.0000000000000000, 14.99999999999999112 ) ) ;
#7633=CYLINDRICAL_SURFACE ( 'NONE', #4995, 7.000000000000006217 ) ;
#7634=CARTESIAN_POINT ( 'NONE',  ( 95.00472066334982912, 103.1245878333314323, -44.82500000273117990 ) ) ;
#7638=FACE_OUTER_BOUND ( 'NONE', #12884, .T. ) ;
#7642=CARTESIAN_POINT ( 'NONE',  ( 112.9999999999999858, 97.00000000000000000, 14.99999999999999467 ) ) ;
#7661=CARTESIAN_POINT ( 'NONE',  ( 102.1631189606246295, 103.3426043859339103, -47.40000000000000568 ) ) ;
#7663=FACE_OUTER_BOUND ( 'NONE', #6981, .T. ) ;
#7672=FACE_OUTER_BOUND ( 'NONE', #20318, .T. ) ;
#7674=CARTESIAN_POINT ( 'NONE',  ( 99.14382582708707048, 124.4000000010924794, -2.066987299999999195 ) ) ;
#7678=ORIENTED_EDGE ( 'NONE', *, *, #14071, .T. ) ;
#7682=CARTESIAN_POINT ( 'NONE',  ( 95.00000000000000000, 92.56250000000000000, 2.071067811865463959 ) ) ;
#7684=VECTOR ( 'NONE', #12120, 1000.000000000000000 ) ;
#7687=VECTOR ( 'NONE', #10929, 1000.000000000000000 ) ;
#7692=( BOUNDED_CURVE ( )  B_SPLINE_CURVE ( 2, ( #15810, #19666, #723, #2720, #11096, #6686, #17953, #9396, #4710 ),
 .UNSPECIFIED., .F., .T. ) 
 B_SPLINE_CURVE_WITH_KNOTS ( ( 3, 2, 2, 2, 3 ),
 ( 0.8500000000000007550, 0.8750000000000008882, 0.9000000000000009104, 0.9250000000000009326, 0.9500000000000009548 ),
 .UNSPECIFIED. ) 
 CURVE ( )  GEOMETRIC_REPRESENTATION_ITEM ( )  RATIONAL_B_SPLINE_CURVE ( ( 0.9999999999999976685, 0.9238795325112890700, 1.000000000000000000, 0.9238795325112867385, 1.000000000000000000, 0.9238795325112867385, 1.000000000000000000, 0.9238795325112837409, 1.000000000000003109 ) ) 
 REPRESENTATION_ITEM ( '' )  );
#7708=CARTESIAN_POINT ( 'NONE',  ( 97.83688103937537051, 103.3426043859339103, -48.10000000546237686 ) ) ;
#7709=MECHANICAL_DESIGN_GEOMETRIC_PRESENTATION_REPRESENTATION('',(#14962),#6330);
#7710=CARTESIAN_POINT ( 'NONE',  ( 101.8468681455907330, 95.37499999863440792, 4.458734124999979898 ) ) ;
#7723=CARTESIAN_POINT ( 'NONE',  ( 97.50236033167492167, 102.3130555110000159, -46.97500000273119269 ) ) ;
#7727=VECTOR ( 'NONE', #11053, 1000.000000000000000 ) ;
#7730=CARTESIAN_POINT ( 'NONE',  ( 96.84719886470463734, 91.93749999863440792, -3.152801135295366208 ) ) ;
#7745=CARTESIAN_POINT ( 'NONE',  ( 95.54126587500000767, 95.06249999863440792, -7.484931351350258973E-15 ) ) ;
#7748=VECTOR ( 'NONE', #12727, 1000.000000000000000 ) ;
#7752=DIRECTION ( 'NONE',  ( -1.000000000000000000, 0.000000000000000000, 0.000000000000000000 ) ) ;
#7757=ORIENTED_EDGE ( 'NONE', *, *, #446, .T. ) ;
#7759=AXIS2_PLACEMENT_3D ( 'NONE', #6802, #15487, #13342 ) ;
#7764=DIRECTION ( 'NONE',  ( 0.000000000000000000, 1.000000000000000000, -1.156482317317871478E-16 ) ) ;
#7766=ADVANCED_FACE ( 'NONE', ( #2177 ), #4453, .T. ) ;
#7771=CARTESIAN_POINT ( 'NONE',  ( 104.9999999999999858, 91.00000000000000000, -6.938893903907228378E-15 ) ) ;
#7781=EDGE_CURVE ( 'NONE', #20441, #14776, #26768, .T. ) ;
#7784=UNCERTAINTY_MEASURE_WITH_UNIT (LENGTH_MEASURE( 1.000000000000000082E-05 ), #5640, 'distance_accuracy_value', 'NONE');
#7791=ORIENTED_EDGE ( 'NONE', *, *, #11098, .T. ) ;
#7800=CARTESIAN_POINT ( 'NONE',  ( 102.4999999999999858, 122.9813376334432604, 0.3865102666887284544 ) ) ;
#7815=CARTESIAN_POINT ( 'NONE',  ( 91.91746824999999887, 110.0000000000000000, -51.37500000273119127 ) ) ;
#7822=VERTEX_POINT ( 'NONE', #26401 ) ;
#7844=DIRECTION ( 'NONE',  ( -5.782411586589357392E-17, 0.000000000000000000, -1.000000000000000000 ) ) ;
#7846=CARTESIAN_POINT ( 'NONE',  ( 93.00000000000000000, 110.0000000000000000, -52.50000000546237544 ) ) ;
#7848=CARTESIAN_POINT ( 'NONE',  ( 97.83688103937538472, 116.6573956140660897, -50.90000000546238113 ) ) ;
#7849=CARTESIAN_POINT ( 'NONE',  ( 104.4587341249999923, 93.62499999863440792, -1.846868145590737198 ) ) ;
#7851=CARTESIAN_POINT ( 'NONE',  ( 102.3556624333333076, 122.3833333351541199, -9.829464563757769835E-15 ) ) ;
#7855=CARTESIAN_POINT ( 'NONE',  ( 99.99999999999998579, 90.56249999863440792, -4.458734124999994997 ) ) ;
#7863=CARTESIAN_POINT ( 'NONE',  ( 97.50236033167492167, 102.3130555110000159, -48.97500000273119269 ) ) ;
#7869=CARTESIAN_POINT ( 'NONE',  ( 104.4587341249999923, 93.62499999863440792, -1.846868145590737198 ) ) ;
#7882=CARTESIAN_POINT ( 'NONE',  ( 96.84719886470463734, 94.93749999863440792, -3.152801135295366208 ) ) ;
#7889=VERTEX_POINT ( 'NONE', #2875 ) ;
#7899=CARTESIAN_POINT ( 'NONE',  ( 93.00000000000000000, 110.0000000000000000, -44.50000000546237544 ) ) ;
#7913=CARTESIAN_POINT ( 'NONE',  ( 103.5355339059327235, 93.74999999726881583, 3.535533905932724874 ) ) ;
#7932=CARTESIAN_POINT ( 'NONE',  ( 102.4999999999999716, 124.5500000000000114, 1.035533905932722876 ) ) ;
#7939=DIRECTION ( 'NONE',  ( 0.000000000000000000, 1.000000000000000000, 0.000000000000000000 ) ) ;
#7948=CARTESIAN_POINT ( 'NONE',  ( 108.0825317500000153, 110.0000000000000000, -48.37500000273119838 ) ) ;
#7949=DIRECTION ( 'NONE',  ( -0.000000000000000000, 1.000000000000000000, -0.000000000000000000 ) ) ;
#7950=CARTESIAN_POINT ( 'NONE',  ( 97.93301269999999192, 123.1000000010924822, -0.8561741729129505041 ) ) ;
#7955=DIRECTION ( 'NONE',  ( 0.000000000000000000, -0.000000000000000000, -1.000000000000000000 ) ) ;
#7968=EDGE_CURVE ( 'NONE', #1889, #13215, #22695, .T. ) ;
#7972=CARTESIAN_POINT ( 'NONE',  ( 101.8468681455907330, 94.12499999863439371, 4.458734124999980786 ) ) ;
#7981=CARTESIAN_POINT ( 'NONE',  ( 105.6631189606246295, 114.1144967660473242, -47.30000000546237260 ) ) ;
#7982=CARTESIAN_POINT ( 'NONE',  ( 98.15313185440925281, 93.24999999863439371, 4.458734124999979898 ) ) ;
#7990=CARTESIAN_POINT ( 'NONE',  ( 104.4587341249999781, 91.31249999863440792, -6.938893903907228378E-15 ) ) ;
#7992=ORIENTED_EDGE ( 'NONE', *, *, #3475, .F. ) ;
#7996=CARTESIAN_POINT ( 'NONE',  ( 99.99999999999998579, 118.4984768113314004, -47.87500000273119127 ) ) ;
#8000=CARTESIAN_POINT ( 'NONE',  ( 91.91746824999999887, 110.0000000000000000, -47.12500000273119838 ) ) ;
#8014=CARTESIAN_POINT ( 'NONE',  ( 84.99999999999998579, 100.0000000000000000, -15.00000000000000533 ) ) ;
#8031=CARTESIAN_POINT ( 'NONE',  ( 94.33688103937537051, 114.1144967660473242, -54.20000000000000284 ) ) ;
#8036=CARTESIAN_POINT ( 'NONE',  ( 84.99999999999998579, 120.0000000000000000, -15.00000000000000533 ) ) ;
#8049=CARTESIAN_POINT ( 'NONE',  ( 93.00000000000002842, 112.2744378736303759, -48.60000000546236976 ) ) ;
#8064=CARTESIAN_POINT ( 'NONE',  ( 102.1631189606246295, 116.6573956140660897, -48.60000000000000142 ) ) ;
#8069=CARTESIAN_POINT ( 'NONE',  ( 97.50000000000000000, 124.1499999999999915, -1.035533905932742416 ) ) ;
#8071=CARTESIAN_POINT ( 'NONE',  ( 97.93301270000000613, 123.9000000010924794, -0.8561741729129506151 ) ) ;
#8077=CARTESIAN_POINT ( 'NONE',  ( 101.7677669529663547, 123.8000000021849587, 1.767766952966350891 ) ) ;
#8085=CARTESIAN_POINT ( 'NONE',  ( 99.99999999999998579, 101.5015231886685854, -46.87500000273119838 ) ) ;
#8088=CARTESIAN_POINT ( 'NONE',  ( 99.14382582708707048, 124.6000000010924822, -2.066987299999999195 ) ) ;
#8105=CARTESIAN_POINT ( 'NONE',  ( 107.0000000000000142, 112.2744378736303048, -47.40000000546237402 ) ) ;
#8112=CARTESIAN_POINT ( 'NONE',  ( 104.4587341249999923, 93.24999999863439371, 1.846868145590726318 ) ) ;
#8122=CARTESIAN_POINT ( 'NONE',  ( 95.67376207875072680, 115.9545556584642867, -50.80000000546237260 ) ) ;
#8123=CARTESIAN_POINT ( 'NONE',  ( 103.1528011352953484, 90.43749999863440792, -3.152801135295366208 ) ) ;
#8127=VERTEX_POINT ( 'NONE', #24787 ) ;
#8133=EDGE_CURVE ( 'NONE', #1383, #25390, #1463, .T. ) ;
#8138=ORIENTED_EDGE ( 'NONE', *, *, #19222, .F. ) ;
#8139=CARTESIAN_POINT ( 'NONE',  ( 106.5389055433251002, 114.7507929638356785, -50.17500000273119554 ) ) ;
#8143=CARTESIAN_POINT ( 'NONE',  ( 97.50236033167492167, 102.3130555110000159, -50.72500000273119980 ) ) ;
#8150=CARTESIAN_POINT ( 'NONE',  ( 99.99999999999998579, 90.00000000000000000, -6.938893903907228378E-15 ) ) ;
#8159=DIRECTION ( 'NONE',  ( 5.782411586589357392E-17, -0.000000000000000000, 1.000000000000000000 ) ) ;
#8160=ORIENTED_EDGE ( 'NONE', *, *, #11572, .T. ) ;
#8162=CARTESIAN_POINT ( 'NONE',  ( 99.99999999999998579, 123.5500000010924850, -2.066987299999998751 ) ) ;
#8163=CARTESIAN_POINT ( 'NONE',  ( 95.54126587499999346, 95.12499999863439371, 1.846868145590722543 ) ) ;
#8168=VERTEX_POINT ( 'NONE', #25072 ) ;
#8176=AXIS2_PLACEMENT_3D ( 'NONE', #27930, #10102, #25229 ) ;
#8183=VERTEX_POINT ( 'NONE', #16919 ) ;
#8189=LINE ( 'NONE', #8608, #7748 ) ;
#8209=CARTESIAN_POINT ( 'NONE',  ( 97.50000000000000000, 123.4069999999781402, -9.540979117872439019E-15 ) ) ;
#8211=CARTESIAN_POINT ( 'NONE',  ( 98.53841926354351699, 124.6500000010924651, -1.461580736456474794 ) ) ;
#8222=CARTESIAN_POINT ( 'NONE',  ( 93.46109445667491400, 114.7507929638356785, -45.57500000273119412 ) ) ;
#8224=CARTESIAN_POINT ( 'NONE',  ( 101.4615807364564546, 122.8500000010924680, -1.461580736456474794 ) ) ;
#8228=EDGE_LOOP ( 'NONE', ( #16188, #23958, #18976, #4951 ) ) ;
#8232=CARTESIAN_POINT ( 'NONE',  ( 96.46446609406726225, 94.62500000000000000, 3.535533905932723986 ) ) ;
#8234=AXIS2_PLACEMENT_3D ( 'NONE', #5606, #24983, #18430 ) ;
#8235=CARTESIAN_POINT ( 'NONE',  ( 93.00000000000000000, 110.0000000000000000, -55.00000000000000711 ) ) ;
#8239=CARTESIAN_POINT ( 'NONE',  ( 97.83688103937538472, 116.6573956140660897, -46.90000000546238113 ) ) ;
#8247=CARTESIAN_POINT ( 'NONE',  ( 99.99999999999998579, 93.06249999863440792, 4.458734124999981674 ) ) ;
#8257=CARTESIAN_POINT ( 'NONE',  ( 104.4587341249999781, 93.56249999863440792, -6.938893903907228378E-15 ) ) ;
#8258=DIRECTION ( 'NONE',  ( 0.000000000000000000, -1.000000000000000000, 0.000000000000000000 ) ) ;
#8264=CARTESIAN_POINT ( 'NONE',  ( 96.84719886470463734, 91.68749999863440792, -3.152801135295366208 ) ) ;
#8265=ORIENTED_EDGE ( 'NONE', *, *, #17331, .T. ) ;
#8269=FACE_OUTER_BOUND ( 'NONE', #2850, .T. ) ;
#8276=CARTESIAN_POINT ( 'NONE',  ( 84.99999999999998579, 120.0000000000000000, -45.00000000000000711 ) ) ;
#8280=ORIENTED_EDGE ( 'NONE', *, *, #22594, .T. ) ;
#8283=EDGE_CURVE ( 'NONE', #15184, #3280, #17621, .T. ) ;
#8286=FACE_OUTER_BOUND ( 'NONE', #13254, .T. ) ;
#8293=VERTEX_POINT ( 'NONE', #26328 ) ;
#8296=CARTESIAN_POINT ( 'NONE',  ( 104.7293670624999748, 90.15624999931721106, -6.938893903907228378E-15 ) ) ;
#8301=EDGE_LOOP ( 'NONE', ( #23669, #19242, #5304, #12669 ) ) ;
#8306=CARTESIAN_POINT ( 'NONE',  ( 93.00000000000000000, 110.0000000000000000, -48.00000000000000711 ) ) ;
#8308=CARTESIAN_POINT ( 'NONE',  ( 104.9999999999999716, 92.93749999726880162, -2.071067811865478170 ) ) ;
#8313=EDGE_CURVE ( 'NONE', #10673, #9430, #23903, .T. ) ;
#8322=CARTESIAN_POINT ( 'NONE',  ( 97.92893218813451028, 92.18749999726878741, -4.999999999999984013 ) ) ;
#8324=CARTESIAN_POINT ( 'NONE',  ( 100.0000000000000000, 110.0000000000000000, -45.00000000000000711 ) ) ;
#8326=CARTESIAN_POINT ( 'NONE',  ( 112.9999999999999858, 123.0000000000000000, 14.99999999999999112 ) ) ;
#8332=UNCERTAINTY_MEASURE_WITH_UNIT (LENGTH_MEASURE( 1.000000000000000082E-05 ), #17603, 'distance_accuracy_value', 'NONE');
#8343=CARTESIAN_POINT ( 'NONE',  ( 97.50000000000000000, 124.9500000000000028, -1.035533905932742416 ) ) ;
#8347=CARTESIAN_POINT ( 'NONE',  ( 101.7677669529663547, 123.8999999999999915, -1.767766952966370209 ) ) ;
#8350=VECTOR ( 'NONE', #5212, 1000.000000000000000 ) ;
#8352=CARTESIAN_POINT ( 'NONE',  ( 92.99999999999997158, 107.7255621263696952, -48.40000000546237402 ) ) ;
#8361=CARTESIAN_POINT ( 'NONE',  ( 95.00472066334982912, 116.8754121666685393, -45.67500000273119554 ) ) ;
#8364=CARTESIAN_POINT ( 'NONE',  ( 99.14382582708707048, 122.8000000010924708, -2.066987299999999195 ) ) ;
#8368=ORIENTED_EDGE ( 'NONE', *, *, #11906, .T. ) ;
#8369=DIRECTION ( 'NONE',  ( 0.000000000000000000, -1.000000000000000000, 0.000000000000000000 ) ) ;
#8384=CARTESIAN_POINT ( 'NONE',  ( 99.99999999999998579, 89.99899999999999523, -9.540979117872439019E-15 ) ) ;
#8394=CARTESIAN_POINT ( 'NONE',  ( 101.8468681455907330, 94.49999999863442213, -4.458734124999994997 ) ) ;
#8401=CARTESIAN_POINT ( 'NONE',  ( 104.4587341249999781, 90.31249999863440792, -6.938893903907228378E-15 ) ) ;
#8403=FACE_OUTER_BOUND ( 'NONE', #22838, .T. ) ;
#8408=EDGE_LOOP ( 'NONE', ( #9154, #6882, #10112, #14093 ) ) ;
#8416=VECTOR ( 'NONE', #15402, 1000.000000000000000 ) ;
#8420=LINE ( 'NONE', #23820, #6841 ) ;
#8425=CARTESIAN_POINT ( 'NONE',  ( 95.00472066334982912, 116.8754121666685393, -49.42500000273118133 ) ) ;
#8438=DIRECTION ( 'NONE',  ( 0.000000000000000000, -0.000000000000000000, 1.000000000000000000 ) ) ;
#8442=ORIENTED_EDGE ( 'NONE', *, *, #25568, .T. ) ;
#8443=DIRECTION ( 'NONE',  ( -0.000000000000000000, 1.000000000000000000, -0.000000000000000000 ) ) ;
#8448=CARTESIAN_POINT ( 'NONE',  ( 99.99999999999998579, 102.6397644303321215, -53.50000000000000711 ) ) ;
#8451=CARTESIAN_POINT ( 'NONE',  ( 102.0669872999999939, 123.6000000010924680, -0.8561741729129507261 ) ) ;
#8458=ORIENTED_EDGE ( 'NONE', *, *, #27445, .F. ) ;
#8463=CARTESIAN_POINT ( 'NONE',  ( 103.5355339059327235, 94.87500000000000000, 3.535533905932724874 ) ) ;
#8468=CARTESIAN_POINT ( 'NONE',  ( 102.4999999999999858, 123.0000000000000000, -8.724596124144689908E-15 ) ) ;
#8469=AXIS2_PLACEMENT_3D ( 'NONE', #22618, #11609, #22761 ) ;
#8490=CARTESIAN_POINT ( 'NONE',  ( 101.7677669529663547, 123.0000000021849615, 1.767766952966350891 ) ) ;
#8505=CARTESIAN_POINT ( 'NONE',  ( 99.99999999999998579, 101.5015231886685854, -52.62500000273118417 ) ) ;
#8519=DIRECTION ( 'NONE',  ( 0.000000000000000000, 0.000000000000000000, 1.000000000000000000 ) ) ;
#8528=CARTESIAN_POINT ( 'NONE',  ( 98.96446609406726225, 122.5500000021849587, -2.499999999999997780 ) ) ;
#8530=CARTESIAN_POINT ( 'NONE',  ( 107.0000000000000142, 112.2744378736303190, -54.90000000000000568 ) ) ;
#8538=CARTESIAN_POINT ( 'NONE',  ( 105.6631189606246295, 114.1144967660473242, -45.30000000546237970 ) ) ;
#8539=CARTESIAN_POINT ( 'NONE',  ( 104.4587341249999923, 93.37499999863439371, -1.846868145590737198 ) ) ;
#8545=CARTESIAN_POINT ( 'NONE',  ( 95.54126587499999346, 92.74999999863439371, -1.846868145590737864 ) ) ;
#8546=EDGE_LOOP ( 'NONE', ( #12717, #1597, #9060, #7066 ) ) ;
#8558=CARTESIAN_POINT ( 'NONE',  ( 108.0825317500000153, 110.0000000000000000, -44.12500000273119127 ) ) ;
#8561=VERTEX_POINT ( 'NONE', #19625 ) ;
#8570=CARTESIAN_POINT ( 'NONE',  ( 102.4976396683250925, 102.3130555110000159, -52.52500000273119696 ) ) ;
#8579=PLANE ( 'NONE',  #2980 ) ;
#8581=DIRECTION ( 'NONE',  ( 0.000000000000000000, -1.000000000000000000, 3.469446951953611231E-16 ) ) ;
#8584=DIRECTION ( 'NONE',  ( -0.000000000000000000, 1.000000000000000000, -0.000000000000000000 ) ) ;
#8589=CARTESIAN_POINT ( 'NONE',  ( 97.83688103937537051, 103.3426043859339103, -51.60000000000000853 ) ) ;
#8608=CARTESIAN_POINT ( 'NONE',  ( 99.99999999999998579, 90.00000000000000000, 2.999999999999982681 ) ) ;
#8627=CARTESIAN_POINT ( 'NONE',  ( 99.99999999999998579, 118.4984768113314146, -51.62500000273119127 ) ) ;
#8635=CARTESIAN_POINT ( 'NONE',  ( 0.000000000000000000, 0.000000000000000000, 0.000000000000000000 ) ) ;
#8638=CARTESIAN_POINT ( 'NONE',  ( 98.96446609406727646, 122.8500000021849416, 2.499999999999977796 ) ) ;
#8647=CARTESIAN_POINT ( 'NONE',  ( 104.9952793366501851, 116.8754121666685393, -49.82500000273120122 ) ) ;
#8670=CARTESIAN_POINT ( 'NONE',  ( 91.00000000000000000, 110.0000000000000000, -55.00000000000000711 ) ) ;
#8675=CARTESIAN_POINT ( 'NONE',  ( 108.0825317500000011, 107.3738262389971680, -46.47500000273118559 ) ) ;
#8681=CARTESIAN_POINT ( 'NONE',  ( 98.15313185440925281, 92.62499999863439371, -4.458734124999994997 ) ) ;
#8684=CARTESIAN_POINT ( 'NONE',  ( 104.3262379212492590, 104.0454443415356991, -45.29999999999999716 ) ) ;
#8688=CARTESIAN_POINT ( 'NONE',  ( 98.15313185440925281, 93.99999999863439371, 4.458734124999979898 ) ) ;
#8692=ORIENTED_EDGE ( 'NONE', *, *, #10691, .F. ) ;
#8710=CARTESIAN_POINT ( 'NONE',  ( 99.99999999999998579, 118.4984768113314004, -49.62500000273118417 ) ) ;
#8712=LINE ( 'NONE', #25821, #24428 ) ;
#8723=VERTEX_POINT ( 'NONE', #22623 ) ;
#8727=ORIENTED_EDGE ( 'NONE', *, *, #12749, .F. ) ;
#8728=CARTESIAN_POINT ( 'NONE',  ( 93.00000000000001421, 112.2744378736303332, -52.10000000000000853 ) ) ;
#8730=CARTESIAN_POINT ( 'NONE',  ( 102.0710678118654329, 93.06249999726880162, -5.000000000000023093 ) ) ;
#8733=CARTESIAN_POINT ( 'NONE',  ( 103.5355339059327235, 94.74999999726881583, 3.535533905932724874 ) ) ;
#8743=CARTESIAN_POINT ( 'NONE',  ( 103.5355339059327235, 91.12500000000000000, -3.535533905932738197 ) ) ;
#8766=CARTESIAN_POINT ( 'NONE',  ( 91.91746824999998466, 112.6261737610028320, -51.22500000273119980 ) ) ;
#8769=CARTESIAN_POINT ( 'NONE',  ( 97.50000000000000000, 123.4500000021849502, -1.035533905932742416 ) ) ;
#8774=CARTESIAN_POINT ( 'NONE',  ( 101.7677669529663547, 123.2000000021849502, -1.767766952966370209 ) ) ;
#8782=EDGE_CURVE ( 'NONE', #9247, #28082, #20901, .T. ) ;
#8783=CARTESIAN_POINT ( 'NONE',  ( 102.4976396683250925, 117.6869444889999841, -49.72500000273119269 ) ) ;
#8800=CARTESIAN_POINT ( 'NONE',  ( 99.99999999999998579, 97.00000000000000000, -6.938893903907228378E-15 ) ) ;
#8806=DIRECTION ( 'NONE',  ( -5.782411586589357392E-17, 0.000000000000000000, -1.000000000000000000 ) ) ;
#8808=DIRECTION ( 'NONE',  ( 0.000000000000000000, 1.000000000000000000, 0.000000000000000000 ) ) ;
#8819=CARTESIAN_POINT ( 'NONE',  ( 105.6631189606246295, 105.8855032339526758, -43.70000000546238539 ) ) ;
#8820=CARTESIAN_POINT ( 'NONE',  ( 99.99999999999998579, 95.06249999863440792, 4.458734124999981674 ) ) ;
#8824=ORIENTED_EDGE ( 'NONE', *, *, #15132, .T. ) ;
#8828=CARTESIAN_POINT ( 'NONE',  ( 96.84719886470463734, 93.93749999863440792, 3.152801135295351997 ) ) ;
#8842=CARTESIAN_POINT ( 'NONE',  ( 104.9952793366501709, 103.1245878333314465, -44.42500000273119554 ) ) ;
#8843=CARTESIAN_POINT ( 'NONE',  ( 84.99999999999998579, 102.0000000000000142, -13.00000000000000533 ) ) ;
#8853=CARTESIAN_POINT ( 'NONE',  ( 106.5389055433251002, 105.2492070361643215, -50.32500000273120122 ) ) ;
#8869=CARTESIAN_POINT ( 'NONE',  ( 99.99999999999998579, 102.6397644303321215, -49.50000000000001421 ) ) ;
#8871=CARTESIAN_POINT ( 'NONE',  ( 97.93301269999999192, 124.7000000010924623, -0.8561741729129505041 ) ) ;
#8874=CARTESIAN_POINT ( 'NONE',  ( 102.0710678118654613, 94.06249999726880162, -4.999999999999997335 ) ) ;
#8899=VECTOR ( 'NONE', #14532, 1000.000000000000000 ) ;
#8900=ORIENTED_EDGE ( 'NONE', *, *, #22594, .F. ) ;
#8904=ORIENTED_EDGE ( 'NONE', *, *, #19539, .T. ) ;
#8905=CARTESIAN_POINT ( 'NONE',  ( 102.0710678118653902, 95.06249999726880162, -5.000000000000047073 ) ) ;
#8908=CARTESIAN_POINT ( 'NONE',  ( 104.9952793366501709, 116.8754121666685393, -53.82500000273119412 ) ) ;
#8910=CARTESIAN_POINT ( 'NONE',  ( 98.96446609406727646, 122.8500000021849416, 2.499999999999977796 ) ) ;
#8912=EDGE_CURVE ( 'NONE', #17550, #13582, #20939, .T. ) ;
#8916=VECTOR ( 'NONE', #12419, 1000.000000000000000 ) ;
#8917=CARTESIAN_POINT ( 'NONE',  ( 99.99999999999998579, 123.5500000010924850, -2.066987299999998751 ) ) ;
#8921=FACE_BOUND ( 'NONE', #3481, .T. ) ;
#8924=CARTESIAN_POINT ( 'NONE',  ( 104.9952793366501851, 103.1245878333314323, -44.67500000273118843 ) ) ;
#8930=ORIENTED_EDGE ( 'NONE', *, *, #12640, .T. ) ;
#8931=CARTESIAN_POINT ( 'NONE',  ( 99.99999999999998579, 90.00000000000000000, -4.999999999999996447 ) ) ;
#8942=EDGE_CURVE ( 'NONE', #11, #10673, #6812, .T. ) ;
#8945=CARTESIAN_POINT ( 'NONE',  ( 99.99999999999998579, 93.25000000000000000, -4.999999999999997335 ) ) ;
#8947=ORIENTED_EDGE ( 'NONE', *, *, #14071, .F. ) ;
#8951=CARTESIAN_POINT ( 'NONE',  ( 93.00000000000000000, 112.2744378736303190, -54.10000000000000853 ) ) ;
#8962=CARTESIAN_POINT ( 'NONE',  ( 99.11671166979772352, 122.9999999999999858, 2.356244385768401894 ) ) ;
#8967=EDGE_CURVE ( 'NONE', #11725, #2410, #6399, .T. ) ;
#8971=CARTESIAN_POINT ( 'NONE',  ( 99.99999999999998579, 92.56249999863440792, -4.458734124999994997 ) ) ;
#8979=ORIENTED_EDGE ( 'NONE', *, *, #26208, .F. ) ;
#8984=ORIENTED_EDGE ( 'NONE', *, *, #850, .F. ) ;
#8987=EDGE_CURVE ( 'NONE', #11020, #5734, #13352, .T. ) ;
#8997=EDGE_CURVE ( 'NONE', #8127, #2410, #27687, .T. ) ;
#8998=CARTESIAN_POINT ( 'NONE',  ( 104.9952793366501851, 103.1245878333314323, -48.42500000273120264 ) ) ;
#9008=CARTESIAN_POINT ( 'NONE',  ( 101.4615807364564546, 122.6500000010924794, -1.461580736456474794 ) ) ;
#9016=CARTESIAN_POINT ( 'NONE',  ( 93.46109445667491400, 114.7507929638356785, -51.57500000273120122 ) ) ;
#9018=CARTESIAN_POINT ( 'NONE',  ( 97.50000000000000000, 123.3999999999999915, -9.540979117872439019E-15 ) ) ;
#9023=CARTESIAN_POINT ( 'NONE',  ( 97.92893218813452449, 92.56249999726881583, 4.999999999999983125 ) ) ;
#9028=LINE ( 'NONE', #17720, #18513 ) ;
#9049=EDGE_LOOP ( 'NONE', ( #14719, #9743, #7018, #19855 ) ) ;
#9060=ORIENTED_EDGE ( 'NONE', *, *, #25499, .T. ) ;
#9061=CARTESIAN_POINT ( 'NONE',  ( 99.99999999999998579, 124.3500000010924822, -2.066987299999998751 ) ) ;
#9063=CARTESIAN_POINT ( 'NONE',  ( 99.99999999999998579, 90.00000000000000000, -6.938893903907228378E-15 ) ) ;
#9068=CARTESIAN_POINT ( 'NONE',  ( 97.50236033167492167, 117.6869444889999841, -53.52500000273118985 ) ) ;
#9100=CARTESIAN_POINT ( 'NONE',  ( 104.7293670624999748, 90.71874999795159056, -6.938893903907228378E-15 ) ) ;
#9103=( BOUNDED_SURFACE ( )  B_SPLINE_SURFACE ( 1, 2, ( 
 ( #25330, #6226, #19191, #12342, #27620, #10759, #27893, #5816, #17040, #14892, #8077, #16773, #19047, #5952, #3811, #4089, #12754, #1953, #17605, #26165, #6773, #11175, #8774, #22178, #11461, #15459, #6632, #20180, #377, #8638, #7048, #15316, #13166, #17328, #11318, #22037, #19893, #230, #4651, #4937, #15170 ),
 ( #15747, #26312, #24030, #24174, #9061, #17463, #2657, #26023, #13310, #4509, #6494, #17756, #23889, #24451, #21905, #2379, #4368, #20040, #2513, #26459, #8917, #6913, #13600, #9200, #519, #15604, #13024, #21761, #22323, #24307, #11037, #19747, #4793, #13452, #2238, #17894, #10900, #26602, #2794, #19608, #93 ) ),
 .UNSPECIFIED., .F., .F., .F. ) 
 B_SPLINE_SURFACE_WITH_KNOTS ( ( 2, 2 ),
 ( 3, 2, 2, 2, 2, 2, 2, 2, 2, 2, 2, 2, 2, 2, 2, 2, 2, 2, 2, 2, 3 ),
 ( 0.000000000000000000, 1.000000000000000000 ),
 ( 0.000000000000000000, 0.04166666666666666435, 0.08333333333333332871, 0.1250000000000000000, 0.1666666666666666574, 0.2083333333333333426, 0.2500000000000000000, 0.2916666666666666852, 0.3333333333333333148, 0.3750000000000000000, 0.4166666666666666852, 0.4583333333333333148, 0.5000000000000000000, 0.5416666666666666297, 0.5833333333333333703, 0.6250000000000000000, 0.6666666666666666297, 0.7083333333333333703, 0.7500000000000000000, 0.7916666666666666297, 0.8333333333333333703 ),
 .UNSPECIFIED. ) 
 GEOMETRIC_REPRESENTATION_ITEM ( )  RATIONAL_B_SPLINE_SURFACE ( (
 ( 1.000000000000000000, 0.9238795325112867385, 1.000000000000000000, 0.9238795325112867385, 1.000000000000000000, 0.9238795325112867385, 1.000000000000000000, 0.9238795325112867385, 1.000000000000000000, 0.9238795325112867385, 1.000000000000000000, 0.9238795325112867385, 1.000000000000000000, 0.9238795325112867385, 1.000000000000000000, 0.9238795325112867385, 1.000000000000000000, 0.9238795325112867385, 1.000000000000000000, 0.9238795325112867385, 1.000000000000000000, 0.9238795325112867385, 1.000000000000000000, 0.9238795325112867385, 1.000000000000000000, 0.9238795325112867385, 1.000000000000000000, 0.9238795325112867385, 1.000000000000000000, 0.9238795325112867385, 1.000000000000000000, 0.9238795325112867385, 1.000000000000000000, 0.9238795325112867385, 1.000000000000000000, 0.9238795325112867385, 1.000000000000000000, 0.9238795325112867385, 1.000000000000000000, 0.9238795325112867385, 1.000000000000000000),
 ( 1.000000000000000000, 0.9238795325112867385, 1.000000000000000000, 0.9238795325112867385, 1.000000000000000000, 0.9238795325112867385, 1.000000000000000000, 0.9238795325112867385, 1.000000000000000000, 0.9238795325112867385, 1.000000000000000000, 0.9238795325112867385, 1.000000000000000000, 0.9238795325112867385, 1.000000000000000000, 0.9238795325112867385, 1.000000000000000000, 0.9238795325112867385, 1.000000000000000000, 0.9238795325112867385, 1.000000000000000000, 0.9238795325112867385, 1.000000000000000000, 0.9238795325112867385, 1.000000000000000000, 0.9238795325112867385, 1.000000000000000000, 0.9238795325112867385, 1.000000000000000000, 0.9238795325112867385, 1.000000000000000000, 0.9238795325112867385, 1.000000000000000000, 0.9238795325112867385, 1.000000000000000000, 0.9238795325112867385, 1.000000000000000000, 0.9238795325112867385, 1.000000000000000000, 0.9238795325112867385, 1.000000000000000000) ) ) 
 REPRESENTATION_ITEM ( '' )  SURFACE ( )  );
#9105=CARTESIAN_POINT ( 'NONE',  ( 97.56535394163772423, 123.0000000000000142, 0.5875565381436620438 ) ) ;
#9106=CARTESIAN_POINT ( 'NONE',  ( 99.99999999999998579, 93.12499999726881583, -4.999999999999997335 ) ) ;
#9113=CARTESIAN_POINT ( 'NONE',  ( 98.15313185440925281, 93.62499999863440792, -4.458734124999994997 ) ) ;
#9114=CARTESIAN_POINT ( 'NONE',  ( 96.84719886470463734, 95.18749999863440792, 3.152801135295351997 ) ) ;
#9122=ORIENTED_EDGE ( 'NONE', *, *, #116, .F. ) ;
#9137=CARTESIAN_POINT ( 'NONE',  ( 91.91746824999998466, 107.3738262389971538, -49.02500000273119696 ) ) ;
#9138=DIRECTION ( 'NONE',  ( 5.782411586589357392E-17, -0.000000000000000000, 1.000000000000000000 ) ) ;
#9146=CARTESIAN_POINT ( 'NONE',  ( 98.53841926354351699, 123.0500000010924850, 1.461580736456455920 ) ) ;
#9147=DIRECTION ( 'NONE',  ( 5.782411586589357392E-17, 3.469446951953611231E-16, 1.000000000000000000 ) ) ;
#9148=VECTOR ( 'NONE', #25138, 1000.000000000000000 ) ;
#9150=EDGE_LOOP ( 'NONE', ( #17015, #16319, #17844, #20861 ) ) ;
#9154=ORIENTED_EDGE ( 'NONE', *, *, #8967, .F. ) ;
#9155=CARTESIAN_POINT ( 'NONE',  ( 108.0825317500000011, 112.6261737610028320, -54.27500000273118275 ) ) ;
#9158=CARTESIAN_POINT ( 'NONE',  ( 100.8561741729129153, 122.9000000010924936, -2.066987299999999195 ) ) ;
#9162=CARTESIAN_POINT ( 'NONE',  ( 99.99999999999998579, 95.12499999726881583, -4.999999999999997335 ) ) ;
#9165=CARTESIAN_POINT ( 'NONE',  ( 108.0825317500000011, 107.3738262389971680, -50.47500000273119269 ) ) ;
#9167=EDGE_CURVE ( 'NONE', #6002, #24722, #18509, .T. ) ;
#9177=CARTESIAN_POINT ( 'NONE',  ( 87.00000000000000000, 120.0000000000000000, -43.00000000000000000 ) ) ;
#9193=CARTESIAN_POINT ( 'NONE',  ( 108.0825317500000011, 107.3738262389971680, -52.22500000273119269 ) ) ;
#9199=VERTEX_POINT ( 'NONE', #10205 ) ;
#9200=CARTESIAN_POINT ( 'NONE',  ( 102.0669872999999939, 123.4000000010924936, -0.8561741729129507261 ) ) ;
#9205=CARTESIAN_POINT ( 'NONE',  ( 93.00000000000000000, 107.7255621263696668, -52.40000000546238113 ) ) ;
#9231=VECTOR ( 'NONE', #8584, 1000.000000000000000 ) ;
#9233=CARTESIAN_POINT ( 'NONE',  ( 97.92893218813455292, 94.56249999726881583, 5.000000000000023981 ) ) ;
#9246=CARTESIAN_POINT ( 'NONE',  ( 99.49163138471199375, 123.0000000000000000, -2.452424707819559568 ) ) ;
#9247=VERTEX_POINT ( 'NONE', #25477 ) ;
#9255=CARTESIAN_POINT ( 'NONE',  ( 97.92893218813452449, 93.31250000000001421, -4.999999999999997335 ) ) ;
#9256=CARTESIAN_POINT ( 'NONE',  ( 95.54126587499999346, 95.12499999863439371, 1.846868145590722543 ) ) ;
#9269=CARTESIAN_POINT ( 'NONE',  ( 105.6631189606246295, 105.8855032339526758, -49.70000000546237828 ) ) ;
#9271=CARTESIAN_POINT ( 'NONE',  ( 99.99999999999998579, 91.75000000000000000, 4.999999999999984013 ) ) ;
#9275=CARTESIAN_POINT ( 'NONE',  ( 99.99999999999998579, 123.7000000021849502, 2.499999999999978684 ) ) ;
#9277=CARTESIAN_POINT ( 'NONE',  ( 104.9952793366501851, 103.1245878333314323, -46.42500000273119554 ) ) ;
#9278=CARTESIAN_POINT ( 'NONE',  ( 103.1528011352953484, 91.43749999863440792, 3.152801135295352886 ) ) ;
#9283=CARTESIAN_POINT ( 'NONE',  ( 95.00000000000000000, 91.56249999999998579, 2.071067811865463959 ) ) ;
#9284=CARTESIAN_POINT ( 'NONE',  ( 84.99999999999998579, 97.00000000000000000, -13.00000000000000355 ) ) ;
#9290=CARTESIAN_POINT ( 'NONE',  ( 99.99999999999998579, 117.3602355696678501, -46.50000000000001421 ) ) ;
#9296=ADVANCED_FACE ( 'NONE', ( #27489 ), #10487, .T. ) ;
#9297=CARTESIAN_POINT ( 'NONE',  ( 103.5355339059327235, 93.99999999726881583, -3.535533905932738197 ) ) ;
#9301=CARTESIAN_POINT ( 'NONE',  ( 91.91746824999999887, 110.0000000000000000, -53.37500000273119838 ) ) ;
#9308=CARTESIAN_POINT ( 'NONE',  ( 107.0000000000000142, 110.0000000000000000, -55.00000000000000711 ) ) ;
#9311=CARTESIAN_POINT ( 'NONE',  ( 104.4587341249999923, 91.62499999863439371, -1.846868145590737198 ) ) ;
#9328=CARTESIAN_POINT ( 'NONE',  ( 91.91746824999998466, 112.6261737610028320, -47.22500000273119269 ) ) ;
#9334=ORIENTED_EDGE ( 'NONE', *, *, #484, .F. ) ;
#9342=CARTESIAN_POINT ( 'NONE',  ( 104.9999999999999858, 95.87499999726881583, -6.938893903907228378E-15 ) ) ;
#9343=CARTESIAN_POINT ( 'NONE',  ( 103.1528011352953484, 92.18749999863440792, 3.152801135295352886 ) ) ;
#9344=( BOUNDED_CURVE ( )  B_SPLINE_CURVE ( 2, ( #4830, #11492, #13489, #22210, #11350, #551, #5108, #9233, #17925 ),
 .UNSPECIFIED., .F., .T. ) 
 B_SPLINE_CURVE_WITH_KNOTS ( ( 3, 2, 2, 2, 3 ),
 ( 0.6500000000000005773, 0.6750000000000005995, 0.7000000000000006217, 0.7250000000000006439, 0.7500000000000006661 ),
 .UNSPECIFIED. ) 
 CURVE ( )  GEOMETRIC_REPRESENTATION_ITEM ( )  RATIONAL_B_SPLINE_CURVE ( ( 0.9999999999999983347, 0.9238795325112884038, 1.000000000000000000, 0.9238795325112867385, 1.000000000000000000, 0.9238795325112867385, 1.000000000000000000, 0.9238795325112847401, 1.000000000000001998 ) ) 
 REPRESENTATION_ITEM ( '' )  );
#9345=CARTESIAN_POINT ( 'NONE',  ( 97.50236033167492167, 117.6869444889999841, -47.52500000273119696 ) ) ;
#9347=ADVANCED_FACE ( 'NONE', ( #16504 ), #25198, .T. ) ;
#9348=VECTOR ( 'NONE', #5575, 1000.000000000000000 ) ;
#9354=ORIENTED_EDGE ( 'NONE', *, *, #21989, .T. ) ;
#9372=CARTESIAN_POINT ( 'NONE',  ( 94.33688103937537051, 114.1144967660473242, -54.20000000000000284 ) ) ;
#9380=CARTESIAN_POINT ( 'NONE',  ( 108.0825317500000011, 107.3738262389971538, -52.47500000273118559 ) ) ;
#9381=CARTESIAN_POINT ( 'NONE',  ( 102.4515117831381730, 123.0000000000000000, -0.5701068363804095984 ) ) ;
#9387=ORIENTED_EDGE ( 'NONE', *, *, #606, .T. ) ;
#9389=CARTESIAN_POINT ( 'NONE',  ( 99.99999999999998579, 94.75000000000000000, 4.999999999999984013 ) ) ;
#9391=CARTESIAN_POINT ( 'NONE',  ( 104.9999999999999716, 93.06249999999998579, -2.071067811865478170 ) ) ;
#9396=CARTESIAN_POINT ( 'NONE',  ( 97.92893218813459555, 95.56249999726881583, 5.000000000000046185 ) ) ;
#9401=AXIS2_PLACEMENT_3D ( 'NONE', #16073, #18511, #855 ) ;
#9406=CARTESIAN_POINT ( 'NONE',  ( 106.9999999999999858, 107.7255621263696241, -49.60000000546236976 ) ) ;
#9407=CARTESIAN_POINT ( 'NONE',  ( 99.99999999999998579, 92.06249999863440792, 4.458734124999981674 ) ) ;
#9409=VECTOR ( 'NONE', #27035, 1000.000000000000000 ) ;
#9415=CARTESIAN_POINT ( 'NONE',  ( 91.91746824999999887, 110.0000000000000000, -47.12500000273119838 ) ) ;
#9416=CARTESIAN_POINT ( 'NONE',  ( 96.84719886470463734, 92.18749999863440792, 3.152801135295351997 ) ) ;
#9422=FACE_OUTER_BOUND ( 'NONE', #25140, .T. ) ;
#9430=VERTEX_POINT ( 'NONE', #17187 ) ;
#9431=CARTESIAN_POINT ( 'NONE',  ( 105.6631189606246295, 105.8855032339526758, -47.20000000000000284 ) ) ;
#9433=CARTESIAN_POINT ( 'NONE',  ( 102.0669872999999939, 122.8000000010924708, -0.8561741729129507261 ) ) ;
#9438=CARTESIAN_POINT ( 'NONE',  ( 95.54126587499999346, 94.12499999863439371, 1.846868145590722543 ) ) ;
#9441=CARTESIAN_POINT ( 'NONE',  ( 91.91746824999998466, 112.6261737610028320, -49.47500000273119269 ) ) ;
#9453=CARTESIAN_POINT ( 'NONE',  ( 96.84719886470463734, 92.18749999863440792, 3.152801135295351997 ) ) ;
#9459=VERTEX_POINT ( 'NONE', #381 ) ;
#9469=CARTESIAN_POINT ( 'NONE',  ( 91.91746824999998466, 112.6261737610028320, -45.22500000273119980 ) ) ;
#9483=CARTESIAN_POINT ( 'NONE',  ( 99.99999999999998579, 95.62499999726881583, 4.999999999999984013 ) ) ;
#9484=CARTESIAN_POINT ( 'NONE',  ( 95.00472066334982912, 116.8754121666685393, -47.42500000273118843 ) ) ;
#9489=CARTESIAN_POINT ( 'NONE',  ( 103.5355339059327235, 91.74999999726880162, 3.535533905932724874 ) ) ;
#9499=ADVANCED_FACE ( 'NONE', ( #13028 ), #13316, .F. ) ;
#9500=DIRECTION ( 'NONE',  ( 5.782411586589357392E-17, -0.000000000000000000, 1.000000000000000000 ) ) ;
#9502=AXIS2_PLACEMENT_3D ( 'NONE', #3731, #19527, #2150 ) ;
#9506=DIRECTION ( 'NONE',  ( 5.782411586589357392E-17, 0.000000000000000000, 1.000000000000000000 ) ) ;
#9510=CARTESIAN_POINT ( 'NONE',  ( 98.23223304703363112, 124.3069999999781459, 1.767766952966351557 ) ) ;
#9527=CARTESIAN_POINT ( 'NONE',  ( 99.99999999999998579, 90.75000000000000000, 4.999999999999984013 ) ) ;
#9528=CARTESIAN_POINT ( 'NONE',  ( 97.50120075755764049, 123.0000000000000000, 0.1653216690150871027 ) ) ;
#9533=ORIENTED_EDGE ( 'NONE', *, *, #7781, .F. ) ;
#9538=CARTESIAN_POINT ( 'NONE',  ( 104.9999999999999716, 90.93749999999998579, 2.071067811865467956 ) ) ;
#9550=EDGE_CURVE ( 'NONE', #15121, #7547, #19493, .T. ) ;
#9559=CARTESIAN_POINT ( 'NONE',  ( 99.99999999999998579, 90.00000000000000000, 2.999999999999982681 ) ) ;
#9561=CARTESIAN_POINT ( 'NONE',  ( 102.4976396683250925, 117.6869444889999841, -45.72500000273119269 ) ) ;
#9562=CARTESIAN_POINT ( 'NONE',  ( 99.99999999999998579, 91.81249999863440792, -4.458734124999994997 ) ) ;
#9569=CARTESIAN_POINT ( 'NONE',  ( 104.9999999999999858, 95.43749999863440792, -6.938893903907228378E-15 ) ) ;
#9576=CARTESIAN_POINT ( 'NONE',  ( 104.3262379212492590, 104.0454443415356991, -45.29999999999999716 ) ) ;
#9578=CARTESIAN_POINT ( 'NONE',  ( 97.50000000000000000, 124.1499999999999915, -1.035533905932742416 ) ) ;
#9583=CARTESIAN_POINT ( 'NONE',  ( 95.54126587499999346, 92.12499999863437949, 1.846868145590722543 ) ) ;
#9585=CARTESIAN_POINT ( 'NONE',  ( 108.0825317500000153, 110.0000000000000000, -48.37500000273119838 ) ) ;
#9591=CARTESIAN_POINT ( 'NONE',  ( 99.99999999999998579, 124.3999999999999915, 2.499999999999978684 ) ) ;
#9597=LINE ( 'NONE', #9177, #27158 ) ;
#9609=CARTESIAN_POINT ( 'NONE',  ( 104.7293670624999748, 95.15624999931721106, -6.938893903907228378E-15 ) ) ;
#9613=CARTESIAN_POINT ( 'NONE',  ( 93.46109445667491400, 114.7507929638356785, -47.32500000273119412 ) ) ;
#9617=ORIENTED_EDGE ( 'NONE', *, *, #23297, .T. ) ;
#9620=ORIENTED_EDGE ( 'NONE', *, *, #15372, .T. ) ;
#9624=CARTESIAN_POINT ( 'NONE',  ( 104.7293670624999748, 90.15624999931721106, -6.938893903907228378E-15 ) ) ;
#9627=CARTESIAN_POINT ( 'NONE',  ( 93.46109445667491400, 105.2492070361643215, -44.92500000273119554 ) ) ;
#9635=ADVANCED_FACE ( 'NONE', ( #21619, #8921 ), #15320, .T. ) ;
#9638=( BOUNDED_CURVE ( )  B_SPLINE_CURVE ( 2, ( #5087, #26613, #15757, #11328, #7060, #24463, #4946, #26755, #14179, #8049, #27321 ),
 .UNSPECIFIED., .F., .F. ) 
 B_SPLINE_CURVE_WITH_KNOTS ( ( 3, 2, 2, 2, 2, 3 ),
 ( 0.3999999999999996891, 0.4199999999999996514, 0.4399999999999996692, 0.4599999999999996869, 0.4799999999999996492, 0.4999999999999996669 ),
 .UNSPECIFIED. ) 
 CURVE ( )  GEOMETRIC_REPRESENTATION_ITEM ( )  RATIONAL_B_SPLINE_CURVE ( ( 1.000000000000000888, 0.9510565162951527540, 1.000000000000000000, 0.9510565162951535312, 1.000000000000000000, 0.9510565162951535312, 1.000000000000000000, 0.9510565162951535312, 1.000000000000000000, 0.9510565162951543083, 0.9999999999999992228 ) ) 
 REPRESENTATION_ITEM ( '' )  );
#9647=FACE_BOUND ( 'NONE', #22999, .T. ) ;
#9662=DIRECTION ( 'NONE',  ( -5.782411586589357392E-17, 0.000000000000000000, -1.000000000000000000 ) ) ;
#9665=CARTESIAN_POINT ( 'NONE',  ( 97.50236033167492167, 117.6869444889999841, -53.77500000273119696 ) ) ;
#9677=CARTESIAN_POINT ( 'NONE',  ( 102.0710678118654613, 94.18749999999998579, -4.999999999999997335 ) ) ;
#9679=ADVANCED_FACE ( 'NONE', ( #5470, #7599 ), #14139, .F. ) ;
#9697=CARTESIAN_POINT ( 'NONE',  ( 96.84719886470463734, 92.68749999863440792, -3.152801135295366208 ) ) ;
#9704=CARTESIAN_POINT ( 'NONE',  ( 107.0000000000000142, 110.0000000000000000, -47.50000000546238255 ) ) ;
#9705=CARTESIAN_POINT ( 'NONE',  ( 97.50000000000000000, 124.2500000021849900, -1.035533905932742416 ) ) ;
#9707=DIRECTION ( 'NONE',  ( 0.000000000000000000, 0.000000000000000000, -1.000000000000000000 ) ) ;
#9712=CARTESIAN_POINT ( 'NONE',  ( 97.92893218813451028, 91.31249999999998579, -4.999999999999984013 ) ) ;
#9719=CARTESIAN_POINT ( 'NONE',  ( 99.99999999999998579, 118.4984768113314004, -49.87500000273118417 ) ) ;
#9726=CARTESIAN_POINT ( 'NONE',  ( 98.15313185440925281, 93.24999999863439371, 4.458734124999979898 ) ) ;
#9728=CARTESIAN_POINT ( 'NONE',  ( 95.00472066334981491, 103.1245878333314465, -51.07500000273119412 ) ) ;
#9734=DIRECTION ( 'NONE',  ( 5.782411586589357392E-17, -0.000000000000000000, 1.000000000000000000 ) ) ;
#9743=ORIENTED_EDGE ( 'NONE', *, *, #5433, .F. ) ;
#9748=ORIENTED_EDGE ( 'NONE', *, *, #7968, .F. ) ;
#9754=DIRECTION ( 'NONE',  ( -0.000000000000000000, 1.000000000000000000, -0.000000000000000000 ) ) ;
#9756=ORIENTED_EDGE ( 'NONE', *, *, #18381, .T. ) ;
#9766=CARTESIAN_POINT ( 'NONE',  ( 108.0825317500000011, 107.3738262389971538, -44.22500000273118559 ) ) ;
#9771=CARTESIAN_POINT ( 'NONE',  ( 103.5355339059327235, 90.99999999726880162, -3.535533905932738197 ) ) ;
#9774=ORIENTED_EDGE ( 'NONE', *, *, #3693, .T. ) ;
#9791=LINE ( 'NONE', #1673, #18382 ) ;
#9793=SURFACE_SIDE_STYLE ('',( #11919 ) ) ;
#9795=CARTESIAN_POINT ( 'NONE',  ( 99.99999999999998579, 102.6397644303321215, -47.50000000000000711 ) ) ;
#9806=CARTESIAN_POINT ( 'NONE',  ( 91.91746824999998466, 112.6261737610028320, -53.47500000273119980 ) ) ;
#9815=CARTESIAN_POINT ( 'NONE',  ( 99.99999999999998579, 94.25000000000000000, -4.999999999999997335 ) ) ;
#9817=CARTESIAN_POINT ( 'NONE',  ( 95.00000000000000000, 92.50000000000000000, -7.551217303480904118E-15 ) ) ;
#9822=ORIENTED_EDGE ( 'NONE', *, *, #12253, .T. ) ;
#9838=CARTESIAN_POINT ( 'NONE',  ( 97.50000000000000000, 123.4500000000000028, 1.035533905932725096 ) ) ;
#9840=CARTESIAN_POINT ( 'NONE',  ( 99.99999999999998579, 117.3602355696678501, -47.00000000546238255 ) ) ;
#9841=CARTESIAN_POINT ( 'NONE',  ( 101.8468681455907330, 93.74999999863439371, -4.458734124999994997 ) ) ;
#9844=DIRECTION ( 'NONE',  ( 0.000000000000000000, -1.000000000000000000, 0.000000000000000000 ) ) ;
#9858=CARTESIAN_POINT ( 'NONE',  ( 91.91746824999998466, 112.6261737610028320, -47.47500000273119269 ) ) ;
#9865=CARTESIAN_POINT ( 'NONE',  ( 98.15313185440925281, 91.24999999863439371, 4.458734124999979898 ) ) ;
#9866=DIRECTION ( 'NONE',  ( 0.000000000000000000, 0.000000000000000000, 1.000000000000000000 ) ) ;
#9874=ORIENTED_EDGE ( 'NONE', *, *, #19965, .F. ) ;
#9877=CARTESIAN_POINT ( 'NONE',  ( 96.84719886470463734, 94.18749999863440792, 3.152801135295351997 ) ) ;
#9887=CARTESIAN_POINT ( 'NONE',  ( 99.99999999999998579, 92.75000000000000000, 4.999999999999984013 ) ) ;
#9893=CARTESIAN_POINT ( 'NONE',  ( 94.99999999999998579, 110.0000000000000000, -43.00000000000000000 ) ) ;
#9904=CYLINDRICAL_SURFACE ( 'NONE', #6750, 4.999999999999989342 ) ;
#9919=CARTESIAN_POINT ( 'NONE',  ( 98.96446609406726225, 124.3500000000000085, 2.499999999999981348 ) ) ;
#9920=CARTESIAN_POINT ( 'NONE',  ( 97.50000000000000000, 123.4569999999781373, 1.035533905932725096 ) ) ;
#9929=CARTESIAN_POINT ( 'NONE',  ( 99.99999999999998579, 90.00000000000000000, -4.999999999999996447 ) ) ;
#9937=CARTESIAN_POINT ( 'NONE',  ( 106.5389055433251002, 105.2492070361643215, -48.57500000273119412 ) ) ;
#9940=CARTESIAN_POINT ( 'NONE',  ( 97.93301269999999192, 123.2000000010924765, 0.8561741729129329626 ) ) ;
#9946=ADVANCED_FACE ( 'NONE', ( #25754 ), #12352, .F. ) ;
#9956=ORIENTED_EDGE ( 'NONE', *, *, #476, .T. ) ;
#9958=ORIENTED_EDGE ( 'NONE', *, *, #24151, .F. ) ;
#9972=CARTESIAN_POINT ( 'NONE',  ( 107.0000000000000142, 112.2744378736303190, -53.40000000546236691 ) ) ;
#9974=CARTESIAN_POINT ( 'NONE',  ( 99.99999999999998579, 102.6397644303321215, -48.00000000546237544 ) ) ;
#9976=CARTESIAN_POINT ( 'NONE',  ( 104.4587341249999923, 94.62499999863439371, -1.846868145590737198 ) ) ;
#9979=CARTESIAN_POINT ( 'NONE',  ( 114.9999999999999858, 100.0000000000000000, -15.00000000000000711 ) ) ;
#9981=ORIENTED_EDGE ( 'NONE', *, *, #21320, .T. ) ;
#9983=CARTESIAN_POINT ( 'NONE',  ( 99.99999999999998579, 123.3000000021849587, -2.499999999999997780 ) ) ;
#9989=EDGE_LOOP ( 'NONE', ( #22899, #11457 ) ) ;
#9990=CARTESIAN_POINT ( 'NONE',  ( 93.46109445667491400, 114.7507929638356785, -47.57500000273119412 ) ) ;
#9997=CARTESIAN_POINT ( 'NONE',  ( 103.1528011352953484, 93.43749999863440792, 3.152801135295352886 ) ) ;
#9998=DIRECTION ( 'NONE',  ( -0.000000000000000000, 1.000000000000000000, -0.000000000000000000 ) ) ;
#10005=CARTESIAN_POINT ( 'NONE',  ( 84.99999999999998579, 95.00000000000000000, 14.99999999999999467 ) ) ;
#10006=CARTESIAN_POINT ( 'NONE',  ( 93.00000000000000000, 110.0000000000000000, -55.00000000000000711 ) ) ;
#10012=CARTESIAN_POINT ( 'NONE',  ( 98.15313185440923860, 92.87499999863439371, -4.458734124999994997 ) ) ;
#10017=ORIENTED_EDGE ( 'NONE', *, *, #17241, .F. ) ;
#10024=FACE_OUTER_BOUND ( 'NONE', #13804, .T. ) ;
#10030=EDGE_LOOP ( 'NONE', ( #27398, #21276, #17893, #1381 ) ) ;
#10052=LINE ( 'NONE', #22910, #27988 ) ;
#10059=CARTESIAN_POINT ( 'NONE',  ( 101.0355339059327378, 123.6569999999781544, 2.499999999999977796 ) ) ;
#10073=CARTESIAN_POINT ( 'NONE',  ( 91.91746824999998466, 112.6261737610028320, -47.47500000273119269 ) ) ;
#10074=DIRECTION ( 'NONE',  ( 0.000000000000000000, 0.000000000000000000, 1.000000000000000000 ) ) ;
#10075=CARTESIAN_POINT ( 'NONE',  ( 98.53841926354351699, 123.8500000010924680, -1.461580736456474794 ) ) ;
#10081=CARTESIAN_POINT ( 'NONE',  ( 99.99999999999998579, 90.00000000000000000, -6.938893903907228378E-15 ) ) ;
#10098=CARTESIAN_POINT ( 'NONE',  ( 101.8468681455907330, 93.12499999863439371, 4.458734124999980786 ) ) ;
#10102=DIRECTION ( 'NONE',  ( 0.000000000000000000, -1.000000000000000000, -0.000000000000000000 ) ) ;
#10105=CARTESIAN_POINT ( 'NONE',  ( 102.1631189606246295, 103.3426043859339103, -45.90000000546237402 ) ) ;
#10106=CARTESIAN_POINT ( 'NONE',  ( 99.99999999999998579, 92.81249999863440792, -4.458734124999994997 ) ) ;
#10112=ORIENTED_EDGE ( 'NONE', *, *, #5547, .T. ) ;
#10114=( BOUNDED_CURVE ( )  B_SPLINE_CURVE ( 2, ( #9483, #18184, #16178, #22757, #9342 ),
 .UNSPECIFIED., .F., .T. ) 
 B_SPLINE_CURVE_WITH_KNOTS ( ( 3, 2, 3 ),
 ( 0.9500000000000009548, 0.9750000000000005329, 1.000000000000000000 ),
 .UNSPECIFIED. ) 
 CURVE ( )  GEOMETRIC_REPRESENTATION_ITEM ( )  RATIONAL_B_SPLINE_CURVE ( ( 0.9999999999999970024, 0.9238795325112897361, 1.000000000000000000, 0.9238795325112867385, 1.000000000000000000 ) ) 
 REPRESENTATION_ITEM ( '' )  );
#10119=CARTESIAN_POINT ( 'NONE',  ( 95.00472066334982912, 103.1245878333314323, -49.07500000273118701 ) ) ;
#10123=CARTESIAN_POINT ( 'NONE',  ( 108.0825317500000011, 112.6261737610028320, -46.02500000273120406 ) ) ;
#10130=FACE_OUTER_BOUND ( 'NONE', #4177, .T. ) ;
#10140=CARTESIAN_POINT ( 'NONE',  ( 103.1528011352953484, 95.43749999863440792, 3.152801135295352886 ) ) ;
#10146=CARTESIAN_POINT ( 'NONE',  ( 97.93301270000000613, 123.1000000010924822, -0.8561741729129506151 ) ) ;
#10151=CARTESIAN_POINT ( 'NONE',  ( 84.99999999999998579, 102.0000000000000142, -15.00000000000000711 ) ) ;
#10155=CARTESIAN_POINT ( 'NONE',  ( 103.5355339059327235, 90.12500000000000000, -3.535533905932738197 ) ) ;
#10164=CARTESIAN_POINT ( 'NONE',  ( 95.00000000000000000, 92.43749999726880162, 2.071067811865463959 ) ) ;
#10168=CARTESIAN_POINT ( 'NONE',  ( 102.0669872999999797, 122.7500000010924737, -9.794112055954760458E-15 ) ) ;
#10169=CARTESIAN_POINT ( 'NONE',  ( 87.00000000000000000, 118.0000000000000000, -43.00000000000000000 ) ) ;
#10190=CARTESIAN_POINT ( 'NONE',  ( 101.7677669529663547, 124.7000000000000028, -1.767766952966370209 ) ) ;
#10192=CARTESIAN_POINT ( 'NONE',  ( 97.93301270000000613, 124.0000000010924879, 0.8561741729129328515 ) ) ;
#10198=VERTEX_POINT ( 'NONE', #11186 ) ;
#10205=CARTESIAN_POINT ( 'NONE',  ( 93.00000000000000000, 110.0000000000000000, -52.00000000000000711 ) ) ;
#10208=CARTESIAN_POINT ( 'NONE',  ( 97.50236033167492167, 102.3130555110000159, -50.97500000273119980 ) ) ;
#10209=CARTESIAN_POINT ( 'NONE',  ( 102.0710678118653902, 94.18749999999998579, -5.000000000000047073 ) ) ;
#10210=CARTESIAN_POINT ( 'NONE',  ( 102.0669872999999939, 122.6000000010924964, -0.8561741729129507261 ) ) ;
#10243=CARTESIAN_POINT ( 'NONE',  ( 93.00000000000000000, 110.0000000000000000, -50.50000000546237544 ) ) ;
#10244=CARTESIAN_POINT ( 'NONE',  ( 101.8468681455907330, 94.74999999863440792, -4.458734124999994997 ) ) ;
#10248=EDGE_LOOP ( 'NONE', ( #9617, #8824, #1243, #15179, #1963, #650 ) ) ;
#10258=CARTESIAN_POINT ( 'NONE',  ( 104.9952793366501851, 116.8754121666685393, -50.07500000273120122 ) ) ;
#10262=CARTESIAN_POINT ( 'NONE',  ( 102.4976396683250925, 117.6869444889999841, -49.72500000273119269 ) ) ;
#10263=CARTESIAN_POINT ( 'NONE',  ( 93.00000000000001421, 107.7255621263696668, -51.90000000000000568 ) ) ;
#10266=EDGE_LOOP ( 'NONE', ( #7348, #9533, #16000, #15265 ) ) ;
#10268=VECTOR ( 'NONE', #2938, 1000.000000000000000 ) ;
#10269=FACE_OUTER_BOUND ( 'NONE', #8228, .T. ) ;
#10277=DIRECTION ( 'NONE',  ( -1.000000000000000000, 0.000000000000000000, 0.000000000000000000 ) ) ;
#10281=CARTESIAN_POINT ( 'NONE',  ( 97.93301270000000613, 123.7500000010924879, -9.540979117872439019E-15 ) ) ;
#10282=CARTESIAN_POINT ( 'NONE',  ( 104.4587341249999923, 93.49999999863440792, 1.846868145590726318 ) ) ;
#10294=FACE_BOUND ( 'NONE', #12628, .T. ) ;
#10306=DIRECTION ( 'NONE',  ( -1.000000000000000000, 0.000000000000000000, 0.000000000000000000 ) ) ;
#10308=CARTESIAN_POINT ( 'NONE',  ( 102.4999999999999858, 123.0000000000000000, -8.724596124144689908E-15 ) ) ;
#10310=CARTESIAN_POINT ( 'NONE',  ( 104.9999999999999858, 93.87499999726881583, -6.938893903907228378E-15 ) ) ;
#10330=CARTESIAN_POINT ( 'NONE',  ( 98.96446609406727646, 123.2569999999781487, -2.499999999999997780 ) ) ;
#10331=EDGE_CURVE ( 'NONE', #24831, #24171, #21771, .T. ) ;
#10333=CARTESIAN_POINT ( 'NONE',  ( 99.99999999999998579, 123.3500000010924680, 2.066987299999980099 ) ) ;
#10338=DIRECTION ( 'NONE',  ( 0.000000000000000000, 0.000000000000000000, 1.000000000000000000 ) ) ;
#10339=AXIS2_PLACEMENT_3D ( 'NONE', #12875, #6622, #26015 ) ;
#10341=AXIS2_PLACEMENT_3D ( 'NONE', #4063, #4339, #23726 ) ;
#10347=CARTESIAN_POINT ( 'NONE',  ( 102.4976396683250925, 102.3130555110000159, -46.77500000273119696 ) ) ;
#10349=CARTESIAN_POINT ( 'NONE',  ( 99.14382582708707048, 124.1000000010924964, 2.066987299999979211 ) ) ;
#10373=CARTESIAN_POINT ( 'NONE',  ( 97.50000000000000000, 122.7500000021849615, 1.035533905932725096 ) ) ;
#10375=CARTESIAN_POINT ( 'NONE',  ( 95.54126587500000767, 94.81249999863440792, -7.484931351350258973E-15 ) ) ;
#10385=CARTESIAN_POINT ( 'NONE',  ( 98.15313185440925281, 90.62499999863439371, -4.458734124999994997 ) ) ;
#10390=VECTOR ( 'NONE', #15875, 1000.000000000000000 ) ;
#10391=ORIENTED_EDGE ( 'NONE', *, *, #446, .F. ) ;
#10394=CARTESIAN_POINT ( 'NONE',  ( 99.99999999999998579, 91.56249999863440792, -4.458734124999994997 ) ) ;
#10423=CARTESIAN_POINT ( 'NONE',  ( 107.0000000000000142, 110.0000000000000000, -55.00000000000000711 ) ) ;
#10427=DIRECTION ( 'NONE',  ( 1.000000000000000000, 0.000000000000000000, 0.000000000000000000 ) ) ;
#10438=CARTESIAN_POINT ( 'NONE',  ( 97.92893218813455292, 92.68749999999998579, 5.000000000000011546 ) ) ;
#10454=CARTESIAN_POINT ( 'NONE',  ( 102.0669872999999797, 122.5500000010924850, -9.794112055954760458E-15 ) ) ;
#10475=CARTESIAN_POINT ( 'NONE',  ( 102.4999999999999858, 122.9976688166997860, 0.1932551333443592867 ) ) ;
#10477=CARTESIAN_POINT ( 'NONE',  ( 97.93301270000000613, 123.2000000010924765, 0.8561741729129328515 ) ) ;
#10483=FACE_OUTER_BOUND ( 'NONE', #21156, .T. ) ;
#10487=PLANE ( 'NONE',  #4021 ) ;
#10491=CARTESIAN_POINT ( 'NONE',  ( 97.50236033167492167, 102.3130555110000159, -46.97500000273119269 ) ) ;
#10494=CARTESIAN_POINT ( 'NONE',  ( 97.93301270000000613, 124.7500000010924737, -9.540979117872439019E-15 ) ) ;
#10509=CARTESIAN_POINT ( 'NONE',  ( 94.33688103937537051, 114.1144967660473242, -46.70000000546237828 ) ) ;
#10516=CARTESIAN_POINT ( 'NONE',  ( 95.54126587499999346, 94.74999999863439371, -1.846868145590737864 ) ) ;
#10517=CARTESIAN_POINT ( 'NONE',  ( 99.99999999999998579, 89.99899999999999523, -2.500000000000004885 ) ) ;
#10525=EDGE_CURVE ( 'NONE', #23799, #8723, #14739, .T. ) ;
#10527=CARTESIAN_POINT ( 'NONE',  ( 107.0000000000000142, 107.7255621263696526, -43.60000000546237686 ) ) ;
#10528=CARTESIAN_POINT ( 'NONE',  ( 104.4587341249999781, 94.31249999863440792, -6.938893903907228378E-15 ) ) ;
#10531=CARTESIAN_POINT ( 'NONE',  ( 107.0000000000000142, 110.0000000000000000, -45.00000000000000711 ) ) ;
#10532=ADVANCED_FACE ( 'NONE', ( #27731 ), #9904, .T. ) ;
#10554=DIRECTION ( 'NONE',  ( 0.8660254037844380415, 0.5000000000000013323, 0.000000000000000000 ) ) ;
#10560=CARTESIAN_POINT ( 'NONE',  ( 108.0825317500000153, 110.0000000000000000, -50.12500000273119127 ) ) ;
#10579=CARTESIAN_POINT ( 'NONE',  ( 102.1631189606246295, 103.3426043859339103, -49.40000000000000568 ) ) ;
#10581=CARTESIAN_POINT ( 'NONE',  ( 99.99999999999998579, 124.5500000010924708, -2.066987299999998751 ) ) ;
#10590=ORIENTED_EDGE ( 'NONE', *, *, #16450, .F. ) ;
#10595=FACE_OUTER_BOUND ( 'NONE', #17560, .T. ) ;
#10601=VECTOR ( 'NONE', #2629, 1000.000000000000000 ) ;
#10617=CARTESIAN_POINT ( 'NONE',  ( 99.99999999999998579, 122.9000000021849530, 2.499999999999978684 ) ) ;
#10630=CARTESIAN_POINT ( 'NONE',  ( 95.00472066334982912, 103.1245878333314323, -50.82500000273118701 ) ) ;
#10636=ORIENTED_EDGE ( 'NONE', *, *, #12253, .F. ) ;
#10650=CARTESIAN_POINT ( 'NONE',  ( 99.99999999999998579, 92.75000000000000000, 4.999999999999984013 ) ) ;
#10651=FACE_OUTER_BOUND ( 'NONE', #19260, .T. ) ;
#10658=CARTESIAN_POINT ( 'NONE',  ( 97.50236033167492167, 102.3130555110000159, -44.97500000273119980 ) ) ;
#10662=CARTESIAN_POINT ( 'NONE',  ( 107.0000000000000142, 110.0000000000000000, -43.50000000546237544 ) ) ;
#10663=CARTESIAN_POINT ( 'NONE',  ( 104.4587341249999923, 92.24999999863439371, 1.846868145590726318 ) ) ;
#10667=ORIENTED_EDGE ( 'NONE', *, *, #5693, .F. ) ;
#10669=CARTESIAN_POINT ( 'NONE',  ( 95.54126587500000767, 94.81249999863440792, -7.484931351350258973E-15 ) ) ;
#10673=VERTEX_POINT ( 'NONE', #24148 ) ;
#10677=EDGE_CURVE ( 'NONE', #25390, #19945, #14909, .T. ) ;
#10683=CARTESIAN_POINT ( 'NONE',  ( 102.4976396683250925, 102.3130555110000159, -44.52500000273119696 ) ) ;
#10684=CARTESIAN_POINT ( 'NONE',  ( 105.6631189606246295, 105.8855032339526758, -51.20000000000000995 ) ) ;
#10691=EDGE_CURVE ( 'NONE', #20441, #1383, #4485, .T. ) ;
#10695=CARTESIAN_POINT ( 'NONE',  ( 99.99999999999998579, 101.5015231886685854, -50.62500000273119838 ) ) ;
#10703=CARTESIAN_POINT ( 'NONE',  ( 102.1631189606246295, 116.6573956140660897, -51.10000000546237686 ) ) ;
#10705=CARTESIAN_POINT ( 'NONE',  ( 99.99999999999998579, 124.3500000010924822, -2.066987299999998751 ) ) ;
#10710=EDGE_LOOP ( 'NONE', ( #11833, #1091, #24150, #26261, #26547 ) ) ;
#10715=CARTESIAN_POINT ( 'NONE',  ( 93.00000000000000000, 110.0000000000000000, -52.00000000000000711 ) ) ;
#10718=CARTESIAN_POINT ( 'NONE',  ( 101.4615807364564546, 124.2500000010924737, 1.461580736456455476 ) ) ;
#10726=ORIENTED_EDGE ( 'NONE', *, *, #7041, .F. ) ;
#10746=CARTESIAN_POINT ( 'NONE',  ( 102.1631189606246295, 103.3426043859339103, -45.90000000546237402 ) ) ;
#10750=CYLINDRICAL_SURFACE ( 'NONE', #7581, 4.999999999999989342 ) ;
#10752=CARTESIAN_POINT ( 'NONE',  ( 106.5389055433251002, 114.7507929638356785, -51.92500000273119554 ) ) ;
#10759=CARTESIAN_POINT ( 'NONE',  ( 101.0355339059327378, 124.0500000021849445, -2.499999999999997780 ) ) ;
#10766=CARTESIAN_POINT ( 'NONE',  ( 108.0825317500000011, 107.3738262389971538, -50.22500000273118559 ) ) ;
#10779=DIRECTION ( 'NONE',  ( 1.000000000000000000, -0.000000000000000000, -5.782411586589357392E-17 ) ) ;
#10783=CARTESIAN_POINT ( 'NONE',  ( 95.67376207875072680, 115.9545556584642867, -46.80000000546237260 ) ) ;
#10789=CARTESIAN_POINT ( 'NONE',  ( 97.93301270000000613, 124.6500000010924651, -9.540979117872439019E-15 ) ) ;
#10801=CARTESIAN_POINT ( 'NONE',  ( 95.54126587499999346, 91.74999999863439371, -1.846868145590737864 ) ) ;
#10802=DIRECTION ( 'NONE',  ( -0.000000000000000000, 1.000000000000000000, -0.000000000000000000 ) ) ;
#10807=CARTESIAN_POINT ( 'NONE',  ( 98.15313185440925281, 92.62499999863439371, -4.458734124999994997 ) ) ;
#10819=LINE ( 'NONE', #6148, #25777 ) ;
#10829=CARTESIAN_POINT ( 'NONE',  ( 95.67376207875072680, 115.9545556584642867, -46.30000000000001137 ) ) ;
#10831=CARTESIAN_POINT ( 'NONE',  ( 97.50236033167492167, 102.3130555110000159, -50.72500000273119980 ) ) ;
#10841=CARTESIAN_POINT ( 'NONE',  ( 87.00000000000000000, 97.00000000000000000, -13.00000000000000533 ) ) ;
#10844=ORIENTED_EDGE ( 'NONE', *, *, #15372, .F. ) ;
#10850=CARTESIAN_POINT ( 'NONE',  ( 99.99999999999998579, 117.3602355696678501, -52.50000000000000000 ) ) ;
#10857=CARTESIAN_POINT ( 'NONE',  ( 102.0710678118654613, 93.68749999726881583, 4.999999999999983125 ) ) ;
#10876=CARTESIAN_POINT ( 'NONE',  ( 92.99999999999997158, 107.7255621263696952, -49.89999999999999858 ) ) ;
#10879=EDGE_LOOP ( 'NONE', ( #23994, #9748, #25111, #1727, #25426, #9874, #18552, #641 ) ) ;
#10887=CARTESIAN_POINT ( 'NONE',  ( 99.99999999999998579, 102.6397644303321215, -46.00000000546238255 ) ) ;
#10892=CARTESIAN_POINT ( 'NONE',  ( 93.46109445667491400, 114.7507929638356785, -53.32500000273119412 ) ) ;
#10895=CARTESIAN_POINT ( 'NONE',  ( 98.96446609406727646, 123.6500000021849530, 2.499999999999977796 ) ) ;
#10897=CARTESIAN_POINT ( 'NONE',  ( 107.0000000000000142, 110.0000000000000000, -47.00000000000000711 ) ) ;
#10899=VERTEX_POINT ( 'NONE', #21138 ) ;
#10900=CARTESIAN_POINT ( 'NONE',  ( 99.99999999999998579, 122.7500000010924879, -2.066987299999998751 ) ) ;
#10907=CARTESIAN_POINT ( 'NONE',  ( 95.00472066334982912, 116.8754121666685393, -51.42500000273118843 ) ) ;
#10928=CARTESIAN_POINT ( 'NONE',  ( 98.23223304703363112, 122.6000000021849559, -1.767766952966370209 ) ) ;
#10929=DIRECTION ( 'NONE',  ( 0.000000000000000000, -1.000000000000000000, 0.000000000000000000 ) ) ;
#10932=CARTESIAN_POINT ( 'NONE',  ( 107.0000000000000142, 110.0000000000000000, -53.50000000546238255 ) ) ;
#10936=CARTESIAN_POINT ( 'NONE',  ( 106.5389055433251002, 105.2492070361643215, -46.57500000273119412 ) ) ;
#10939=CARTESIAN_POINT ( 'NONE',  ( 93.00000000000000000, 110.0000000000000000, -44.50000000546237544 ) ) ;
#10940=CARTESIAN_POINT ( 'NONE',  ( 96.84719886470463734, 93.68749999863440792, -3.152801135295366208 ) ) ;
#10949=CARTESIAN_POINT ( 'NONE',  ( 95.54126587500000767, 93.81249999863440792, -7.484931351350258973E-15 ) ) ;
#10957=EDGE_CURVE ( 'NONE', #24722, #11653, #19565, .T. ) ;
#10972=CARTESIAN_POINT ( 'NONE',  ( 91.91746824999998466, 107.3738262389971538, -53.02500000273119696 ) ) ;
#10981=CARTESIAN_POINT ( 'NONE',  ( 99.99999999999998579, 90.25000000000000000, -4.999999999999997335 ) ) ;
#10989=CARTESIAN_POINT ( 'NONE',  ( 99.99999999999998579, 102.6397644303321215, -51.50000000000000711 ) ) ;
#10994=CARTESIAN_POINT ( 'NONE',  ( 103.5355339059327235, 91.99999999726880162, -3.535533905932738197 ) ) ;
#11011=ORIENTED_EDGE ( 'NONE', *, *, #25297, .F. ) ;
#11020=VERTEX_POINT ( 'NONE', #3473 ) ;
#11031=DIRECTION ( 'NONE',  ( 0.000000000000000000, -1.000000000000000000, 0.000000000000000000 ) ) ;
#11032=ADVANCED_FACE ( 'NONE', ( #16437 ), #3336, .T. ) ;
#11037=CARTESIAN_POINT ( 'NONE',  ( 98.53841926354351699, 123.0500000010924850, 1.461580736456455920 ) ) ;
#11042=DIRECTION ( 'NONE',  ( 0.000000000000000000, -1.000000000000000000, 0.000000000000000000 ) ) ;
#11045=CARTESIAN_POINT ( 'NONE',  ( 102.4976396683250925, 102.3130555110000159, -44.77500000273119696 ) ) ;
#11048=LINE ( 'NONE', #21914, #1216 ) ;
#11053=DIRECTION ( 'NONE',  ( -0.000000000000000000, 1.000000000000000000, -0.000000000000000000 ) ) ;
#11063=DIRECTION ( 'NONE',  ( -0.000000000000000000, -1.000000000000000000, -0.000000000000000000 ) ) ;
#11066=DIRECTION ( 'NONE',  ( 0.000000000000000000, 0.000000000000000000, 1.000000000000000000 ) ) ;
#11068=CARTESIAN_POINT ( 'NONE',  ( 102.0710678118654187, 93.18749999999998579, -5.000000000000031974 ) ) ;
#11070=ORIENTED_EDGE ( 'NONE', *, *, #12602, .T. ) ;
#11091=CARTESIAN_POINT ( 'NONE',  ( 99.99999999999998579, 90.25000000000000000, -4.999999999999997335 ) ) ;
#11096=CARTESIAN_POINT ( 'NONE',  ( 95.00000000000000000, 95.37499999726881583, -7.551217303480904118E-15 ) ) ;
#11098=EDGE_CURVE ( 'NONE', #26503, #13118, #24810, .T. ) ;
#11120=CARTESIAN_POINT ( 'NONE',  ( 95.67376207875072680, 115.9545556584642867, -50.80000000546237260 ) ) ;
#11125=LINE ( 'NONE', #17273, #9231 ) ;
#11129=CARTESIAN_POINT ( 'NONE',  ( 99.99999999999998579, 118.4984768113314004, -51.87500000273118417 ) ) ;
#11131=CARTESIAN_POINT ( 'NONE',  ( 102.4999999999999716, 123.7500000000000142, 1.035533905932722876 ) ) ;
#11133=CARTESIAN_POINT ( 'NONE',  ( 114.9999999999999858, 95.00000000000000000, 14.99999999999999289 ) ) ;
#11134=CARTESIAN_POINT ( 'NONE',  ( 96.46446609406726225, 95.49999999726881583, 3.535533905932723986 ) ) ;
#11143=CARTESIAN_POINT ( 'NONE',  ( 104.9999999999999858, 95.00000000000000000, -6.938893903907228378E-15 ) ) ;
#11148=AXIS2_PLACEMENT_3D ( 'NONE', #23749, #12885, #10338 ) ;
#11152=VERTEX_POINT ( 'NONE', #886 ) ;
#11169=CARTESIAN_POINT ( 'NONE',  ( 98.23223304703363112, 123.6000000021849416, 1.767766952966351557 ) ) ;
#11175=CARTESIAN_POINT ( 'NONE',  ( 101.0355339059327378, 123.2500000021849758, -2.499999999999997780 ) ) ;
#11182=CARTESIAN_POINT ( 'NONE',  ( 104.9952793366501851, 103.1245878333314323, -52.42500000273119554 ) ) ;
#11185=LINE ( 'NONE', #19904, #23939 ) ;
#11186=CARTESIAN_POINT ( 'NONE',  ( 101.7677669209684552, 123.0000000000000000, 1.767766984964258992 ) ) ;
#11218=CARTESIAN_POINT ( 'NONE',  ( 104.9952793366501709, 103.1245878333314465, -46.67500000273118843 ) ) ;
#11222=CARTESIAN_POINT ( 'NONE',  ( 102.2453236122039471, 123.0000000000000000, -1.108986377174830507 ) ) ;
#11232=CARTESIAN_POINT ( 'NONE',  ( 96.84719886470463734, 91.93749999863440792, 3.152801135295351997 ) ) ;
#11234=EDGE_CURVE ( 'NONE', #6002, #13072, #2741, .T. ) ;
#11240=ADVANCED_FACE ( 'NONE', ( #20961 ), #27656, .T. ) ;
#11257=CARTESIAN_POINT ( 'NONE',  ( 102.4976396683250925, 102.3130555110000159, -46.52500000273119696 ) ) ;
#11265=CARTESIAN_POINT ( 'NONE',  ( 99.99999999999998579, 123.1500000010924794, 2.066987299999980099 ) ) ;
#11273=CARTESIAN_POINT ( 'NONE',  ( 99.99999999999998579, 102.6397644303321215, -47.50000000000000711 ) ) ;
#11275=CARTESIAN_POINT ( 'NONE',  ( 101.0355339059327378, 123.9500000000000028, -2.499999999999997780 ) ) ;
#11279=CARTESIAN_POINT ( 'NONE',  ( 96.46446609406726225, 94.49999999726881583, 3.535533905932723986 ) ) ;
#11286=VERTEX_POINT ( 'NONE', #25374 ) ;
#11290=LINE ( 'NONE', #20011, #5161 ) ;
#11296=AXIS2_PLACEMENT_3D ( 'NONE', #23213, #18788, #1558 ) ;
#11298=ORIENTED_EDGE ( 'NONE', *, *, #14123, .T. ) ;
#11318=CARTESIAN_POINT ( 'NONE',  ( 98.23223304703363112, 122.6000000021849559, -1.767766952966370209 ) ) ;
#11320=CARTESIAN_POINT ( 'NONE',  ( 107.0000000000000142, 110.0000000000000000, -55.00000000000000711 ) ) ;
#11326=CARTESIAN_POINT ( 'NONE',  ( 95.00472066334982912, 116.8754121666685393, -45.42500000273119554 ) ) ;
#11328=CARTESIAN_POINT ( 'NONE',  ( 104.3262379212492590, 115.9545556584642867, -49.20000000546237828 ) ) ;
#11349=CARTESIAN_POINT ( 'NONE',  ( 108.0825317500000153, 110.0000000000000000, -54.37500000273119838 ) ) ;
#11350=CARTESIAN_POINT ( 'NONE',  ( 95.00000000000000000, 94.37499999726881583, -7.551217303480904118E-15 ) ) ;
#11363=CARTESIAN_POINT ( 'NONE',  ( 97.95371496370606224, 123.0000000000000000, -1.465530591365614477 ) ) ;
#11365=EDGE_LOOP ( 'NONE', ( #20900, #18799, #18302, #5653 ) ) ;
#11369=ORIENTED_EDGE ( 'NONE', *, *, #3399, .T. ) ;
#11371=VECTOR ( 'NONE', #16744, 1000.000000000000000 ) ;
#11374=CARTESIAN_POINT ( 'NONE',  ( 103.5355339059327235, 92.87500000000000000, 3.535533905932724874 ) ) ;
#11377=CIRCLE ( 'NONE', #25960, 5.000000000000004441 ) ;
#11390=DIRECTION ( 'NONE',  ( 1.000000000000000000, 0.000000000000000000, -5.782411586589357392E-17 ) ) ;
#11394=FACE_OUTER_BOUND ( 'NONE', #10710, .T. ) ;
#11398=DIRECTION ( 'NONE',  ( 0.000000000000000000, 0.000000000000000000, -1.000000000000000000 ) ) ;
#11400=CARTESIAN_POINT ( 'NONE',  ( 95.67376207875072680, 115.9545556584642867, -52.80000000546237260 ) ) ;
#11401=CARTESIAN_POINT ( 'NONE',  ( 98.15313185440925281, 90.87499999863439371, -4.458734124999994997 ) ) ;
#11415=ORIENTED_EDGE ( 'NONE', *, *, #28113, .F. ) ;
#11416=CARTESIAN_POINT ( 'NONE',  ( 95.67376207875072680, 104.0454443415356991, -45.70000000000000995 ) ) ;
#11418=CARTESIAN_POINT ( 'NONE',  ( 98.96446609406727646, 123.5499999999999972, 2.499999999999977796 ) ) ;
#11423=CARTESIAN_POINT ( 'NONE',  ( 95.00000000000000000, 95.37499999726881583, -7.551217303480904118E-15 ) ) ;
#11426=CARTESIAN_POINT ( 'NONE',  ( 91.91746824999999887, 110.0000000000000000, -49.37500000273119838 ) ) ;
#11435=ORIENTED_EDGE ( 'NONE', *, *, #5863, .T. ) ;
#11450=CARTESIAN_POINT ( 'NONE',  ( 99.99999999999998579, 110.0000000000000000, 15.00099999999999412 ) ) ;
#11453=CARTESIAN_POINT ( 'NONE',  ( 106.5389055433251002, 114.7507929638356785, -49.92500000273119554 ) ) ;
#11457=ORIENTED_EDGE ( 'NONE', *, *, #288, .T. ) ;
#11461=CARTESIAN_POINT ( 'NONE',  ( 102.4999999999999858, 123.1000000021849416, -9.847140817659276890E-15 ) ) ;
#11467=CARTESIAN_POINT ( 'NONE',  ( 101.8468681455907330, 92.49999999863442213, -4.458734124999994997 ) ) ;
#11472=CARTESIAN_POINT ( 'NONE',  ( 102.0710678118654613, 91.68749999726881583, 4.999999999999983125 ) ) ;
#11474=ORIENTED_EDGE ( 'NONE', *, *, #5547, .F. ) ;
#11475=AXIS2_PLACEMENT_3D ( 'NONE', #1127, #18065, #11922 ) ;
#11490=CARTESIAN_POINT ( 'NONE',  ( 101.0355339059327378, 124.4569999999781515, 2.499999999999977796 ) ) ;
#11491=PRESENTATION_STYLE_ASSIGNMENT (( #13633 ) ) ;
#11492=CARTESIAN_POINT ( 'NONE',  ( 97.92893218813448186, 94.18749999726881583, -4.999999999999963585 ) ) ;
#11505=CARTESIAN_POINT ( 'NONE',  ( 102.4976396683250925, 102.3130555110000159, -52.77500000273119696 ) ) ;
#11506=CARTESIAN_POINT ( 'NONE',  ( 98.84711739976860656, 122.9999999999999574, 2.236958744467042237 ) ) ;
#11513=CARTESIAN_POINT ( 'NONE',  ( 95.00000000000000000, 94.56250000000000000, 2.071067811865463959 ) ) ;
#11515=CARTESIAN_POINT ( 'NONE',  ( 99.99999999999998579, 92.25000000000000000, -4.999999999999997335 ) ) ;
#11519=ORIENTED_EDGE ( 'NONE', *, *, #3475, .T. ) ;
#11531=CARTESIAN_POINT ( 'NONE',  ( 95.54126587499999346, 91.74999999863439371, -1.846868145590737864 ) ) ;
#11536=VECTOR ( 'NONE', #19322, 1000.000000000000000 ) ;
#11539=CARTESIAN_POINT ( 'NONE',  ( 94.33688103937537051, 114.1144967660473242, -52.70000000546237828 ) ) ;
#11540=CARTESIAN_POINT ( 'NONE',  ( 103.1528011352953484, 92.43749999863440792, 3.152801135295352886 ) ) ;
#11547=ADVANCED_FACE ( 'NONE', ( #5535 ), #11667, .F. ) ;
#11555=CARTESIAN_POINT ( 'NONE',  ( 91.91746824999998466, 112.6261737610028320, -51.47500000273119980 ) ) ;
#11562=CARTESIAN_POINT ( 'NONE',  ( 104.4587341249999781, 93.56249999863440792, -6.938893903907228378E-15 ) ) ;
#11564=CARTESIAN_POINT ( 'NONE',  ( 99.99999999999998579, 118.4984768113314146, -51.87500000273119127 ) ) ;
#11572=EDGE_CURVE ( 'NONE', #14907, #26503, #18262, .T. ) ;
#11576=CARTESIAN_POINT ( 'NONE',  ( 98.15313185440923860, 91.87499999863439371, -4.458734124999994997 ) ) ;
#11586=EDGE_CURVE ( 'NONE', #18466, #3788, #22317, .T. ) ;
#11590=CARTESIAN_POINT ( 'NONE',  ( 95.00000000000000000, 91.31249999726880162, -2.071067811865479058 ) ) ;
#11593=CARTESIAN_POINT ( 'NONE',  ( 99.99999999999998579, 118.4984768113314146, -45.62500000273119127 ) ) ;
#11595=CARTESIAN_POINT ( 'NONE',  ( 99.99999999999998579, 90.00000000000000000, -6.938893903907228378E-15 ) ) ;
#11606=CARTESIAN_POINT ( 'NONE',  ( 91.91746824999999887, 110.0000000000000000, -47.12500000273119838 ) ) ;
#11608=AXIS2_PLACEMENT_3D ( 'NONE', #26831, #26396, #5158 ) ;
#11609=DIRECTION ( 'NONE',  ( 0.000000000000000000, -1.000000000000000000, 0.000000000000000000 ) ) ;
#11622=ORIENTED_EDGE ( 'NONE', *, *, #21676, .T. ) ;
#11632=CARTESIAN_POINT ( 'NONE',  ( 102.4999999999999858, 124.6069999999781572, -9.847140817659276890E-15 ) ) ;
#11648=AXIS2_PLACEMENT_3D ( 'NONE', #21966, #13529, #22531 ) ;
#11650=CARTESIAN_POINT ( 'NONE',  ( 102.0669872999999939, 124.2000000010924907, -0.8561741729129507261 ) ) ;
#11653=VERTEX_POINT ( 'NONE', #4931 ) ;
#11658=CARTESIAN_POINT ( 'NONE',  ( 104.9999999999999716, 92.06249999999998579, -2.071067811865478170 ) ) ;
#11667=( BOUNDED_SURFACE ( )  B_SPLINE_SURFACE ( 1, 2, ( 
 ( #26634, #18210, #16350, #5391, #18353, #25050, #7511, #2957, #20071, #15777, #11632, #549, #13631, #11490, #20355, #693, #9510, #7221, #15910, #7364, #24767, #5248, #13913, #11917, #22640, #27061, #21329, #21054, #18771, #10059, #14479, #1674, #20777, #9920, #8209, #25735, #1538, #10330, #27612, #23196, #3531, #16629, #12187, #10475, #27476 ),
 ( #5809, #17032, #27749, #3673, #16898, #12335, #1399, #3803, #10190, #27885, #18901, #7932, #19183, #20916, #14746, #6219, #25183, #12605, #1810, #8069, #19037, #14336, #16764, #3946, #8347, #25322, #25466, #12463, #16488, #5944, #14612, #25596, #6080, #5671, #23329, #23468, #23054, #21188, #22919, #27341, #3380, #12051, #1259, #18637, #7800 ),
 ( #225, #17748, #13018, #12879, #26451, #6626, #14887, #13304, #21608, #19466, #23603, #17601, #87, #17458, #6489, #10895, #11169, #15455, #26306, #8769, #4084, #12747, #22031, #28025, #24168, #4504, #1948, #13161, #8490, #4220, #10617, #8910, #6769, #4361, #21756, #2086, #21472, #25882, #6351, #17321, #4645, #2507, #15163, #19323, #372 ) ),
 .UNSPECIFIED., .F., .F., .F. ) 
 B_SPLINE_SURFACE_WITH_KNOTS ( ( 2, 1, 2 ),
 ( 3, 2, 2, 2, 2, 2, 2, 2, 2, 2, 2, 2, 2, 2, 2, 2, 2, 2, 2, 2, 2, 2, 3 ),
 ( -0.01000000000000000021, 0.000000000000000000, 1.000000000000000000 ),
 ( -0.008333333333333333218, 0.000000000000000000, 0.04166666666666666435, 0.08333333333333332871, 0.1250000000000000000, 0.1666666666666666574, 0.2083333333333333426, 0.2500000000000000000, 0.2916666666666666852, 0.3333333333333333148, 0.3750000000000000000, 0.4166666666666666852, 0.4583333333333333148, 0.5000000000000000000, 0.5416666666666666297, 0.5833333333333333703, 0.6250000000000000000, 0.6666666666666666297, 0.7083333333333333703, 0.7500000000000000000, 0.7916666666666666297, 0.8333333333333333703, 0.8417499999999999982 ),
 .UNSPECIFIED. ) 
 GEOMETRIC_REPRESENTATION_ITEM ( )  RATIONAL_B_SPLINE_SURFACE ( (
 ( 1.000000000000000000, 1.000000000000000000, 1.000000000000000000, 0.9238795325112867385, 1.000000000000000000, 0.9238795325112867385, 1.000000000000000000, 0.9238795325112867385, 1.000000000000000000, 0.9238795325112867385, 1.000000000000000000, 0.9238795325112867385, 1.000000000000000000, 0.9238795325112867385, 1.000000000000000000, 0.9238795325112867385, 1.000000000000000000, 0.9238795325112867385, 1.000000000000000000, 0.9238795325112867385, 1.000000000000000000, 0.9238795325112867385, 1.000000000000000000, 0.9238795325112867385, 1.000000000000000000, 0.9238795325112867385, 1.000000000000000000, 0.9238795325112867385, 1.000000000000000000, 0.9238795325112867385, 1.000000000000000000, 0.9238795325112867385, 1.000000000000000000, 0.9238795325112867385, 1.000000000000000000, 0.9238795325112867385, 1.000000000000000000, 0.9238795325112867385, 1.000000000000000000, 0.9238795325112867385, 1.000000000000000000, 0.9238795325112867385, 1.000000000000000000, 1.000000000000000000, 1.000000000000000000),
 ( 1.000000000000000000, 1.000000000000000000, 1.000000000000000000, 0.9238795325112867385, 1.000000000000000000, 0.9238795325112867385, 1.000000000000000000, 0.9238795325112867385, 1.000000000000000000, 0.9238795325112867385, 1.000000000000000000, 0.9238795325112867385, 1.000000000000000000, 0.9238795325112867385, 1.000000000000000000, 0.9238795325112867385, 1.000000000000000000, 0.9238795325112867385, 1.000000000000000000, 0.9238795325112867385, 1.000000000000000000, 0.9238795325112867385, 1.000000000000000000, 0.9238795325112867385, 1.000000000000000000, 0.9238795325112867385, 1.000000000000000000, 0.9238795325112867385, 1.000000000000000000, 0.9238795325112867385, 1.000000000000000000, 0.9238795325112867385, 1.000000000000000000, 0.9238795325112867385, 1.000000000000000000, 0.9238795325112867385, 1.000000000000000000, 0.9238795325112867385, 1.000000000000000000, 0.9238795325112867385, 1.000000000000000000, 0.9238795325112867385, 1.000000000000000000, 1.000000000000000000, 1.000000000000000000),
 ( 1.000000000000000000, 1.000000000000000000, 1.000000000000000000, 0.9238795325112867385, 1.000000000000000000, 0.9238795325112867385, 1.000000000000000000, 0.9238795325112867385, 1.000000000000000000, 0.9238795325112867385, 1.000000000000000000, 0.9238795325112867385, 1.000000000000000000, 0.9238795325112867385, 1.000000000000000000, 0.9238795325112867385, 1.000000000000000000, 0.9238795325112867385, 1.000000000000000000, 0.9238795325112867385, 1.000000000000000000, 0.9238795325112867385, 1.000000000000000000, 0.9238795325112867385, 1.000000000000000000, 0.9238795325112867385, 1.000000000000000000, 0.9238795325112867385, 1.000000000000000000, 0.9238795325112867385, 1.000000000000000000, 0.9238795325112867385, 1.000000000000000000, 0.9238795325112867385, 1.000000000000000000, 0.9238795325112867385, 1.000000000000000000, 0.9238795325112867385, 1.000000000000000000, 0.9238795325112867385, 1.000000000000000000, 0.9238795325112867385, 1.000000000000000000, 1.000000000000000000, 1.000000000000000000) ) ) 
 REPRESENTATION_ITEM ( '' )  SURFACE ( )  );
#11670=AXIS2_PLACEMENT_3D ( 'NONE', #19693, #6444, #465 ) ;
#11682=CARTESIAN_POINT ( 'NONE',  ( 99.99999999999998579, 101.5015231886685854, -46.62500000273119838 ) ) ;
#11696=CARTESIAN_POINT ( 'NONE',  ( 104.9952793366501851, 116.8754121666685393, -54.07500000273119412 ) ) ;
#11704=CARTESIAN_POINT ( 'NONE',  ( 99.99999999999998579, 92.81249999863440792, -4.458734124999994997 ) ) ;
#11708=CARTESIAN_POINT ( 'NONE',  ( 108.0825317500000011, 107.3738262389971680, -52.47500000273119269 ) ) ;
#11709=EDGE_CURVE ( 'NONE', #3863, #7002, #18318, .T. ) ;
#11710=CARTESIAN_POINT ( 'NONE',  ( 84.99999999999998579, 120.0000000000000000, -15.00000000000000533 ) ) ;
#11714=PRODUCT ( 'vaccum generator', 'vaccum generator', '', ( #1857 ) ) ;
#11715=CARTESIAN_POINT ( 'NONE',  ( 101.0355339059327235, 124.4499999999999744, 2.499999999999974687 ) ) ;
#11725=VERTEX_POINT ( 'NONE', #14021 ) ;
#11730=ORIENTED_EDGE ( 'NONE', *, *, #22425, .F. ) ;
#11733=FACE_OUTER_BOUND ( 'NONE', #10879, .T. ) ;
#11735=CARTESIAN_POINT ( 'NONE',  ( 108.0825317500000011, 107.3738262389971680, -50.22500000273118559 ) ) ;
#11736=DIRECTION ( 'NONE',  ( 0.000000000000000000, 0.000000000000000000, 1.000000000000000000 ) ) ;
#11737=ADVANCED_FACE ( 'NONE', ( #1087 ), #15879, .T. ) ;
#11742=SURFACE_STYLE_USAGE ( .BOTH. , #27030 ) ;
#11747=LINE ( 'NONE', #16176, #9409 ) ;
#11752=CARTESIAN_POINT ( 'NONE',  ( 103.5355339059327235, 91.74999999726880162, 3.535533905932724874 ) ) ;
#11753=CARTESIAN_POINT ( 'NONE',  ( 102.4976396683250925, 117.6869444889999841, -47.72500000273119269 ) ) ;
#11789=CARTESIAN_POINT ( 'NONE',  ( 112.9999999999999858, 102.0000000000000142, -15.00000000000000711 ) ) ;
#11791=CARTESIAN_POINT ( 'NONE',  ( 106.5389055433251002, 114.7507929638356785, -54.17500000273119554 ) ) ;
#11799=CARTESIAN_POINT ( 'NONE',  ( 105.6631189606246295, 114.1144967660473242, -50.80000000000000426 ) ) ;
#11801=CARTESIAN_POINT ( 'NONE',  ( 97.92893218813459555, 94.68750000000001421, 5.000000000000046185 ) ) ;
#11803=CARTESIAN_POINT ( 'NONE',  ( 97.92893218813452449, 94.31250000000001421, -4.999999999999997335 ) ) ;
#11811=VECTOR ( 'NONE', #18573, 1000.000000000000000 ) ;
#11813=ORIENTED_EDGE ( 'NONE', *, *, #10331, .F. ) ;
#11821=CARTESIAN_POINT ( 'NONE',  ( 95.54126587500000767, 90.81249999863440792, -7.484931351350258973E-15 ) ) ;
#11828=CARTESIAN_POINT ( 'NONE',  ( 97.50236033167492167, 102.3130555110000159, -44.72500000273119980 ) ) ;
#11829=CARTESIAN_POINT ( 'NONE',  ( 104.4587341249999923, 90.62499999863439371, -1.846868145590737198 ) ) ;
#11833=ORIENTED_EDGE ( 'NONE', *, *, #12749, .T. ) ;
#11839=VERTEX_POINT ( 'NONE', #19005 ) ;
#11844=CARTESIAN_POINT ( 'NONE',  ( 108.0825317500000011, 112.6261737610028320, -50.27500000273119696 ) ) ;
#11851=CARTESIAN_POINT ( 'NONE',  ( 99.99999999999998579, 91.31249999863440792, 4.458734124999981674 ) ) ;
#11852=LINE ( 'NONE', #25540, #11811 ) ;
#11853=CARTESIAN_POINT ( 'NONE',  ( 97.50236033167492167, 102.3130555110000159, -50.97500000273119980 ) ) ;
#11863=CARTESIAN_POINT ( 'NONE',  ( 103.1528011352953484, 91.43749999863440792, 3.152801135295352886 ) ) ;
#11874=DIRECTION ( 'NONE',  ( -0.8660254037844418162, 0.4999999999999947264, -0.000000000000000000 ) ) ;
#11883=ORIENTED_EDGE ( 'NONE', *, *, #19952, .F. ) ;
#11891=CARTESIAN_POINT ( 'NONE',  ( 91.91746824999998466, 107.3738262389971538, -47.02500000273118275 ) ) ;
#11892=CARTESIAN_POINT ( 'NONE',  ( 101.0355339059327235, 123.1500000000000057, -2.500000000000001776 ) ) ;
#11898=VERTEX_POINT ( 'NONE', #9893 ) ;
#11906=EDGE_CURVE ( 'NONE', #18097, #6897, #27436, .T. ) ;
#11910=DIRECTION ( 'NONE',  ( 0.000000000000000000, -1.000000000000000000, 0.000000000000000000 ) ) ;
#11916=CARTESIAN_POINT ( 'NONE',  ( 99.99999999999998579, 124.3999999999999915, 2.499999999999978684 ) ) ;
#11917=CARTESIAN_POINT ( 'NONE',  ( 101.0355339059327378, 123.9569999999781515, -2.499999999999997780 ) ) ;
#11919=SURFACE_STYLE_FILL_AREA ( #3252 ) ;
#11921=CARTESIAN_POINT ( 'NONE',  ( 112.9999999999999858, 97.00000000000000000, 12.99999999999999289 ) ) ;
#11922=DIRECTION ( 'NONE',  ( 1.000000000000000000, 0.000000000000000000, -0.000000000000000000 ) ) ;
#11930=DIRECTION ( 'NONE',  ( 0.000000000000000000, 4.625929269271485914E-16, 1.000000000000000000 ) ) ;
#11934=ORIENTED_EDGE ( 'NONE', *, *, #4292, .T. ) ;
#11941=CARTESIAN_POINT ( 'NONE',  ( 102.1631189606246295, 116.6573956140660897, -50.60000000000000853 ) ) ;
#11944=CARTESIAN_POINT ( 'NONE',  ( 104.9999999999999716, 92.93749999999998579, 2.071067811865467956 ) ) ;
#11950=EDGE_CURVE ( 'NONE', #20336, #10673, #5637, .T. ) ;
#11959=DIRECTION ( 'NONE',  ( 0.8660254037844392627, -0.000000000000000000, -0.4999999999999987788 ) ) ;
#11969=CARTESIAN_POINT ( 'NONE',  ( 105.6631189606246295, 105.8855032339526758, -49.70000000546237828 ) ) ;
#11974=CIRCLE ( 'NONE', #18800, 7.000000000000006217 ) ;
#11980=ORIENTED_EDGE ( 'NONE', *, *, #27445, .T. ) ;
#11984=CARTESIAN_POINT ( 'NONE',  ( 108.0825317500000011, 107.3738262389971538, -50.47500000273118559 ) ) ;
#11987=FACE_OUTER_BOUND ( 'NONE', #8546, .T. ) ;
#11992=CARTESIAN_POINT ( 'NONE',  ( 95.54126587499999346, 91.12499999863439371, 1.846868145590722543 ) ) ;
#11997=CARTESIAN_POINT ( 'NONE',  ( 99.99999999999998579, 97.00000000000000000, -2.999999999999996447 ) ) ;
#12003=CARTESIAN_POINT ( 'NONE',  ( 96.84719886470463734, 92.93749999863440792, -3.152801135295366208 ) ) ;
#12011=CARTESIAN_POINT ( 'NONE',  ( 101.4615807364564546, 122.8500000010924680, -1.461580736456474794 ) ) ;
#12013=ORIENTED_EDGE ( 'NONE', *, *, #24846, .F. ) ;
#12019=DIRECTION ( 'NONE',  ( -0.000000000000000000, 1.000000000000000000, -0.000000000000000000 ) ) ;
#12023=ADVANCED_FACE ( 'NONE', ( #25433, #3774 ), #27172, .F. ) ;
#12024=( NAMED_UNIT ( * ) PLANE_ANGLE_UNIT ( ) SI_UNIT ( $, .RADIAN. ) );
#12027=CARTESIAN_POINT ( 'NONE',  ( 97.92893218813455292, 92.56249999726880162, 5.000000000000003553 ) ) ;
#12051=CARTESIAN_POINT ( 'NONE',  ( 102.4999999999999716, 123.0500000000000114, -1.035533905932742638 ) ) ;
#12068=CARTESIAN_POINT ( 'NONE',  ( 108.0825317500000011, 107.3738262389971538, -48.47500000273118559 ) ) ;
#12070=CARTESIAN_POINT ( 'NONE',  ( 102.0669872999999939, 123.4000000010924936, -0.8561741729129507261 ) ) ;
#12093=CARTESIAN_POINT ( 'NONE',  ( 101.8468681455907330, 92.12499999863440792, 4.458734124999980786 ) ) ;
#12101=CARTESIAN_POINT ( 'NONE',  ( 105.6631189606246295, 114.1144967660473242, -51.30000000546237970 ) ) ;
#12102=CARTESIAN_POINT ( 'NONE',  ( 103.1528011352953484, 95.43749999863440792, 3.152801135295352886 ) ) ;
#12118=CARTESIAN_POINT ( 'NONE',  ( 102.4976396683250925, 117.6869444889999841, -47.97500000273119269 ) ) ;
#12120=DIRECTION ( 'NONE',  ( 5.782411586589357392E-17, -0.000000000000000000, 1.000000000000000000 ) ) ;
#12125=CARTESIAN_POINT ( 'NONE',  ( 101.8468681455907330, 92.74999999863439371, -4.458734124999994997 ) ) ;
#12139=CARTESIAN_POINT ( 'NONE',  ( 99.99999999999998579, 93.81249999863440792, -4.458734124999994997 ) ) ;
#12150=CARTESIAN_POINT ( 'NONE',  ( 104.3262379212492590, 115.9545556584642867, -54.70000000000000995 ) ) ;
#12154=CARTESIAN_POINT ( 'NONE',  ( 95.67376207875072680, 115.9545556584642867, -44.80000000546236549 ) ) ;
#12162=CARTESIAN_POINT ( 'NONE',  ( 95.00000000000000000, 92.37499999726880162, -7.551217303480904118E-15 ) ) ;
#12171=ORIENTED_EDGE ( 'NONE', *, *, #4782, .F. ) ;
#12187=CARTESIAN_POINT ( 'NONE',  ( 102.4999999999999858, 123.0069999999781487, -9.847140817659276890E-15 ) ) ;
#12188=VECTOR ( 'NONE', #2277, 1000.000000000000000 ) ;
#12203=CARTESIAN_POINT ( 'NONE',  ( 93.46109445667491400, 105.2492070361643215, -49.17500000273119554 ) ) ;
#12205=CARTESIAN_POINT ( 'NONE',  ( 99.14382582708707048, 123.0000000010925021, -2.066987299999999195 ) ) ;
#12215=AXIS2_PLACEMENT_3D ( 'NONE', #3175, #24973, #1192 ) ;
#12229=CARTESIAN_POINT ( 'NONE',  ( 95.54126587499999346, 92.87499999863439371, 1.846868145590722543 ) ) ;
#12237=CARTESIAN_POINT ( 'NONE',  ( 94.33688103937537051, 105.8855032339526758, -46.30000000546237970 ) ) ;
#12239=CARTESIAN_POINT ( 'NONE',  ( 98.15313185440925281, 90.99999999863439371, 4.458734124999979898 ) ) ;
#12240=CIRCLE ( 'NONE', #25911, 4.999999999999989342 ) ;
#12247=CARTESIAN_POINT ( 'NONE',  ( 84.99999999999998579, 95.00000000000000000, 14.99999999999999467 ) ) ;
#12253=EDGE_CURVE ( 'NONE', #4950, #11, #17428, .T. ) ;
#12255=CARTESIAN_POINT ( 'NONE',  ( 91.91746824999999887, 110.0000000000000000, -47.37500000273119838 ) ) ;
#12259=VECTOR ( 'NONE', #20125, 1000.000000000000000 ) ;
#12261=CARTESIAN_POINT ( 'NONE',  ( 99.99999999999998579, 101.5015231886685712, -44.62500000273119838 ) ) ;
#12278=CARTESIAN_POINT ( 'NONE',  ( 101.8468681455907330, 94.37499999863440792, 4.458734124999980786 ) ) ;
#12279=DIRECTION ( 'NONE',  ( -5.782411586589357392E-17, 0.000000000000000000, -1.000000000000000000 ) ) ;
#12287=CARTESIAN_POINT ( 'NONE',  ( 102.0669872999999797, 122.7500000010924737, -9.794112055954760458E-15 ) ) ;
#12290=CARTESIAN_POINT ( 'NONE',  ( 96.46446609406726225, 92.37500000000000000, -3.535533905932738197 ) ) ;
#12291=AXIS2_PLACEMENT_3D ( 'NONE', #9063, #26025, #25891 ) ;
#12292=EDGE_CURVE ( 'NONE', #17147, #23013, #11852, .T. ) ;
#12295=ADVANCED_FACE ( 'NONE', ( #1611 ), #18978, .F. ) ;
#12301=AXIS2_PLACEMENT_3D ( 'NONE', #26821, #592, #26965 ) ;
#12304=ADVANCED_FACE ( 'NONE', ( #10269 ), #3182, .F. ) ;
#12309=VECTOR ( 'NONE', #7764, 1000.000000000000000 ) ;
#12314=ORIENTED_EDGE ( 'NONE', *, *, #24484, .T. ) ;
#12335=CARTESIAN_POINT ( 'NONE',  ( 98.96446609406727646, 124.8500000000000085, -2.499999999999997780 ) ) ;
#12340=CARTESIAN_POINT ( 'NONE',  ( 99.99999999999998579, 123.3000000021849587, -2.499999999999997780 ) ) ;
#12341=ORIENTED_EDGE ( 'NONE', *, *, #12292, .F. ) ;
#12342=CARTESIAN_POINT ( 'NONE',  ( 98.96446609406727646, 124.1500000021849672, -2.499999999999997780 ) ) ;
#12349=CARTESIAN_POINT ( 'NONE',  ( 106.5389055433251002, 114.7507929638356785, -50.17500000273119554 ) ) ;
#12352=CYLINDRICAL_SURFACE ( 'NONE', #11296, 2.499999999999995115 ) ;
#12365=CARTESIAN_POINT ( 'NONE',  ( 94.33688103937537051, 114.1144967660473242, -52.20000000000000995 ) ) ;
#12369=DIRECTION ( 'NONE',  ( 0.000000000000000000, 1.000000000000000000, 0.000000000000000000 ) ) ;
#12382=CARTESIAN_POINT ( 'NONE',  ( 107.0000000000000142, 107.7255621263696526, -47.60000000546237686 ) ) ;
#12383=CARTESIAN_POINT ( 'NONE',  ( 96.84719886470463734, 93.93749999863440792, -3.152801135295366208 ) ) ;
#12387=ORIENTED_EDGE ( 'NONE', *, *, #3399, .F. ) ;
#12393=ORIENTED_EDGE ( 'NONE', *, *, #19253, .F. ) ;
#12394=CARTESIAN_POINT ( 'NONE',  ( 108.0825317500000011, 112.6261737610028320, -46.27500000273120406 ) ) ;
#12398=CARTESIAN_POINT ( 'NONE',  ( 99.99999999999998579, 118.4984768113314146, -49.62500000273118417 ) ) ;
#12405=CARTESIAN_POINT ( 'NONE',  ( 107.0000000000000142, 112.2744378736303190, -46.90000000000001279 ) ) ;
#12406=( BOUNDED_CURVE ( )  B_SPLINE_CURVE ( 2, ( #16767, #25737, #8211, #6221, #14614, #18904, #1540, #25598, #17034, #14889, #23331, #16900, #27751, #14748, #3805, #10192, #27615, #8071, #25468, #12465, #21334, #12608, #21190, #23470, #6082, #3948, #27887, #1676, #10333, #1813, #19040, #10477, #23607, #10146, #14573, #14011, #1077, #18309, #12011, #3201, #12287 ),
 .UNSPECIFIED., .F., .F. ) 
 B_SPLINE_CURVE_WITH_KNOTS ( ( 3, 2, 2, 2, 2, 2, 2, 2, 2, 2, 2, 2, 2, 2, 2, 2, 2, 2, 2, 2, 3 ),
 ( 0.000000000000000000, 0.04166666666666666435, 0.08333333333333332871, 0.1250000000000000000, 0.1666666666666666574, 0.2083333333333333426, 0.2500000000000000000, 0.2916666666666666852, 0.3333333333333333148, 0.3750000000000000000, 0.4166666666666666852, 0.4583333333333332593, 0.5000000000000000000, 0.5416666666666666297, 0.5833333333333333703, 0.6250000000000000000, 0.6666666666666666297, 0.7083333333333333703, 0.7500000000000000000, 0.7916666666666666297, 0.8333333333333333703 ),
 .UNSPECIFIED. ) 
 CURVE ( )  GEOMETRIC_REPRESENTATION_ITEM ( )  RATIONAL_B_SPLINE_CURVE ( ( 1.000000000000000000, 0.9238795325112867385, 1.000000000000000000, 0.9238795325112867385, 1.000000000000000000, 0.9238795325112867385, 1.000000000000000000, 0.9238795325112867385, 1.000000000000000000, 0.9238795325112867385, 1.000000000000000000, 0.9238795325112867385, 1.000000000000000000, 0.9238795325112867385, 1.000000000000000000, 0.9238795325112867385, 1.000000000000000000, 0.9238795325112867385, 1.000000000000000000, 0.9238795325112867385, 1.000000000000000000, 0.9238795325112867385, 1.000000000000000000, 0.9238795325112867385, 1.000000000000000000, 0.9238795325112867385, 1.000000000000000000, 0.9238795325112867385, 1.000000000000000000, 0.9238795325112867385, 1.000000000000000000, 0.9238795325112867385, 1.000000000000000000, 0.9238795325112867385, 1.000000000000000000, 0.9238795325112867385, 1.000000000000000000, 0.9238795325112867385, 1.000000000000000000, 0.9238795325112867385, 1.000000000000000000 ) ) 
 REPRESENTATION_ITEM ( '' )  );
#12415=VERTEX_POINT ( 'NONE', #27276 ) ;
#12416=ADVANCED_FACE ( 'NONE', ( #1055 ), #3743, .T. ) ;
#12419=DIRECTION ( 'NONE',  ( 1.000000000000000000, 0.000000000000000000, -5.782411586589357392E-17 ) ) ;
#12426=ADVANCED_FACE ( 'NONE', ( #5464 ), #14133, .T. ) ;
#12430=DIRECTION ( 'NONE',  ( -1.000000000000000000, 0.000000000000000000, 0.000000000000000000 ) ) ;
#12436=CARTESIAN_POINT ( 'NONE',  ( 102.0710678118654613, 90.81249999999995737, 4.999999999999974243 ) ) ;
#12441=FACE_OUTER_BOUND ( 'NONE', #10248, .T. ) ;
#12459=CARTESIAN_POINT ( 'NONE',  ( 99.99999999999998579, 93.12499999726881583, -4.999999999999997335 ) ) ;
#12463=CARTESIAN_POINT ( 'NONE',  ( 102.4999999999999716, 123.7500000000000142, 1.035533905932722876 ) ) ;
#12465=CARTESIAN_POINT ( 'NONE',  ( 99.14382582708708469, 123.8000000010924566, -2.066987299999998751 ) ) ;
#12466=VECTOR ( 'NONE', #26545, 1000.000000000000000 ) ;
#12478=CARTESIAN_POINT ( 'NONE',  ( 99.99999999999998579, 101.5015231886685854, -48.87500000273119838 ) ) ;
#12480=CARTESIAN_POINT ( 'NONE',  ( 99.14382582708707048, 123.8000000010924850, -2.066987299999999195 ) ) ;
#12486=CARTESIAN_POINT ( 'NONE',  ( 93.00000000000002842, 112.2744378736303759, -50.10000000000000853 ) ) ;
#12500=CYLINDRICAL_SURFACE ( 'NONE', #7327, 2.499999999999995115 ) ;
#12502=CARTESIAN_POINT ( 'NONE',  ( 103.1528011352953484, 93.18749999863440792, 3.152801135295352886 ) ) ;
#12512=CARTESIAN_POINT ( 'NONE',  ( 99.99999999999998579, 90.00000000000000000, -4.999999999999996447 ) ) ;
#12513=CARTESIAN_POINT ( 'NONE',  ( 98.15313185440925281, 94.24999999863439371, 4.458734124999979898 ) ) ;
#12516=ORIENTED_EDGE ( 'NONE', *, *, #20742, .F. ) ;
#12519=AXIS2_PLACEMENT_3D ( 'NONE', #20258, #744, #17693 ) ;
#12528=ORIENTED_EDGE ( 'NONE', *, *, #2192, .T. ) ;
#12541=DIRECTION ( 'NONE',  ( 1.000000000000000000, 0.000000000000000000, 0.000000000000000000 ) ) ;
#12550=CARTESIAN_POINT ( 'NONE',  ( 99.99999999999998579, 90.00000000000000000, 4.999999999999983125 ) ) ;
#12553=CARTESIAN_POINT ( 'NONE',  ( 98.15313185440923860, 94.87499999863440792, -4.458734124999994997 ) ) ;
#12556=CARTESIAN_POINT ( 'NONE',  ( 99.99999999999998579, 93.75000000000000000, 4.999999999999984013 ) ) ;
#12565=CARTESIAN_POINT ( 'NONE',  ( 99.14382582708707048, 123.8000000010924850, -2.066987299999999195 ) ) ;
#12579=CARTESIAN_POINT ( 'NONE',  ( 102.0669872999999797, 122.6166666677591337, -9.794112055954758880E-15 ) ) ;
#12583=CARTESIAN_POINT ( 'NONE',  ( 99.99999999999998579, 94.12499999726881583, -4.999999999999997335 ) ) ;
#12602=EDGE_CURVE ( 'NONE', #23799, #20591, #8420, .T. ) ;
#12605=CARTESIAN_POINT ( 'NONE',  ( 97.50000000000000000, 124.2500000000000000, 1.035533905932725096 ) ) ;
#12608=CARTESIAN_POINT ( 'NONE',  ( 100.8561741729129295, 123.7000000010924765, -2.066987299999998751 ) ) ;
#12611=ORIENTED_EDGE ( 'NONE', *, *, #25541, .F. ) ;
#12614=VECTOR ( 'NONE', #1514, 1000.000000000000000 ) ;
#12621=CARTESIAN_POINT ( 'NONE',  ( 99.99999999999998579, 118.4984768113314004, -49.87500000273118417 ) ) ;
#12623=VERTEX_POINT ( 'NONE', #6430 ) ;
#12624=CARTESIAN_POINT ( 'NONE',  ( 99.99999999999998579, 124.1500000010924651, 2.066987299999980099 ) ) ;
#12628=EDGE_LOOP ( 'NONE', ( #24231, #196 ) ) ;
#12630=PLANE ( 'NONE',  #14407 ) ;
#12640=EDGE_CURVE ( 'NONE', #26108, #11, #19122, .T. ) ;
#12644=EDGE_CURVE ( 'NONE', #613, #2287, #4298, .T. ) ;
#12648=CARTESIAN_POINT ( 'NONE',  ( 104.9999999999999858, 95.87499999726881583, -6.938893903907228378E-15 ) ) ;
#12659=CARTESIAN_POINT ( 'NONE',  ( 101.8468681455907330, 93.37499999863439371, 4.458734124999979898 ) ) ;
#12669=ORIENTED_EDGE ( 'NONE', *, *, #21706, .F. ) ;
#12675=ORIENTED_EDGE ( 'NONE', *, *, #25532, .F. ) ;
#12691=CARTESIAN_POINT ( 'NONE',  ( 104.9952793366501851, 116.8754121666685393, -51.82500000273120122 ) ) ;
#12699=( BOUNDED_CURVE ( )  B_SPLINE_CURVE ( 2, ( #16002, #13427, #6891, #15577, #15722, #26719, #18299, #3192, #22155, #22297, #26432, #20157, #638, #2907, #11863, #2633, #4765, #9311, #20586, #20445, #7165, #11576, #20296, #7313, #783, #5337, #9453, #7454, #18153, #13858, #27007, #16148, #14003, #16720, #18583, #21005, #16575, #10012, #12003, #3618, #5899, #18446, #25268, #23143, #3333, #18991, #18721, #10282, #14699, #14146, #1211, #27153, #12139, #20727, #5758, #23418, #22865, #7605, #9877, #3891, #14568, #12278, #27419, #1762, #27560, #23002, #16855, #14286, #27700, #12553, #7882, #27288, #7745, #8163, #25417, #16433, #1485, #14426, #10140, #25131, #18852 ),
 .UNSPECIFIED., .F., .F. ) 
 B_SPLINE_CURVE_WITH_KNOTS ( ( 3, 2, 2, 2, 2, 2, 2, 2, 2, 2, 2, 2, 2, 2, 2, 2, 2, 2, 2, 2, 2, 2, 2, 2, 2, 2, 2, 2, 2, 2, 2, 2, 2, 2, 2, 2, 2, 2, 2, 2, 3 ),
 ( 0.000000000000000000, 0.02500000000000000139, 0.05000000000000000278, 0.07499999999999999722, 0.1000000000000000056, 0.1250000000000000000, 0.1499999999999999944, 0.1749999999999999889, 0.2000000000000000111, 0.2250000000000000056, 0.2500000000000000000, 0.2750000000000000222, 0.2999999999999999889, 0.3250000000000000111, 0.3499999999999999778, 0.3750000000000000000, 0.4000000000000000222, 0.4249999999999999889, 0.4500000000000000111, 0.4749999999999999778, 0.5000000000000000000, 0.5250000000000000222, 0.5500000000000000444, 0.5749999999999999556, 0.5999999999999999778, 0.6250000000000000000, 0.6500000000000000222, 0.6750000000000000444, 0.6999999999999999556, 0.7249999999999999778, 0.7500000000000000000, 0.7750000000000000222, 0.8000000000000000444, 0.8249999999999999556, 0.8499999999999999778, 0.8750000000000000000, 0.9000000000000000222, 0.9250000000000000444, 0.9499999999999999556, 0.9749999999999999778, 1.000000000000000000 ),
 .UNSPECIFIED. ) 
 CURVE ( )  GEOMETRIC_REPRESENTATION_ITEM ( )  RATIONAL_B_SPLINE_CURVE ( ( 1.000000000000000000, 0.9238795325112867385, 1.000000000000000000, 0.9238795325112867385, 1.000000000000000000, 0.9238795325112867385, 1.000000000000000000, 0.9238795325112867385, 1.000000000000000000, 0.9238795325112867385, 1.000000000000000000, 0.9238795325112867385, 1.000000000000000000, 0.9238795325112867385, 1.000000000000000000, 0.9238795325112867385, 1.000000000000000000, 0.9238795325112867385, 1.000000000000000000, 0.9238795325112867385, 1.000000000000000000, 0.9238795325112867385, 1.000000000000000000, 0.9238795325112867385, 1.000000000000000000, 0.9238795325112867385, 1.000000000000000000, 0.9238795325112867385, 1.000000000000000000, 0.9238795325112867385, 1.000000000000000000, 0.9238795325112867385, 1.000000000000000000, 0.9238795325112867385, 1.000000000000000000, 0.9238795325112867385, 1.000000000000000000, 0.9238795325112867385, 1.000000000000000000, 0.9238795325112867385, 1.000000000000000000, 0.9238795325112867385, 1.000000000000000000, 0.9238795325112867385, 1.000000000000000000, 0.9238795325112867385, 1.000000000000000000, 0.9238795325112867385, 1.000000000000000000, 0.9238795325112867385, 1.000000000000000000, 0.9238795325112867385, 1.000000000000000000, 0.9238795325112867385, 1.000000000000000000, 0.9238795325112867385, 1.000000000000000000, 0.9238795325112867385, 1.000000000000000000, 0.9238795325112867385, 1.000000000000000000, 0.9238795325112867385, 1.000000000000000000, 0.9238795325112867385, 1.000000000000000000, 0.9238795325112867385, 1.000000000000000000, 0.9238795325112867385, 1.000000000000000000, 0.9238795325112867385, 1.000000000000000000, 0.9238795325112867385, 1.000000000000000000, 0.9238795325112867385, 1.000000000000000000, 0.9238795325112867385, 1.000000000000000000, 0.9238795325112867385, 1.000000000000000000, 0.9238795325112867385, 1.000000000000000000 ) ) 
 REPRESENTATION_ITEM ( '' )  );
#12710=CARTESIAN_POINT ( 'NONE',  ( 107.0000000000000142, 112.2744378736303332, -50.90000000000001279 ) ) ;
#12715=CARTESIAN_POINT ( 'NONE',  ( 105.6631189606246295, 105.8855032339526758, -43.70000000546238539 ) ) ;
#12717=ORIENTED_EDGE ( 'NONE', *, *, #15545, .F. ) ;
#12718=ORIENTED_EDGE ( 'NONE', *, *, #3440, .T. ) ;
#12723=DIRECTION ( 'NONE',  ( -0.000000000000000000, 1.000000000000000000, -0.000000000000000000 ) ) ;
#12727=DIRECTION ( 'NONE',  ( -0.000000000000000000, 1.000000000000000000, -0.000000000000000000 ) ) ;
#12747=CARTESIAN_POINT ( 'NONE',  ( 98.96446609406727646, 123.3500000021849701, -2.499999999999997780 ) ) ;
#12749=EDGE_CURVE ( 'NONE', #25694, #4172, #24620, .T. ) ;
#12752=CARTESIAN_POINT ( 'NONE',  ( 97.83688103937537051, 103.3426043859339103, -48.10000000546237686 ) ) ;
#12754=CARTESIAN_POINT ( 'NONE',  ( 97.50000000000000000, 123.5000000021849615, -9.540979117872439019E-15 ) ) ;
#12761=CARTESIAN_POINT ( 'NONE',  ( 99.99999999999998579, 101.5015231886685854, -44.87500000273119838 ) ) ;
#12763=APPLICATION_CONTEXT ( 'automotive_design' ) ;
#12765=CARTESIAN_POINT ( 'NONE',  ( 102.0669872999999939, 124.4000000010924651, -0.8561741729129507261 ) ) ;
#12780=EDGE_CURVE ( 'NONE', #20388, #21081, #21503, .T. ) ;
#12781=CARTESIAN_POINT ( 'NONE',  ( 105.6631189606246295, 114.1144967660473242, -52.80000000000000426 ) ) ;
#12785=CARTESIAN_POINT ( 'NONE',  ( 102.4999999999999858, 122.3000000021849587, -9.847140817659276890E-15 ) ) ;
#12787=CARTESIAN_POINT ( 'NONE',  ( 103.1528011352953484, 95.18749999863440792, 3.152801135295352886 ) ) ;
#12793=CARTESIAN_POINT ( 'NONE',  ( 93.46109445667491400, 105.2492070361643215, -47.17500000273119554 ) ) ;
#12797=CARTESIAN_POINT ( 'NONE',  ( 104.4587341249999923, 95.24999999863437949, 1.846868145590726318 ) ) ;
#12816=DIRECTION ( 'NONE',  ( -0.000000000000000000, -0.000000000000000000, 1.000000000000000000 ) ) ;
#12817=CARTESIAN_POINT ( 'NONE',  ( 97.83688103937537051, 103.3426043859339103, -51.60000000000000853 ) ) ;
#12824=DIRECTION ( 'NONE',  ( 5.782411586589357392E-17, -0.000000000000000000, 1.000000000000000000 ) ) ;
#12826=CARTESIAN_POINT ( 'NONE',  ( 97.50236033167492167, 117.6869444889999841, -53.52500000273118985 ) ) ;
#12831=AXIS2_PLACEMENT_3D ( 'NONE', #27307, #12019, #11736 ) ;
#12839=VERTEX_POINT ( 'NONE', #15958 ) ;
#12844=CARTESIAN_POINT ( 'NONE',  ( 107.0000000000000142, 110.0000000000000000, -51.00000000000000711 ) ) ;
#12845=CARTESIAN_POINT ( 'NONE',  ( 99.14382582708707048, 123.3000000010924708, 2.066987299999979211 ) ) ;
#12861=DIRECTION ( 'NONE',  ( 5.782411586589357392E-17, -0.000000000000000000, 1.000000000000000000 ) ) ;
#12870=CARTESIAN_POINT ( 'NONE',  ( 95.67376207875072680, 104.0454443415356991, -46.20000000546237118 ) ) ;
#12875=CARTESIAN_POINT ( 'NONE',  ( 99.99999999999998579, 95.00000000000000000, -6.938893903907228378E-15 ) ) ;
#12879=CARTESIAN_POINT ( 'NONE',  ( 97.50000000000000000, 124.2500000021849758, -1.035533905932742416 ) ) ;
#12883=CARTESIAN_POINT ( 'NONE',  ( 101.7677669209684552, 123.0000000000000000, 1.767766984964258992 ) ) ;
#12884=EDGE_LOOP ( 'NONE', ( #15453, #4330, #6761, #276, #20225, #25135, #2004, #7442, #18963, #17698, #10844, #1952, #19769, #12978, #12675 ) ) ;
#12885=DIRECTION ( 'NONE',  ( 0.000000000000000000, 1.000000000000000000, -0.000000000000000000 ) ) ;
#12892=CARTESIAN_POINT ( 'NONE',  ( 108.0825317500000011, 112.6261737610028320, -54.02500000273118275 ) ) ;
#12909=CARTESIAN_POINT ( 'NONE',  ( 112.9999999999999858, 118.0000000000000000, -13.00000000000000888 ) ) ;
#12913=CARTESIAN_POINT ( 'NONE',  ( 103.5355339059327235, 92.87500000000000000, 3.535533905932724874 ) ) ;
#12923=CARTESIAN_POINT ( 'NONE',  ( 93.46109445667491400, 114.7507929638356785, -45.57500000273119412 ) ) ;
#12924=CARTESIAN_POINT ( 'NONE',  ( 84.99999999999998579, 95.00000000000000000, -15.00000000000000533 ) ) ;
#12928=CARTESIAN_POINT ( 'NONE',  ( 103.1528011352953484, 91.43749999863440792, -3.152801135295366208 ) ) ;
#12929=CARTESIAN_POINT ( 'NONE',  ( 95.00000000000000000, 93.31249999726880162, -2.071067811865479058 ) ) ;
#12935=CARTESIAN_POINT ( 'NONE',  ( 104.4587341249999923, 95.24999999863437949, 1.846868145590726318 ) ) ;
#12942=ORIENTED_EDGE ( 'NONE', *, *, #12644, .T. ) ;
#12961=CARTESIAN_POINT ( 'NONE',  ( 99.99999999999998579, 101.5015231886685854, -52.62500000273118417 ) ) ;
#12971=CARTESIAN_POINT ( 'NONE',  ( 98.53841926354351699, 122.8500000010924680, -1.461580736456474794 ) ) ;
#12975=FACE_OUTER_BOUND ( 'NONE', #17300, .T. ) ;
#12978=ORIENTED_EDGE ( 'NONE', *, *, #26612, .F. ) ;
#12979=CARTESIAN_POINT ( 'NONE',  ( 95.67376207875072680, 104.0454443415356991, -49.70000000000000995 ) ) ;
#12986=VERTEX_POINT ( 'NONE', #13098 ) ;
#12991=CARTESIAN_POINT ( 'NONE',  ( 102.0710678118654329, 91.18749999999997158, -5.000000000000011546 ) ) ;
#13014=CARTESIAN_POINT ( 'NONE',  ( 95.00472066334981491, 116.8754121666685393, -51.42500000273118843 ) ) ;
#13018=CARTESIAN_POINT ( 'NONE',  ( 97.50000000000000000, 124.3000000021849587, -9.540979117872439019E-15 ) ) ;
#13024=CARTESIAN_POINT ( 'NONE',  ( 101.4615807364564546, 123.2500000010924879, 1.461580736456455476 ) ) ;
#13028=FACE_OUTER_BOUND ( 'NONE', #14345, .T. ) ;
#13031=CARTESIAN_POINT ( 'NONE',  ( 91.91746824999999887, 110.0000000000000000, -53.12500000273119838 ) ) ;
#13038=ORIENTED_EDGE ( 'NONE', *, *, #18718, .T. ) ;
#13040=ADVANCED_FACE ( 'NONE', ( #8286 ), #13667, .T. ) ;
#13066=CARTESIAN_POINT ( 'NONE',  ( 104.3262379212492590, 104.0454443415356991, -43.80000000546238681 ) ) ;
#13067=CARTESIAN_POINT ( 'NONE',  ( 95.54126587499999346, 93.87499999863439371, 1.846868145590722543 ) ) ;
#13068=CARTESIAN_POINT ( 'NONE',  ( 97.92893218813449607, 93.18749999726877320, -4.999999999999971578 ) ) ;
#13072=VERTEX_POINT ( 'NONE', #16943 ) ;
#13074=EDGE_CURVE ( 'NONE', #10899, #4535, #26210, .T. ) ;
#13075=CARTESIAN_POINT ( 'NONE',  ( 101.8468681455907330, 93.12499999863439371, 4.458734124999979898 ) ) ;
#13080=ORIENTED_EDGE ( 'NONE', *, *, #11709, .T. ) ;
#13096=ADVANCED_FACE ( 'NONE', ( #1995 ), #25929, .F. ) ;
#13098=CARTESIAN_POINT ( 'NONE',  ( 93.00000000000000000, 110.0000000000000000, -48.00000000000000711 ) ) ;
#13100=CARTESIAN_POINT ( 'NONE',  ( 101.7677669529663547, 123.7000000000000028, 1.767766952966350891 ) ) ;
#13114=CARTESIAN_POINT ( 'NONE',  ( 99.99999999999998579, 95.00000000000000000, 4.999999999999983125 ) ) ;
#13118=VERTEX_POINT ( 'NONE', #3995 ) ;
#13119=CARTESIAN_POINT ( 'NONE',  ( 97.83688103937538472, 116.6573956140660897, -52.40000000000000568 ) ) ;
#13127=CARTESIAN_POINT ( 'NONE',  ( 104.9999999999999858, 94.87499999726881583, -6.938893903907228378E-15 ) ) ;
#13153=ORIENTED_EDGE ( 'NONE', *, *, #26208, .T. ) ;
#13161=CARTESIAN_POINT ( 'NONE',  ( 102.4999999999999716, 123.0500000021849445, 1.035533905932722876 ) ) ;
#13166=CARTESIAN_POINT ( 'NONE',  ( 97.50000000000000000, 122.7000000021849502, -9.540979117872439019E-15 ) ) ;
#13173=CARTESIAN_POINT ( 'NONE',  ( 97.50236033167492167, 102.3130555110000159, -50.72500000273119980 ) ) ;
#13184=( BOUNDED_CURVE ( )  B_SPLINE_CURVE ( 2, ( #1726, #21389, #21663, #15077, #27804, #3999, #4272, #8684, #1866, #25933, #10531 ),
 .UNSPECIFIED., .F., .T. ) 
 B_SPLINE_CURVE_WITH_KNOTS ( ( 3, 2, 2, 2, 2, 3 ),
 ( 0.9000000000000000222, 0.9200000000000000400, 0.9399999999999999467, 0.9599999999999999645, 0.9799999999999999822, 1.000000000000000000 ),
 .UNSPECIFIED. ) 
 CURVE ( )  GEOMETRIC_REPRESENTATION_ITEM ( )  RATIONAL_B_SPLINE_CURVE ( ( 1.000000000000000000, 0.9510565162951535312, 1.000000000000000000, 0.9510565162951535312, 1.000000000000000000, 0.9510565162951535312, 1.000000000000000000, 0.9510565162951535312, 1.000000000000000000, 0.9510565162951535312, 1.000000000000000000 ) ) 
 REPRESENTATION_ITEM ( '' )  );
#13189=CARTESIAN_POINT ( 'NONE',  ( 84.99999999999998579, 95.00000000000000000, 14.99999999999999467 ) ) ;
#13193=MECHANICAL_DESIGN_GEOMETRIC_PRESENTATION_REPRESENTATION('',(#25076),#4139);
#13197=CARTESIAN_POINT ( 'NONE',  ( 104.9999999999999716, 93.06249999999998579, -2.071067811865478170 ) ) ;
#13207=CARTESIAN_POINT ( 'NONE',  ( 91.91746824999998466, 107.3738262389971680, -45.27500000273118985 ) ) ;
#13211=CARTESIAN_POINT ( 'NONE',  ( 97.57936185695767506, 123.0000000000000000, -0.6890590944183185851 ) ) ;
#13215=VERTEX_POINT ( 'NONE', #13785 ) ;
#13220=CARTESIAN_POINT ( 'NONE',  ( 103.5355339059327235, 90.12500000000000000, -3.535533905932738197 ) ) ;
#13233=PRODUCT_DEFINITION ( 'UNKNOWN', '', #21314, #27459 ) ;
#13236=EDGE_CURVE ( 'NONE', #12623, #10198, #17411, .T. ) ;
#13243=CARTESIAN_POINT ( 'NONE',  ( 95.00472066334982912, 103.1245878333314323, -50.82500000273118701 ) ) ;
#13250=CARTESIAN_POINT ( 'NONE',  ( 107.0000000000000142, 112.2744378736303332, -51.40000000546236691 ) ) ;
#13251=CARTESIAN_POINT ( 'NONE',  ( 100.8561741729129437, 123.2000000010924765, 2.066987299999979655 ) ) ;
#13254=EDGE_LOOP ( 'NONE', ( #8280, #21196, #20759, #22123, #3767, #5231, #24970, #2623, #3495, #26424, #5163, #8265, #19106 ) ) ;
#13258=ORIENTED_EDGE ( 'NONE', *, *, #13961, .T. ) ;
#13259=CARTESIAN_POINT ( 'NONE',  ( 93.00000000000001421, 112.2744378736303332, -48.10000000000000142 ) ) ;
#13261=CARTESIAN_POINT ( 'NONE',  ( 97.50000000000000000, 124.9500000000000028, -1.035533905932742416 ) ) ;
#13264=CARTESIAN_POINT ( 'NONE',  ( 97.92893218813452449, 92.18749999726880162, -4.999999999999997335 ) ) ;
#13285=ORIENTED_EDGE ( 'NONE', *, *, #6335, .T. ) ;
#13286=ORIENTED_EDGE ( 'NONE', *, *, #14042, .T. ) ;
#13289=ORIENTED_EDGE ( 'NONE', *, *, #1510, .T. ) ;
#13303=EDGE_CURVE ( 'NONE', #20591, #14157, #16592, .T. ) ;
#13304=CARTESIAN_POINT ( 'NONE',  ( 101.0355339059327378, 124.0500000021849445, -2.499999999999997780 ) ) ;
#13306=ORIENTED_EDGE ( 'NONE', *, *, #10677, .F. ) ;
#13309=VERTEX_POINT ( 'NONE', #14354 ) ;
#13310=CARTESIAN_POINT ( 'NONE',  ( 102.0669872999999797, 124.1500000010924794, -9.794112055954760458E-15 ) ) ;
#13313=ADVANCED_FACE ( 'NONE', ( #3547 ), #20931, .F. ) ;
#13316=PLANE ( 'NONE',  #3585 ) ;
#13320=CARTESIAN_POINT ( 'NONE',  ( 91.91746824999998466, 107.3738262389971538, -53.02500000273119696 ) ) ;
#13338=CARTESIAN_POINT ( 'NONE',  ( 101.0355339059327235, 123.7500000021849615, 2.499999999999987121 ) ) ;
#13342=DIRECTION ( 'NONE',  ( 1.000000000000000000, 0.000000000000000000, -5.782411586589357392E-17 ) ) ;
#13352=LINE ( 'NONE', #9100, #5864 ) ;
#13353=CARTESIAN_POINT ( 'NONE',  ( 91.00000000000000000, 110.0000000000000000, -45.00000000000000711 ) ) ;
#13365=CARTESIAN_POINT ( 'NONE',  ( 95.54126587499999346, 93.87499999863439371, 1.846868145590722543 ) ) ;
#13387=AXIS2_PLACEMENT_3D ( 'NONE', #22775, #11910, #27334 ) ;
#13389=CARTESIAN_POINT ( 'NONE',  ( 106.5389055433251002, 114.7507929638356785, -45.92500000273119554 ) ) ;
#13396=CARTESIAN_POINT ( 'NONE',  ( 97.83688103937538472, 116.6573956140660897, -50.90000000546238113 ) ) ;
#13405=CARTESIAN_POINT ( 'NONE',  ( 102.4976396683250925, 117.6869444889999841, -51.97500000273119980 ) ) ;
#13408=CARTESIAN_POINT ( 'NONE',  ( 97.50000000000000000, 125.0000000000000000, -9.540979117872439019E-15 ) ) ;
#13411=CARTESIAN_POINT ( 'NONE',  ( 95.00000000000000000, 93.43749999726880162, 2.071067811865463959 ) ) ;
#13422=CARTESIAN_POINT ( 'NONE',  ( 102.0710678118654471, 91.06249999726878741, -5.000000000000000000 ) ) ;
#13427=CARTESIAN_POINT ( 'NONE',  ( 104.4587341249999923, 90.62499999863439371, -1.846868145590737198 ) ) ;
#13438=ORIENTED_EDGE ( 'NONE', *, *, #6510, .F. ) ;
#13444=CARTESIAN_POINT ( 'NONE',  ( 97.50236033167492167, 117.6869444889999841, -53.52500000273118985 ) ) ;
#13446=DIRECTION ( 'NONE',  ( 0.000000000000000000, 0.000000000000000000, -1.000000000000000000 ) ) ;
#13452=CARTESIAN_POINT ( 'NONE',  ( 97.93301269999999192, 122.9000000010924936, -0.8561741729129505041 ) ) ;
#13459=EDGE_CURVE ( 'NONE', #7002, #17147, #24923, .T. ) ;
#13487=ADVANCED_FACE ( 'NONE', ( #23897 ), #26031, .T. ) ;
#13489=CARTESIAN_POINT ( 'NONE',  ( 96.46446609406726225, 94.24999999726881583, -3.535533905932738197 ) ) ;
#13501=LINE ( 'NONE', #561, #7397 ) ;
#13504=CARTESIAN_POINT ( 'NONE',  ( 101.8427817263613235, 123.0000000000000284, -1.695516854503018589 ) ) ;
#13514=CARTESIAN_POINT ( 'NONE',  ( 97.92893218813452449, 92.31250000000000000, -4.999999999999997335 ) ) ;
#13519=VERTEX_POINT ( 'NONE', #14762 ) ;
#13529=DIRECTION ( 'NONE',  ( -5.782411586589357392E-17, -0.000000000000000000, -1.000000000000000000 ) ) ;
#13539=CARTESIAN_POINT ( 'NONE',  ( 99.99999999999998579, 117.3602355696678501, -53.00000000546238255 ) ) ;
#13554=CARTESIAN_POINT ( 'NONE',  ( 93.00000000000000000, 110.0000000000000000, -46.00000000000000711 ) ) ;
#13556=CARTESIAN_POINT ( 'NONE',  ( 99.99999999999998579, 124.0000000000000000, -2.499999999999997780 ) ) ;
#13561=CARTESIAN_POINT ( 'NONE',  ( 102.0710678118654613, 95.06249999726880162, -4.999999999999997335 ) ) ;
#13564=CARTESIAN_POINT ( 'NONE',  ( 104.9952793366501709, 116.8754121666685393, -52.07500000273120122 ) ) ;
#13570=DIRECTION ( 'NONE',  ( -5.782411586589357392E-17, 0.000000000000000000, -1.000000000000000000 ) ) ;
#13582=VERTEX_POINT ( 'NONE', #2246 ) ;
#13592=CARTESIAN_POINT ( 'NONE',  ( 99.99999999999998579, 101.5015231886685712, -50.62500000273119838 ) ) ;
#13597=ORIENTED_EDGE ( 'NONE', *, *, #20062, .F. ) ;
#13600=CARTESIAN_POINT ( 'NONE',  ( 101.4615807364564546, 123.4500000010924765, -1.461580736456474794 ) ) ;
#13603=AXIS2_PLACEMENT_3D ( 'NONE', #15112, #2603, #17410 ) ;
#13607=CARTESIAN_POINT ( 'NONE',  ( 104.4587341249999781, 92.31249999863440792, -6.938893903907228378E-15 ) ) ;
#13612=CARTESIAN_POINT ( 'NONE',  ( 99.99999999999998579, 91.62499999726880162, 4.999999999999984013 ) ) ;
#13631=CARTESIAN_POINT ( 'NONE',  ( 101.7677669529663547, 124.5069999999781487, 1.767766952966350891 ) ) ;
#13633=SURFACE_STYLE_USAGE ( .BOTH. , #9793 ) ;
#13637=LINE ( 'NONE', #24771, #17858 ) ;
#13639=CARTESIAN_POINT ( 'NONE',  ( 95.67376207875072680, 115.9545556584642867, -54.30000000000001137 ) ) ;
#13650=CARTESIAN_POINT ( 'NONE',  ( 98.17215415578155557, 123.0000000000000000, 1.711519470631157391 ) ) ;
#13658=CARTESIAN_POINT ( 'NONE',  ( 99.99999999999998579, 93.75000000000000000, 4.999999999999984013 ) ) ;
#13663=EDGE_LOOP ( 'NONE', ( #1834, #20884 ) ) ;
#13667=( BOUNDED_SURFACE ( )  B_SPLINE_SURFACE ( 1, 2, ( 
 ( #21839, #2452, #21695, #15393, #23825, #4166, #12826, #28106, #15247, #6158, #23548, #10972, #14825, #4305, #23967, #12961, #8570, #25818, #2027, #6293, #24106, #21553, #4025, #12691, #19402, #21416, #19684, #17261, #171, #25962, #14970, #17402, #2169, #13243, #10831, #10695, #4583, #19547, #8853, #1894, #10560, #26247, #21975, #28, #19269, #8710, #27968, #8425, #6567, #17542, #4446, #9137, #26681, #20119, #22399, #17830, #3158, #8998, #5298, #7415, #16110, #22260, #4729, #15965, #19976, #15826, #13819, #26971, #22543, #7129, #9415, #22116, #13682, #15685, #3011, #11682, #11257, #9277, #20405, #2596, #17973, #24531, #13389, #890, #9561, #455, #24679, #18264, #26534, #24815, #5156, #597, #13963, #22688, #11828, #24386, #312, #17690, #4875, #26395, #6991 ),
 ( #5017, #2868, #6849, #15538, #24246, #13539, #2735, #11400, #11539, #20256, #741, #18114, #26828, #7274, #18951, #16402, #1588, #5993, #25100, #25378, #5441, #27112, #12101, #18405, #14528, #7562, #7848, #8122, #23243, #18818, #10243, #5858, #3435, #27660, #16256, #14250, #3851, #1033, #11969, #1305, #24956, #20828, #23379, #14109, #1175, #16817, #20552, #22833, #3720, #14658, #5724, #25514, #18686, #5585, #7708, #9974, #27525, #3299, #20692, #12382, #9704, #27389, #7981, #25233, #16543, #9840, #22971, #18547, #27251, #14389, #23106, #3580, #12237, #20966, #21100, #1449, #10105, #16679, #19233, #21659, #19370, #17508, #8538, #17082, #133, #1862, #4411, #15358, #14793, #2281, #10939, #28073, #19651, #21383, #19091, #24073, #17224, #13066, #8819, #10527, #10662 ) ),
 .UNSPECIFIED., .F., .F., .F. ) 
 B_SPLINE_SURFACE_WITH_KNOTS ( ( 2, 2 ),
 ( 3, 2, 2, 2, 2, 2, 2, 2, 2, 2, 2, 2, 2, 2, 2, 2, 2, 2, 2, 2, 2, 2, 2, 2, 2, 2, 2, 2, 2, 2, 2, 2, 2, 2, 2, 2, 2, 2, 2, 2, 2, 2, 2, 2, 2, 2, 2, 2, 2, 2, 3 ),
 ( 0.000000000000000000, 1.000000000000000000 ),
 ( 0.000000000000000000, 0.02000000000000000042, 0.04000000000000000083, 0.05999999999999999778, 0.08000000000000000167, 0.1000000000000000056, 0.1199999999999999956, 0.1400000000000000133, 0.1600000000000000033, 0.1799999999999999933, 0.2000000000000000111, 0.2200000000000000011, 0.2399999999999999911, 0.2600000000000000089, 0.2800000000000000266, 0.2999999999999999889, 0.3200000000000000067, 0.3400000000000000244, 0.3599999999999999867, 0.3800000000000000044, 0.4000000000000000222, 0.4199999999999999845, 0.4400000000000000022, 0.4600000000000000200, 0.4799999999999999822, 0.5000000000000000000, 0.5200000000000000178, 0.5400000000000000355, 0.5600000000000000533, 0.5799999999999999600, 0.5999999999999999778, 0.6199999999999999956, 0.6400000000000000133, 0.6600000000000000311, 0.6800000000000000488, 0.6999999999999999556, 0.7199999999999999734, 0.7399999999999999911, 0.7600000000000000089, 0.7800000000000000266, 0.8000000000000000444, 0.8199999999999999512, 0.8399999999999999689, 0.8599999999999999867, 0.8800000000000000044, 0.9000000000000000222, 0.9200000000000000400, 0.9399999999999999467, 0.9599999999999999645, 0.9799999999999999822, 1.000000000000000000 ),
 .UNSPECIFIED. ) 
 GEOMETRIC_REPRESENTATION_ITEM ( )  RATIONAL_B_SPLINE_SURFACE ( (
 ( 1.000000000000000000, 0.9510565162951535312, 1.000000000000000000, 0.9510565162951535312, 1.000000000000000000, 0.9510565162951535312, 1.000000000000000000, 0.9510565162951535312, 1.000000000000000000, 0.9510565162951535312, 1.000000000000000000, 0.9510565162951535312, 1.000000000000000000, 0.9510565162951535312, 1.000000000000000000, 0.9510565162951535312, 1.000000000000000000, 0.9510565162951535312, 1.000000000000000000, 0.9510565162951535312, 1.000000000000000000, 0.9510565162951535312, 1.000000000000000000, 0.9510565162951535312, 1.000000000000000000, 0.9510565162951535312, 1.000000000000000000, 0.9510565162951535312, 1.000000000000000000, 0.9510565162951535312, 1.000000000000000000, 0.9510565162951535312, 1.000000000000000000, 0.9510565162951535312, 1.000000000000000000, 0.9510565162951535312, 1.000000000000000000, 0.9510565162951535312, 1.000000000000000000, 0.9510565162951535312, 1.000000000000000000, 0.9510565162951535312, 1.000000000000000000, 0.9510565162951535312, 1.000000000000000000, 0.9510565162951535312, 1.000000000000000000, 0.9510565162951535312, 1.000000000000000000, 0.9510565162951535312, 1.000000000000000000, 0.9510565162951535312, 1.000000000000000000, 0.9510565162951535312, 1.000000000000000000, 0.9510565162951535312, 1.000000000000000000, 0.9510565162951535312, 1.000000000000000000, 0.9510565162951535312, 1.000000000000000000, 0.9510565162951535312, 1.000000000000000000, 0.9510565162951535312, 1.000000000000000000, 0.9510565162951535312, 1.000000000000000000, 0.9510565162951535312, 1.000000000000000000, 0.9510565162951535312, 1.000000000000000000, 0.9510565162951535312, 1.000000000000000000, 0.9510565162951535312, 1.000000000000000000, 0.9510565162951535312, 1.000000000000000000, 0.9510565162951535312, 1.000000000000000000, 0.9510565162951535312, 1.000000000000000000, 0.9510565162951535312, 1.000000000000000000, 0.9510565162951535312, 1.000000000000000000, 0.9510565162951535312, 1.000000000000000000, 0.9510565162951535312, 1.000000000000000000, 0.9510565162951535312, 1.000000000000000000, 0.9510565162951535312, 1.000000000000000000, 0.9510565162951535312, 1.000000000000000000, 0.9510565162951535312, 1.000000000000000000, 0.9510565162951535312, 1.000000000000000000, 0.9510565162951535312, 1.000000000000000000),
 ( 1.000000000000000000, 0.9510565162951535312, 1.000000000000000000, 0.9510565162951535312, 1.000000000000000000, 0.9510565162951535312, 1.000000000000000000, 0.9510565162951535312, 1.000000000000000000, 0.9510565162951535312, 1.000000000000000000, 0.9510565162951535312, 1.000000000000000000, 0.9510565162951535312, 1.000000000000000000, 0.9510565162951535312, 1.000000000000000000, 0.9510565162951535312, 1.000000000000000000, 0.9510565162951535312, 1.000000000000000000, 0.9510565162951535312, 1.000000000000000000, 0.9510565162951535312, 1.000000000000000000, 0.9510565162951535312, 1.000000000000000000, 0.9510565162951535312, 1.000000000000000000, 0.9510565162951535312, 1.000000000000000000, 0.9510565162951535312, 1.000000000000000000, 0.9510565162951535312, 1.000000000000000000, 0.9510565162951535312, 1.000000000000000000, 0.9510565162951535312, 1.000000000000000000, 0.9510565162951535312, 1.000000000000000000, 0.9510565162951535312, 1.000000000000000000, 0.9510565162951535312, 1.000000000000000000, 0.9510565162951535312, 1.000000000000000000, 0.9510565162951535312, 1.000000000000000000, 0.9510565162951535312, 1.000000000000000000, 0.9510565162951535312, 1.000000000000000000, 0.9510565162951535312, 1.000000000000000000, 0.9510565162951535312, 1.000000000000000000, 0.9510565162951535312, 1.000000000000000000, 0.9510565162951535312, 1.000000000000000000, 0.9510565162951535312, 1.000000000000000000, 0.9510565162951535312, 1.000000000000000000, 0.9510565162951535312, 1.000000000000000000, 0.9510565162951535312, 1.000000000000000000, 0.9510565162951535312, 1.000000000000000000, 0.9510565162951535312, 1.000000000000000000, 0.9510565162951535312, 1.000000000000000000, 0.9510565162951535312, 1.000000000000000000, 0.9510565162951535312, 1.000000000000000000, 0.9510565162951535312, 1.000000000000000000, 0.9510565162951535312, 1.000000000000000000, 0.9510565162951535312, 1.000000000000000000, 0.9510565162951535312, 1.000000000000000000, 0.9510565162951535312, 1.000000000000000000, 0.9510565162951535312, 1.000000000000000000, 0.9510565162951535312, 1.000000000000000000, 0.9510565162951535312, 1.000000000000000000, 0.9510565162951535312, 1.000000000000000000, 0.9510565162951535312, 1.000000000000000000, 0.9510565162951535312, 1.000000000000000000) ) ) 
 REPRESENTATION_ITEM ( '' )  SURFACE ( )  );
#13678=CARTESIAN_POINT ( 'NONE',  ( 99.99999999999998579, 90.00000000000000000, 4.999999999999983125 ) ) ;
#13682=CARTESIAN_POINT ( 'NONE',  ( 93.46109445667491400, 105.2492070361643215, -46.92500000273119554 ) ) ;
#13683=CARTESIAN_POINT ( 'NONE',  ( 104.4587341249999923, 92.49999999863442213, 1.846868145590726318 ) ) ;
#13697=ORIENTED_EDGE ( 'NONE', *, *, #71, .F. ) ;
#13698=CARTESIAN_POINT ( 'NONE',  ( 106.5389055433251002, 105.2492070361643215, -52.57500000273119412 ) ) ;
#13704=CARTESIAN_POINT ( 'NONE',  ( 103.1528011352953484, 91.43749999863440792, 3.152801135295352886 ) ) ;
#13706=CARTESIAN_POINT ( 'NONE',  ( 104.9952793366501709, 116.8754121666685393, -54.07500000273119412 ) ) ;
#13708=CARTESIAN_POINT ( 'NONE',  ( 101.7677669529663547, 123.2000000021849502, -1.767766952966370209 ) ) ;
#13714=LINE ( 'NONE', #22148, #10601 ) ;
#13731=CYLINDRICAL_SURFACE ( 'NONE', #5880, 5.000000000000004441 ) ;
#13733=CARTESIAN_POINT ( 'NONE',  ( 97.50236033167492167, 102.3130555110000159, -48.72500000273119269 ) ) ;
#13737=EDGE_LOOP ( 'NONE', ( #19239, #20163, #22579, #19379, #14608, #11415, #1766, #13306, #18232, #25071, #13697, #13438, #15296 ) ) ;
#13747=CARTESIAN_POINT ( 'NONE',  ( 104.9952793366501851, 116.8754121666685393, -45.82500000273119412 ) ) ;
#13771=( NAMED_UNIT ( * ) PLANE_ANGLE_UNIT ( ) SI_UNIT ( $, .RADIAN. ) );
#13784=CARTESIAN_POINT ( 'NONE',  ( 99.99999999999998579, 118.4984768113314004, -51.87500000273118417 ) ) ;
#13785=CARTESIAN_POINT ( 'NONE',  ( 114.9999999999999858, 95.00000000000000000, 14.99999999999999289 ) ) ;
#13788=CARTESIAN_POINT ( 'NONE',  ( 99.99999999999998579, 124.3500000010924822, -2.066987299999998751 ) ) ;
#13793=CARTESIAN_POINT ( 'NONE',  ( 97.92893218813448186, 94.31250000000001421, -4.999999999999948486 ) ) ;
#13795=CARTESIAN_POINT ( 'NONE',  ( 95.00000000000000000, 90.50000000000000000, -7.551217303480904118E-15 ) ) ;
#13804=EDGE_LOOP ( 'NONE', ( #26142, #3363, #1524, #18698 ) ) ;
#13812=DIRECTION ( 'NONE',  ( 5.782411586589357392E-17, 0.000000000000000000, 1.000000000000000000 ) ) ;
#13813=CARTESIAN_POINT ( 'NONE',  ( 99.99999999999998579, 92.56249999863440792, -4.458734124999994997 ) ) ;
#13817=CARTESIAN_POINT ( 'NONE',  ( 98.23223304703363112, 123.2999999999999972, -1.767766952966370209 ) ) ;
#13819=CARTESIAN_POINT ( 'NONE',  ( 97.50236033167492167, 117.6869444889999841, -47.52500000273119696 ) ) ;
#13826=EDGE_CURVE ( 'NONE', #6897, #7134, #26897, .T. ) ;
#13831=EDGE_CURVE ( 'NONE', #18466, #12623, #16754, .T. ) ;
#13834=ORIENTED_EDGE ( 'NONE', *, *, #11586, .T. ) ;
#13835=CARTESIAN_POINT ( 'NONE',  ( 102.4976396683250925, 117.6869444889999841, -53.97500000273119980 ) ) ;
#13837=CARTESIAN_POINT ( 'NONE',  ( 98.96446609406727646, 124.0499999999999972, -2.499999999999997780 ) ) ;
#13844=CARTESIAN_POINT ( 'NONE',  ( 98.15313185440925281, 94.24999999863439371, 4.458734124999979898 ) ) ;
#13846=CARTESIAN_POINT ( 'NONE',  ( 106.5389055433251002, 105.2492070361643215, -48.57500000273119412 ) ) ;
#13847=ADVANCED_FACE ( 'NONE', ( #19015, #27866 ), #21588, .T. ) ;
#13852=CARTESIAN_POINT ( 'NONE',  ( 102.4999999999999858, 124.6000000000000085, -9.847140817659276890E-15 ) ) ;
#13858=CARTESIAN_POINT ( 'NONE',  ( 101.8468681455907330, 92.37499999863440792, 4.458734124999980786 ) ) ;
#13865=ORIENTED_EDGE ( 'NONE', *, *, #11572, .F. ) ;
#13875=CARTESIAN_POINT ( 'NONE',  ( 95.00472066334981491, 103.1245878333314465, -50.82500000273119412 ) ) ;
#13909=CARTESIAN_POINT ( 'NONE',  ( 84.99999999999998579, 120.0000000000000000, -45.00000000000000711 ) ) ;
#13913=CARTESIAN_POINT ( 'NONE',  ( 99.99999999999998579, 124.0069999999781487, -2.499999999999997780 ) ) ;
#13926=EDGE_CURVE ( 'NONE', #2259, #24967, #8189, .T. ) ;
#13927=FACE_OUTER_BOUND ( 'NONE', #18643, .T. ) ;
#13930=CARTESIAN_POINT ( 'NONE',  ( 98.53841926354351699, 123.8500000010924680, 1.461580736456455920 ) ) ;
#13938=CARTESIAN_POINT ( 'NONE',  ( 103.5355339059327235, 94.12500000000000000, -3.535533905932738197 ) ) ;
#13955=CARTESIAN_POINT ( 'NONE',  ( 104.4587341249999781, 91.31249999863440792, -6.938893903907228378E-15 ) ) ;
#13961=EDGE_CURVE ( 'NONE', #26002, #26108, #17296, .T. ) ;
#13963=CARTESIAN_POINT ( 'NONE',  ( 93.46109445667491400, 105.2492070361643215, -44.92500000273119554 ) ) ;
#13964=CARTESIAN_POINT ( 'NONE',  ( 96.84719886470463734, 91.18749999863440792, 3.152801135295351997 ) ) ;
#13970=CARTESIAN_POINT ( 'NONE',  ( 97.50000000000000000, 123.5000000021849615, -9.540979117872439019E-15 ) ) ;
#13976=CARTESIAN_POINT ( 'NONE',  ( 104.9952793366501851, 116.8754121666685393, -52.07500000273120122 ) ) ;
#13983=ADVANCED_FACE ( 'NONE', ( #16880 ), #1929, .F. ) ;
#13984=CARTESIAN_POINT ( 'NONE',  ( 99.99999999999998579, 90.81249999863440792, -4.458734124999994997 ) ) ;
#13985=CIRCLE ( 'NONE', #10339, 4.999999999999989342 ) ;
#13988=CARTESIAN_POINT ( 'NONE',  ( 97.50236033167492167, 102.3130555110000159, -52.97500000273119980 ) ) ;
#13997=CARTESIAN_POINT ( 'NONE',  ( 100.0000000000000000, 110.0000000000000000, -55.00000000000000711 ) ) ;
#14003=CARTESIAN_POINT ( 'NONE',  ( 104.4587341249999781, 92.56249999863440792, -6.938893903907228378E-15 ) ) ;
#14009=CARTESIAN_POINT ( 'NONE',  ( 87.00000000000000000, 0.000000000000000000, 8.673617379884035472E-16 ) ) ;
#14011=CARTESIAN_POINT ( 'NONE',  ( 99.14382582708708469, 123.0000000010924879, -2.066987299999998751 ) ) ;
#14021=CARTESIAN_POINT ( 'NONE',  ( 105.0000000000000000, 110.0000000000000000, -43.00000000000000000 ) ) ;
#14030=AXIS2_PLACEMENT_3D ( 'NONE', #17813, #24229, #434 ) ;
#14034=CARTESIAN_POINT ( 'NONE',  ( 97.50236033167492167, 102.3130555110000159, -46.72500000273119269 ) ) ;
#14036=ADVANCED_FACE ( 'NONE', ( #12441 ), #25443, .F. ) ;
#14042=EDGE_CURVE ( 'NONE', #7134, #26108, #2064, .T. ) ;
#14064=CARTESIAN_POINT ( 'NONE',  ( 92.99999999999997158, 107.7255621263696810, -47.89999999999999147 ) ) ;
#14065=DIRECTION ( 'NONE',  ( -0.000000000000000000, 4.625929269271485914E-16, 1.000000000000000000 ) ) ;
#14071=EDGE_CURVE ( 'NONE', #24017, #11839, #28004, .T. ) ;
#14076=CARTESIAN_POINT ( 'NONE',  ( 108.0825317500000153, 110.0000000000000000, -54.37500000273119838 ) ) ;
#14077=CARTESIAN_POINT ( 'NONE',  ( 84.99999999999998579, 125.0000000000000000, 14.99999999999999112 ) ) ;
#14078=CARTESIAN_POINT ( 'NONE',  ( 99.99999999999998579, 123.5500000010924850, -2.066987299999998751 ) ) ;
#14087=CARTESIAN_POINT ( 'NONE',  ( 95.00000000000000000, 91.50000000000000000, -7.551217303480904118E-15 ) ) ;
#14093=ORIENTED_EDGE ( 'NONE', *, *, #8997, .T. ) ;
#14101=CARTESIAN_POINT ( 'NONE',  ( 104.3262379212492590, 104.0454443415356991, -49.80000000546237970 ) ) ;
#14102=CARTESIAN_POINT ( 'NONE',  ( 95.54126587499999346, 90.74999999863439371, -1.846868145590737864 ) ) ;
#14107=CARTESIAN_POINT ( 'NONE',  ( 104.3262379212492590, 115.9545556584642867, -53.20000000546237118 ) ) ;
#14109=CARTESIAN_POINT ( 'NONE',  ( 104.3262379212492590, 115.9545556584642867, -49.20000000546238539 ) ) ;
#14110=CARTESIAN_POINT ( 'NONE',  ( 104.4587341249999781, 91.56249999863440792, -6.938893903907228378E-15 ) ) ;
#14123=EDGE_CURVE ( 'NONE', #12623, #4367, #16046, .T. ) ;
#14125=CARTESIAN_POINT ( 'NONE',  ( 99.99999999999998579, 101.5015231886685854, -44.87500000273119838 ) ) ;
#14132=CARTESIAN_POINT ( 'NONE',  ( 101.8468681455907330, 93.37499999863439371, 4.458734124999979898 ) ) ;
#14133=CYLINDRICAL_SURFACE ( 'NONE', #6402, 4.999999999999989342 ) ;
#14139=PLANE ( 'NONE',  #16307 ) ;
#14143=ORIENTED_EDGE ( 'NONE', *, *, #20668, .T. ) ;
#14146=CARTESIAN_POINT ( 'NONE',  ( 104.4587341249999923, 93.62499999863439371, -1.846868145590737198 ) ) ;
#14157=VERTEX_POINT ( 'NONE', #18877 ) ;
#14158=CARTESIAN_POINT ( 'NONE',  ( 107.0000000000000142, 112.2744378736303332, -54.90000000000000568 ) ) ;
#14161=ADVANCED_FACE ( 'NONE', ( #5925 ), #2487, .T. ) ;
#14164=FACE_OUTER_BOUND ( 'NONE', #2639, .T. ) ;
#14168=( BOUNDED_CURVE ( )  B_SPLINE_CURVE ( 2, ( #6167, #3755, #14834, #23557, #10705, #21424, #1622, #19410, #14567, #25267, #5757, #23283, #14425, #1903, #3617, #1484, #10281, #18990, #27699, #19278, #8162, #25553, #2178, #17838, #37, #464, #24115, #13251, #11265, #17700, #9146, #25970, #24256, #22125, #12971, #15693, #2604, #23833, #9008, #19986, #322 ),
 .UNSPECIFIED., .F., .T. ) 
 B_SPLINE_CURVE_WITH_KNOTS ( ( 3, 2, 2, 2, 2, 2, 2, 2, 2, 2, 2, 2, 2, 2, 2, 2, 2, 2, 2, 2, 3 ),
 ( 0.000000000000000000, 0.04166666666666666435, 0.08333333333333332871, 0.1250000000000000000, 0.1666666666666666574, 0.2083333333333333426, 0.2500000000000000000, 0.2916666666666666852, 0.3333333333333333148, 0.3750000000000000000, 0.4166666666666666852, 0.4583333333333332593, 0.5000000000000000000, 0.5416666666666666297, 0.5833333333333333703, 0.6250000000000000000, 0.6666666666666666297, 0.7083333333333333703, 0.7500000000000000000, 0.7916666666666666297, 0.8333333333333333703 ),
 .UNSPECIFIED. ) 
 CURVE ( )  GEOMETRIC_REPRESENTATION_ITEM ( )  RATIONAL_B_SPLINE_CURVE ( ( 1.000000000000000000, 0.9238795325112867385, 1.000000000000000000, 0.9238795325112867385, 1.000000000000000000, 0.9238795325112867385, 1.000000000000000000, 0.9238795325112867385, 1.000000000000000000, 0.9238795325112867385, 1.000000000000000000, 0.9238795325112867385, 1.000000000000000000, 0.9238795325112867385, 1.000000000000000000, 0.9238795325112867385, 1.000000000000000000, 0.9238795325112867385, 1.000000000000000000, 0.9238795325112867385, 1.000000000000000000, 0.9238795325112867385, 1.000000000000000000, 0.9238795325112867385, 1.000000000000000000, 0.9238795325112867385, 1.000000000000000000, 0.9238795325112867385, 1.000000000000000000, 0.9238795325112867385, 1.000000000000000000, 0.9238795325112867385, 1.000000000000000000, 0.9238795325112867385, 1.000000000000000000, 0.9238795325112867385, 1.000000000000000000, 0.9238795325112867385, 1.000000000000000000, 0.9238795325112867385, 1.000000000000000000 ) ) 
 REPRESENTATION_ITEM ( '' )  );
#14169=SURFACE_STYLE_FILL_AREA ( #27311 ) ;
#14179=CARTESIAN_POINT ( 'NONE',  ( 94.33688103937537051, 114.1144967660473242, -48.70000000546237828 ) ) ;
#14202=CARTESIAN_POINT ( 'NONE',  ( 107.0000000000000142, 107.7255621263696526, -47.10000000000000142 ) ) ;
#14205=ORIENTED_EDGE ( 'NONE', *, *, #18185, .F. ) ;
#14211=VECTOR ( 'NONE', #17899, 999.9999999999998863 ) ;
#14212=EDGE_CURVE ( 'NONE', #9199, #1383, #966, .T. ) ;
#14217=CARTESIAN_POINT ( 'NONE',  ( 99.99999999999998579, 90.25000000000000000, -4.999999999999997335 ) ) ;
#14243=CARTESIAN_POINT ( 'NONE',  ( 104.4587341249999923, 91.37499999863442213, -1.846868145590737198 ) ) ;
#14250=CARTESIAN_POINT ( 'NONE',  ( 99.99999999999998579, 102.6397644303321215, -50.00000000546236834 ) ) ;
#14251=CARTESIAN_POINT ( 'NONE',  ( 98.15313185440925281, 94.87499999863440792, -4.458734124999994997 ) ) ;
#14259=CARTESIAN_POINT ( 'NONE',  ( 99.99999999999998579, 90.00000000000000000, -2.999999999999996447 ) ) ;
#14265=CARTESIAN_POINT ( 'NONE',  ( 108.0825317500000011, 112.6261737610028320, -48.27500000273119696 ) ) ;
#14272=CARTESIAN_POINT ( 'NONE',  ( 104.4587341249999923, 91.62499999863440792, -1.846868145590737198 ) ) ;
#14286=CARTESIAN_POINT ( 'NONE',  ( 101.8468681455907330, 94.74999999863439371, -4.458734124999994997 ) ) ;
#14296=ORIENTED_EDGE ( 'NONE', *, *, #18321, .T. ) ;
#14298=CARTESIAN_POINT ( 'NONE',  ( 97.92893218813452449, 91.56249999726881583, 4.999999999999991118 ) ) ;
#14301=CARTESIAN_POINT ( 'NONE',  ( 97.83688103937538472, 116.6573956140660897, -44.90000000546237402 ) ) ;
#14336=CARTESIAN_POINT ( 'NONE',  ( 98.96446609406727646, 124.0499999999999972, -2.499999999999997780 ) ) ;
#14344=CIRCLE ( 'NONE', #18477, 4.999999999999989342 ) ;
#14345=EDGE_LOOP ( 'NONE', ( #1352, #11883, #19375, #8900 ) ) ;
#14353=CARTESIAN_POINT ( 'NONE',  ( 91.91746824999998466, 107.3738262389971538, -45.27500000273118985 ) ) ;
#14354=CARTESIAN_POINT ( 'NONE',  ( 108.0825317500000153, 110.0000000000000000, -44.12500000273119127 ) ) ;
#14356=CARTESIAN_POINT ( 'NONE',  ( 99.14382582708707048, 123.3000000010924708, 2.066987299999979211 ) ) ;
#14363=CARTESIAN_POINT ( 'NONE',  ( 95.00000000000000000, 94.50000000000000000, -7.551217303480904118E-15 ) ) ;
#14381=CARTESIAN_POINT ( 'NONE',  ( 103.1528011352953484, 94.18749999863440792, 3.152801135295352886 ) ) ;
#14389=CARTESIAN_POINT ( 'NONE',  ( 93.00000000000001421, 112.2744378736303332, -46.60000000546238397 ) ) ;
#14390=CARTESIAN_POINT ( 'NONE',  ( 103.1528011352953484, 94.68749999863440792, -3.152801135295366208 ) ) ;
#14395=EDGE_LOOP ( 'NONE', ( #27438, #13597 ) ) ;
#14404=EDGE_LOOP ( 'NONE', ( #25290, #25358, #7254, #10590 ) ) ;
#14405=CARTESIAN_POINT ( 'NONE',  ( 91.91746824999998466, 107.3738262389971538, -45.27500000273118985 ) ) ;
#14407=AXIS2_PLACEMENT_3D ( 'NONE', #10081, #1837, #7955 ) ;
#14410=CARTESIAN_POINT ( 'NONE',  ( 104.9952793366501709, 116.8754121666685393, -45.82500000273119412 ) ) ;
#14425=CARTESIAN_POINT ( 'NONE',  ( 99.99999999999998579, 123.9500000010924765, 2.066987299999980099 ) ) ;
#14426=CARTESIAN_POINT ( 'NONE',  ( 101.8468681455907330, 95.37499999863440792, 4.458734124999980786 ) ) ;
#14432=ORIENTED_EDGE ( 'NONE', *, *, #13459, .F. ) ;
#14436=ORIENTED_EDGE ( 'NONE', *, *, #14042, .F. ) ;
#14443=CARTESIAN_POINT ( 'NONE',  ( 99.99999999999998579, 102.6397644303321215, -44.00000000546237544 ) ) ;
#14463=EDGE_LOOP ( 'NONE', ( #12611, #578, #8368, #5919 ) ) ;
#14472=DIRECTION ( 'NONE',  ( 0.000000000000000000, 0.000000000000000000, 1.000000000000000000 ) ) ;
#14473=DIRECTION ( 'NONE',  ( -5.782411586589357392E-17, -0.000000000000000000, -1.000000000000000000 ) ) ;
#14478=CARTESIAN_POINT ( 'NONE',  ( 97.50000000000000000, 124.1499999999999915, -1.035533905932742416 ) ) ;
#14479=CARTESIAN_POINT ( 'NONE',  ( 99.99999999999998579, 123.6069999999781572, 2.499999999999978684 ) ) ;
#14485=CARTESIAN_POINT ( 'NONE',  ( 102.1631189606246295, 103.3426043859339103, -47.90000000546238113 ) ) ;
#14493=CARTESIAN_POINT ( 'NONE',  ( 108.0825317500000011, 107.3738262389971538, -50.47500000273118559 ) ) ;
#14495=CARTESIAN_POINT ( 'NONE',  ( 97.93301269999999192, 123.0000000010925163, 0.8561741729129329626 ) ) ;
#14520=CARTESIAN_POINT ( 'NONE',  ( 97.50236033167492167, 102.3130555110000159, -48.97500000273119269 ) ) ;
#14528=CARTESIAN_POINT ( 'NONE',  ( 102.1631189606246295, 116.6573956140660897, -51.10000000546237686 ) ) ;
#14529=CARTESIAN_POINT ( 'NONE',  ( 98.15313185440925281, 93.87499999863439371, -4.458734124999994997 ) ) ;
#14532=DIRECTION ( 'NONE',  ( 5.782411586589357392E-17, -0.000000000000000000, 1.000000000000000000 ) ) ;
#14534=ADVANCED_FACE ( 'NONE', ( #8269 ), #23256, .F. ) ;
#14545=CARTESIAN_POINT ( 'NONE',  ( 106.5389055433251002, 114.7507929638356785, -48.17500000273120264 ) ) ;
#14549=CARTESIAN_POINT ( 'NONE',  ( 104.9952793366501709, 103.1245878333314465, -48.42500000273120264 ) ) ;
#14552=EDGE_CURVE ( 'NONE', #3810, #19205, #17095, .T. ) ;
#14566=DIRECTION ( 'NONE',  ( -0.000000000000000000, 1.000000000000000000, -0.000000000000000000 ) ) ;
#14567=CARTESIAN_POINT ( 'NONE',  ( 102.0669872999999797, 124.1500000010924794, -9.794112055954760458E-15 ) ) ;
#14568=CARTESIAN_POINT ( 'NONE',  ( 99.99999999999998579, 94.31249999863440792, 4.458734124999981674 ) ) ;
#14573=CARTESIAN_POINT ( 'NONE',  ( 98.53841926354351699, 123.0500000010924850, -1.461580736456474794 ) ) ;
#14578=CARTESIAN_POINT ( 'NONE',  ( 108.0825317500000153, 110.0000000000000000, -54.12500000273119838 ) ) ;
#14587=CARTESIAN_POINT ( 'NONE',  ( 96.46446609406726225, 92.49999999726880162, 3.535533905932723986 ) ) ;
#14590=CARTESIAN_POINT ( 'NONE',  ( 102.0019607628501888, 122.9999999999999858, 1.533685529140143444 ) ) ;
#14608=ORIENTED_EDGE ( 'NONE', *, *, #1945, .F. ) ;
#14612=CARTESIAN_POINT ( 'NONE',  ( 99.99999999999998579, 123.6000000000000085, 2.499999999999978684 ) ) ;
#14614=CARTESIAN_POINT ( 'NONE',  ( 99.99999999999998579, 124.5500000010924708, -2.066987299999998751 ) ) ;
#14619=CARTESIAN_POINT ( 'NONE',  ( 107.0000000000000284, 107.7255621263696952, -53.10000000000001563 ) ) ;
#14626=CARTESIAN_POINT ( 'NONE',  ( 108.0825317500000011, 107.3738262389971538, -46.47500000273117848 ) ) ;
#14628=CARTESIAN_POINT ( 'NONE',  ( 100.8561741729129153, 122.9000000010924936, -2.066987299999999195 ) ) ;
#14650=CARTESIAN_POINT ( 'NONE',  ( 101.8468681455907330, 94.49999999863439371, -4.458734124999994997 ) ) ;
#14658=CARTESIAN_POINT ( 'NONE',  ( 93.00000000000001421, 112.2744378736303332, -48.60000000546237686 ) ) ;
#14659=CARTESIAN_POINT ( 'NONE',  ( 95.54126587499999346, 93.12499999863439371, 1.846868145590722543 ) ) ;
#14663=VERTEX_POINT ( 'NONE', #23670 ) ;
#14665=CARTESIAN_POINT ( 'NONE',  ( 103.1528011352953484, 90.43749999863440792, -3.152801135295366208 ) ) ;
#14672=EDGE_LOOP ( 'NONE', ( #11730, #17395, #17721 ) ) ;
#14673=CARTESIAN_POINT ( 'NONE',  ( 91.91746824999998466, 107.3738262389971538, -49.27500000273118985 ) ) ;
#14684=AXIS2_PLACEMENT_3D ( 'NONE', #6864, #26407, #15551 ) ;
#14698=EDGE_CURVE ( 'NONE', #7889, #13118, #7692, .T. ) ;
#14699=CARTESIAN_POINT ( 'NONE',  ( 104.4587341249999781, 93.56249999863440792, -6.938893903907228378E-15 ) ) ;
#14703=CARTESIAN_POINT ( 'NONE',  ( 96.46446609406726225, 93.37500000000000000, -3.535533905932738197 ) ) ;
#14719=ORIENTED_EDGE ( 'NONE', *, *, #8283, .F. ) ;
#14739=( BOUNDED_CURVE ( )  B_SPLINE_CURVE ( 2, ( #19165, #27868, #7913, #18617, #10310, #27452, #1516, #23448, #12583 ),
 .UNSPECIFIED., .F., .F. ) 
 B_SPLINE_CURVE_WITH_KNOTS ( ( 3, 2, 2, 2, 3 ),
 ( 0.5500000000000004885, 0.5750000000000003997, 0.6000000000000005329, 0.6250000000000005551, 0.6500000000000005773 ),
 .UNSPECIFIED. ) 
 CURVE ( )  GEOMETRIC_REPRESENTATION_ITEM ( )  RATIONAL_B_SPLINE_CURVE ( ( 0.9999999999999986677, 0.9238795325112880708, 1.000000000000000000, 0.9238795325112867385, 1.000000000000000000, 0.9238795325112867385, 1.000000000000000000, 0.9238795325112850731, 1.000000000000001776 ) ) 
 REPRESENTATION_ITEM ( '' )  );
#14746=CARTESIAN_POINT ( 'NONE',  ( 99.99999999999998579, 124.3999999999999915, 2.499999999999978684 ) ) ;
#14748=CARTESIAN_POINT ( 'NONE',  ( 99.14382582708708469, 124.1000000010924822, 2.066987299999979655 ) ) ;
#14749=AXIS2_PLACEMENT_3D ( 'NONE', #21848, #26403, #26111 ) ;
#14754=CARTESIAN_POINT ( 'NONE',  ( 93.00000000000000000, 107.7255621263696668, -53.90000000000000568 ) ) ;
#14761=CARTESIAN_POINT ( 'NONE',  ( 104.9952793366501851, 116.8754121666685393, -46.07500000273119412 ) ) ;
#14762=CARTESIAN_POINT ( 'NONE',  ( 107.0000000000000142, 110.0000000000000000, -47.50000000546238255 ) ) ;
#14764=CARTESIAN_POINT ( 'NONE',  ( 101.4615807364564546, 122.6500000010924794, -1.461580736456474794 ) ) ;
#14772=CARTESIAN_POINT ( 'NONE',  ( 104.9999999999999858, 95.00000000000000000, -6.938893903907228378E-15 ) ) ;
#14776=VERTEX_POINT ( 'NONE', #26664 ) ;
#14782=DIRECTION ( 'NONE',  ( 5.782411586589357392E-17, -0.000000000000000000, 1.000000000000000000 ) ) ;
#14784=CARTESIAN_POINT ( 'NONE',  ( 95.54126587500000767, 92.81249999863440792, -7.484931351350258973E-15 ) ) ;
#14793=CARTESIAN_POINT ( 'NONE',  ( 94.33688103937537051, 114.1144967660473242, -44.70000000546237828 ) ) ;
#14794=CARTESIAN_POINT ( 'NONE',  ( 104.4587341249999923, 91.24999999863439371, 1.846868145590726318 ) ) ;
#14805=ORIENTED_EDGE ( 'NONE', *, *, #25389, .F. ) ;
#14823=CARTESIAN_POINT ( 'NONE',  ( 94.33688103937537051, 114.1144967660473242, -46.20000000000000284 ) ) ;
#14825=CARTESIAN_POINT ( 'NONE',  ( 93.46109445667491400, 105.2492070361643215, -52.92500000273119554 ) ) ;
#14834=CARTESIAN_POINT ( 'NONE',  ( 98.53841926354351699, 124.4500000010924765, -1.461580736456474794 ) ) ;
#14835=CARTESIAN_POINT ( 'NONE',  ( 93.00000000000000000, 110.0000000000000000, -46.00000000000000711 ) ) ;
#14846=CARTESIAN_POINT ( 'NONE',  ( 107.0000000000000142, 112.2744378736303332, -52.90000000000001279 ) ) ;
#14848=CARTESIAN_POINT ( 'NONE',  ( 102.0669872999999797, 124.3500000010924822, -9.794112055954760458E-15 ) ) ;
#14853=ADVANCED_FACE ( 'NONE', ( #4855 ), #17666, .T. ) ;
#14863=CARTESIAN_POINT ( 'NONE',  ( 95.00000000000000000, 92.31249999726880162, -2.071067811865479058 ) ) ;
#14864=CARTESIAN_POINT ( 'NONE',  ( 107.0000000000000142, 110.0000000000000000, -51.50000000546237544 ) ) ;
#14884=CARTESIAN_POINT ( 'NONE',  ( 99.99999999999998579, 110.0000000000000000, -43.00000000000000000 ) ) ;
#14886=LINE ( 'NONE', #86, #20669 ) ;
#14887=CARTESIAN_POINT ( 'NONE',  ( 99.99999999999998579, 124.1000000021849416, -2.499999999999997780 ) ) ;
#14889=CARTESIAN_POINT ( 'NONE',  ( 102.0669873000000081, 124.3000000010924708, 0.8561741729129311862 ) ) ;
#14892=CARTESIAN_POINT ( 'NONE',  ( 102.4999999999999716, 123.8500000021849416, 1.035533905932722876 ) ) ;
#14900=CARTESIAN_POINT ( 'NONE',  ( 97.50236033167492167, 102.3130555110000159, -48.97500000273119269 ) ) ;
#14902=EDGE_LOOP ( 'NONE', ( #18741, #7543, #4000, #25708 ) ) ;
#14907=VERTEX_POINT ( 'NONE', #16090 ) ;
#14909=( BOUNDED_CURVE ( )  B_SPLINE_CURVE ( 2, ( #21737, #10876, #4202, #6332, #26288, #22012, #17298, #4625, #19585, #6606, #28007 ),
 .UNSPECIFIED., .F., .F. ) 
 B_SPLINE_CURVE_WITH_KNOTS ( ( 3, 2, 2, 2, 2, 3 ),
 ( 0.4999999999999996669, 0.5199999999999996847, 0.5399999999999998135, 0.5599999999999998312, 0.5799999999999998490, 0.5999999999999998668 ),
 .UNSPECIFIED. ) 
 CURVE ( )  GEOMETRIC_REPRESENTATION_ITEM ( )  RATIONAL_B_SPLINE_CURVE ( ( 1.000000000000000888, 0.9510565162951527540, 1.000000000000000000, 0.9510565162951535312, 1.000000000000000000, 0.9510565162951535312, 1.000000000000000000, 0.9510565162951535312, 1.000000000000000000, 0.9510565162951537532, 0.9999999999999997780 ) ) 
 REPRESENTATION_ITEM ( '' )  );
#14918=CARTESIAN_POINT ( 'NONE',  ( 107.0000000000000142, 110.0000000000000000, -47.50000000546238255 ) ) ;
#14925=CARTESIAN_POINT ( 'NONE',  ( 97.50000000000000000, 122.7000000021849502, -9.540979117872439019E-15 ) ) ;
#14936=CARTESIAN_POINT ( 'NONE',  ( 95.54126587499999346, 94.87499999863440792, 1.846868145590722543 ) ) ;
#14946=EDGE_LOOP ( 'NONE', ( #9620, #8904, #2057, #18467 ) ) ;
#14962=STYLED_ITEM ( 'NONE', ( #27175 ), #19902 ) ;
#14970=CARTESIAN_POINT ( 'NONE',  ( 91.91746824999999887, 110.0000000000000000, -51.12500000273119127 ) ) ;
#14989=CARTESIAN_POINT ( 'NONE',  ( 107.0000000000000142, 107.7255621263696526, -49.10000000000000853 ) ) ;
#14991=CARTESIAN_POINT ( 'NONE',  ( 100.8561741729129153, 124.5000000010924737, -2.066987299999999195 ) ) ;
#15009=COLOUR_RGB ( '', 0.08235294, 0.09019608, 0.10196078) ;
#15017=CARTESIAN_POINT ( 'NONE',  ( 92.99999999999997158, 107.7255621263696810, -46.40000000546236691 ) ) ;
#15021=DIRECTION ( 'NONE',  ( 0.000000000000000000, 0.000000000000000000, 1.000000000000000000 ) ) ;
#15027=CARTESIAN_POINT ( 'NONE',  ( 99.99999999999998579, 90.75000000000000000, 4.999999999999984013 ) ) ;
#15036=CARTESIAN_POINT ( 'NONE',  ( 100.0000000000000000, 110.0000000000000000, -45.00000000000000711 ) ) ;
#15039=CARTESIAN_POINT ( 'NONE',  ( 91.91746824999998466, 112.6261737610028320, -53.22500000273119269 ) ) ;
#15062=DIRECTION ( 'NONE',  ( 0.000000000000000000, 0.000000000000000000, 1.000000000000000000 ) ) ;
#15068=CARTESIAN_POINT ( 'NONE',  ( 95.00472066334981491, 103.1245878333314465, -47.07500000273119412 ) ) ;
#15069=DIRECTION ( 'NONE',  ( 1.000000000000000000, 0.000000000000000000, -5.782411586589357392E-17 ) ) ;
#15074=CARTESIAN_POINT ( 'NONE',  ( 99.99999999999998579, 94.06249999863440792, 4.458734124999981674 ) ) ;
#15075=CARTESIAN_POINT ( 'NONE',  ( 95.00000000000000000, 93.43749999726880162, 2.071067811865463959 ) ) ;
#15077=CARTESIAN_POINT ( 'NONE',  ( 95.67376207875072680, 104.0454443415356991, -45.70000000000000284 ) ) ;
#15080=CARTESIAN_POINT ( 'NONE',  ( 103.1528011352953484, 95.18749999863440792, 3.152801135295352886 ) ) ;
#15081=EDGE_LOOP ( 'NONE', ( #14205, #17585, #23555, #5056 ) ) ;
#15086=ADVANCED_FACE ( 'NONE', ( #17885 ), #13731, .F. ) ;
#15112=CARTESIAN_POINT ( 'NONE',  ( 99.99999999999998579, 90.00000000000000000, -6.938893903907228378E-15 ) ) ;
#15121=VERTEX_POINT ( 'NONE', #15593 ) ;
#15122=CARTESIAN_POINT ( 'NONE',  ( 94.33688103937537051, 105.8855032339526758, -53.80000000000000426 ) ) ;
#15124=CARTESIAN_POINT ( 'NONE',  ( 98.53841926354351699, 123.0500000010924850, -1.461580736456474794 ) ) ;
#15132=EDGE_CURVE ( 'NONE', #8293, #2910, #22454, .T. ) ;
#15133=ORIENTED_EDGE ( 'NONE', *, *, #7065, .T. ) ;
#15155=CARTESIAN_POINT ( 'NONE',  ( 103.5355338419364699, 95.00000000000001421, -3.535533969929001596 ) ) ;
#15160=CARTESIAN_POINT ( 'NONE',  ( 99.99999999999998579, 101.5015231886685712, -52.62500000273118417 ) ) ;
#15162=CARTESIAN_POINT ( 'NONE',  ( 98.23223304703363112, 124.1000000000000085, -1.767766952966370209 ) ) ;
#15163=CARTESIAN_POINT ( 'NONE',  ( 102.4999999999999858, 122.3000000021849587, -9.847140817659276890E-15 ) ) ;
#15170=CARTESIAN_POINT ( 'NONE',  ( 102.4999999999999858, 122.3000000021849587, -9.847140817659276890E-15 ) ) ;
#15174=DIRECTION ( 'NONE',  ( -5.782411586589357392E-17, 0.000000000000000000, -1.000000000000000000 ) ) ;
#15177=CARTESIAN_POINT ( 'NONE',  ( 93.46109445667491400, 114.7507929638356785, -49.32500000273120122 ) ) ;
#15179=ORIENTED_EDGE ( 'NONE', *, *, #20148, .F. ) ;
#15184=VERTEX_POINT ( 'NONE', #18169 ) ;
#15191=CARTESIAN_POINT ( 'NONE',  ( 112.9999999999999858, 0.000000000000000000, -8.673617379884035472E-16 ) ) ;
#15201=DIRECTION ( 'NONE',  ( 0.000000000000000000, 0.000000000000000000, -1.000000000000000000 ) ) ;
#15204=CARTESIAN_POINT ( 'NONE',  ( 84.99999999999998579, 120.0000000000000000, -15.00000000000000533 ) ) ;
#15211=ADVANCED_FACE ( 'NONE', ( #11733 ), #20457, .F. ) ;
#15214=CARTESIAN_POINT ( 'NONE',  ( 104.4587341249999781, 93.31249999863440792, -6.938893903907228378E-15 ) ) ;
#15222=CARTESIAN_POINT ( 'NONE',  ( 96.84719886470463734, 94.93749999863440792, 3.152801135295351997 ) ) ;
#15224=VERTEX_POINT ( 'NONE', #14578 ) ;
#15238=CARTESIAN_POINT ( 'NONE',  ( 102.4999999999999858, 122.3000000021849587, -9.847140817659276890E-15 ) ) ;
#15244=CARTESIAN_POINT ( 'NONE',  ( 107.0000000000000142, 110.0000000000000000, -47.00000000000000711 ) ) ;
#15247=CARTESIAN_POINT ( 'NONE',  ( 93.46109445667491400, 114.7507929638356785, -53.32500000273119412 ) ) ;
#15248=CARTESIAN_POINT ( 'NONE',  ( 84.99999999999998579, 125.0000000000000000, 14.99999999999999112 ) ) ;
#15258=CARTESIAN_POINT ( 'NONE',  ( 93.00000000000000000, 110.0000000000000000, -54.00000000000000711 ) ) ;
#15265=ORIENTED_EDGE ( 'NONE', *, *, #8133, .T. ) ;
#15266=CARTESIAN_POINT ( 'NONE',  ( 102.1631189606246295, 116.6573956140660897, -48.60000000000000142 ) ) ;
#15272=CARTESIAN_POINT ( 'NONE',  ( 97.92893218813452449, 94.56249999726883004, 4.999999999999983125 ) ) ;
#15284=CARTESIAN_POINT ( 'NONE',  ( 99.99999999999998579, 94.75000000000000000, 4.999999999999984013 ) ) ;
#15296=ORIENTED_EDGE ( 'NONE', *, *, #6126, .F. ) ;
#15308=CARTESIAN_POINT ( 'NONE',  ( 91.91746824999998466, 107.3738262389971680, -51.02500000273119696 ) ) ;
#15316=CARTESIAN_POINT ( 'NONE',  ( 97.50000000000000000, 122.7500000021849615, 1.035533905932725096 ) ) ;
#15320=PLANE ( 'NONE',  #379 ) ;
#15323=( BOUNDED_CURVE ( )  B_SPLINE_CURVE ( 2, ( #19500, #6522, #4398, #21789, #2269, #10373, #14925, #4120, #10928, #8528, #23645, #19638, #3983, #3839, #12785 ),
 .UNSPECIFIED., .F., .T. ) 
 B_SPLINE_CURVE_WITH_KNOTS ( ( 3, 2, 2, 2, 2, 2, 2, 3 ),
 ( 0.5416666676520737189, 0.5833333333333333703, 0.6250000000000000000, 0.6666666666666666297, 0.7083333333333333703, 0.7500000000000000000, 0.7916666666666666297, 0.8333333333333333703 ),
 .UNSPECIFIED. ) 
 CURVE ( )  GEOMETRIC_REPRESENTATION_ITEM ( )  RATIONAL_B_SPLINE_CURVE ( ( 1.000000000000000000, 0.9238795325112867385, 1.000000000000000000, 0.9238795325112867385, 1.000000000000000000, 0.9238795325112867385, 1.000000000000000000, 0.9238795325112867385, 1.000000000000000000, 0.9238795325112867385, 1.000000000000000000, 0.9238795325112867385, 1.000000000000000000, 0.9238795325112867385, 1.000000000000000000 ) ) 
 REPRESENTATION_ITEM ( '' )  );
#15324=CARTESIAN_POINT ( 'NONE',  ( 93.46109445667491400, 105.2492070361643215, -48.92500000273119554 ) ) ;
#15354=DIRECTION ( 'NONE',  ( -5.782411586589357392E-17, -0.000000000000000000, -1.000000000000000000 ) ) ;
#15358=CARTESIAN_POINT ( 'NONE',  ( 95.67376207875072680, 115.9545556584642867, -44.80000000546236549 ) ) ;
#15359=CARTESIAN_POINT ( 'NONE',  ( 101.8468681455907330, 93.49999999863442213, -4.458734124999994997 ) ) ;
#15366=CARTESIAN_POINT ( 'NONE',  ( 104.4587341249999923, 94.24999999863439371, 1.846868145590726318 ) ) ;
#15368=AXIS2_PLACEMENT_3D ( 'NONE', #5820, #3815, #1685 ) ;
#15372=EDGE_CURVE ( 'NONE', #8183, #210, #622, .T. ) ;
#15387=CARTESIAN_POINT ( 'NONE',  ( 104.9999999999999716, 92.06249999999998579, -2.071067811865478170 ) ) ;
#15393=CARTESIAN_POINT ( 'NONE',  ( 104.9952793366501851, 116.8754121666685393, -53.82500000273119412 ) ) ;
#15394=AXIS2_PLACEMENT_3D ( 'NONE', #25428, #5769, #21290 ) ;
#15400=ORIENTED_EDGE ( 'NONE', *, *, #25502, .F. ) ;
#15401=CARTESIAN_POINT ( 'NONE',  ( 107.0000000000000142, 110.0000000000000000, -51.50000000546237544 ) ) ;
#15402=DIRECTION ( 'NONE',  ( 0.000000000000000000, -1.000000000000000000, 3.469446951953611231E-16 ) ) ;
#15406=ADVANCED_FACE ( 'NONE', ( #189 ), #25166, .F. ) ;
#15411=CARTESIAN_POINT ( 'NONE',  ( 107.0000000000000142, 110.0000000000000000, -49.00000000000000711 ) ) ;
#15414=CARTESIAN_POINT ( 'NONE',  ( 99.99999999999998579, 122.9500000010924765, -2.066987299999998751 ) ) ;
#15418=CARTESIAN_POINT ( 'NONE',  ( 95.00000000000000000, 92.43749999726878741, 2.071067811865463959 ) ) ;
#15427=CARTESIAN_POINT ( 'NONE',  ( 102.0710678118655181, 94.81250000000000000, 4.999999999999919176 ) ) ;
#15452=CARTESIAN_POINT ( 'NONE',  ( 99.99999999999998579, 118.4984768113314146, -53.62500000273119838 ) ) ;
#15453=ORIENTED_EDGE ( 'NONE', *, *, #8987, .T. ) ;
#15455=CARTESIAN_POINT ( 'NONE',  ( 97.50000000000000000, 123.5500000021849587, 1.035533905932725096 ) ) ;
#15459=CARTESIAN_POINT ( 'NONE',  ( 102.4999999999999716, 123.0500000021849445, 1.035533905932722876 ) ) ;
#15466=CARTESIAN_POINT ( 'NONE',  ( 97.50236033167492167, 102.3130555110000159, -44.97500000273119980 ) ) ;
#15472=ORIENTED_EDGE ( 'NONE', *, *, #15947, .F. ) ;
#15487=DIRECTION ( 'NONE',  ( 5.782411586589357392E-17, 0.000000000000000000, 1.000000000000000000 ) ) ;
#15506=CARTESIAN_POINT ( 'NONE',  ( 101.1641122485766999, 123.0000000000000284, -2.217301332870669217 ) ) ;
#15508=CARTESIAN_POINT ( 'NONE',  ( 96.46446609406726225, 93.24999999726881583, -3.535533905932738197 ) ) ;
#15514=VECTOR ( 'NONE', #23993, 1000.000000000000000 ) ;
#15516=CARTESIAN_POINT ( 'NONE',  ( 104.4587341249999923, 93.37499999863439371, -1.846868145590737198 ) ) ;
#15517=CARTESIAN_POINT ( 'NONE',  ( 103.1528011352953484, 94.68749999863440792, -3.152801135295366208 ) ) ;
#15520=EDGE_LOOP ( 'NONE', ( #3730, #16724, #25523, #11474 ) ) ;
#15538=CARTESIAN_POINT ( 'NONE',  ( 104.3262379212492590, 115.9545556584642867, -53.20000000546237118 ) ) ;
#15539=LINE ( 'NONE', #4306, #4530 ) ;
#15540=CARTESIAN_POINT ( 'NONE',  ( 107.5412658750000077, 110.0000000000000000, -44.68750000136559919 ) ) ;
#15545=EDGE_CURVE ( 'NONE', #7822, #20854, #24835, .T. ) ;
#15548=FACE_OUTER_BOUND ( 'NONE', #3065, .T. ) ;
#15551=DIRECTION ( 'NONE',  ( 1.000000000000000000, 0.000000000000000000, 0.000000000000000000 ) ) ;
#15555=CARTESIAN_POINT ( 'NONE',  ( 95.00472066334982912, 103.1245878333314323, -51.07500000273118701 ) ) ;
#15561=CARTESIAN_POINT ( 'NONE',  ( 104.9999999999999716, 91.93749999726880162, -2.071067811865478170 ) ) ;
#15573=CARTESIAN_POINT ( 'NONE',  ( 99.99999999999998579, 91.25000000000000000, -4.999999999999997335 ) ) ;
#15575=ADVANCED_FACE ( 'NONE', ( #3736 ), #20984, .T. ) ;
#15577=CARTESIAN_POINT ( 'NONE',  ( 101.8468681455907330, 90.74999999863439371, -4.458734124999994997 ) ) ;
#15593=CARTESIAN_POINT ( 'NONE',  ( 99.99999988184244160, 117.0000000000000000, -45.00000000000000711 ) ) ;
#15595=CARTESIAN_POINT ( 'NONE',  ( 93.46109445667491400, 105.2492070361643215, -52.92500000273119554 ) ) ;
#15596=LINE ( 'NONE', #20175, #8350 ) ;
#15597=DIRECTION ( 'NONE',  ( -0.000000000000000000, 1.000000000000000000, -0.000000000000000000 ) ) ;
#15604=CARTESIAN_POINT ( 'NONE',  ( 102.0669872999999939, 123.3000000010924850, 0.8561741729129311862 ) ) ;
#15607=VECTOR ( 'NONE', #2985, 1000.000000000000000 ) ;
#15613=CARTESIAN_POINT ( 'NONE',  ( 102.4976396683250925, 117.6869444889999841, -51.72500000273119980 ) ) ;
#15630=ORIENTED_EDGE ( 'NONE', *, *, #23425, .T. ) ;
#15633=CARTESIAN_POINT ( 'NONE',  ( 101.7677669529663547, 123.8000000021849587, 1.767766952966350891 ) ) ;
#15645=CARTESIAN_POINT ( 'NONE',  ( 93.00000000000000000, 110.0000000000000000, -54.00000000000000711 ) ) ;
#15649=CARTESIAN_POINT ( 'NONE',  ( 93.46109445667491400, 114.7507929638356785, -47.57500000273119412 ) ) ;
#15653=CARTESIAN_POINT ( 'NONE',  ( 101.5239092622869492, 123.0000000000000284, -1.987527404725653035 ) ) ;
#15654=CARTESIAN_POINT ( 'NONE',  ( 99.99999999999998579, 90.00000000000000000, -4.999999999999996447 ) ) ;
#15662=CARTESIAN_POINT ( 'NONE',  ( 103.1528011352953484, 92.18749999863440792, 3.152801135295352886 ) ) ;
#15685=CARTESIAN_POINT ( 'NONE',  ( 95.00472066334982912, 103.1245878333314323, -46.82500000273118701 ) ) ;
#15693=CARTESIAN_POINT ( 'NONE',  ( 99.14382582708708469, 122.8000000010924708, -2.066987299999998751 ) ) ;
#15701=CARTESIAN_POINT ( 'NONE',  ( 102.1631189606246295, 103.3426043859339103, -47.40000000000000568 ) ) ;
#15704=CARTESIAN_POINT ( 'NONE',  ( 101.0355339059327378, 124.7500000000000142, -2.499999999999997780 ) ) ;
#15706=DIRECTION ( 'NONE',  ( 0.000000000000000000, 1.000000000000000000, -1.156482317317871478E-16 ) ) ;
#15707=CARTESIAN_POINT ( 'NONE',  ( 97.92893218813452449, 94.18749999726880162, -4.999999999999997335 ) ) ;
#15710=CARTESIAN_POINT ( 'NONE',  ( 93.46109445667491400, 114.7507929638356785, -51.57500000273120122 ) ) ;
#15717=PLANE ( 'NONE',  #26076 ) ;
#15722=CARTESIAN_POINT ( 'NONE',  ( 99.99999999999998579, 90.81249999863440792, -4.458734124999994997 ) ) ;
#15728=VECTOR ( 'NONE', #10802, 1000.000000000000000 ) ;
#15747=CARTESIAN_POINT ( 'NONE',  ( 97.93301270000000613, 124.5500000010924850, -9.540979117872439019E-15 ) ) ;
#15755=CARTESIAN_POINT ( 'NONE',  ( 106.5389055433251002, 114.7507929638356785, -45.92500000273119554 ) ) ;
#15757=CARTESIAN_POINT ( 'NONE',  ( 105.6631189606246295, 114.1144967660473242, -49.30000000546237970 ) ) ;
#15769=CARTESIAN_POINT ( 'NONE',  ( 100.0000000000000000, 110.0000000000000000, -55.00000000000000711 ) ) ;
#15777=CARTESIAN_POINT ( 'NONE',  ( 102.4999999999999716, 124.6569999999781544, -1.035533905932742638 ) ) ;
#15779=FILL_AREA_STYLE_COLOUR ( '', #15009 ) ;
#15785=CARTESIAN_POINT ( 'NONE',  ( 105.6631189606246295, 114.1144967660473242, -54.80000000000001137 ) ) ;
#15794=CARTESIAN_POINT ( 'NONE',  ( 95.00472066334982912, 103.1245878333314323, -53.07500000273118701 ) ) ;
#15795=CARTESIAN_POINT ( 'NONE',  ( 97.90609941151407725, 123.0000000000000000, 1.374260159723026176 ) ) ;
#15796=CARTESIAN_POINT ( 'NONE',  ( 100.8561741729129295, 123.2000000010924765, 2.066987299999979211 ) ) ;
#15803=CARTESIAN_POINT ( 'NONE',  ( 97.92893218813452449, 91.31250000000001421, -4.999999999999997335 ) ) ;
#15810=CARTESIAN_POINT ( 'NONE',  ( 99.99999999999998579, 95.12499999726881583, -4.999999999999997335 ) ) ;
#15820=CARTESIAN_POINT ( 'NONE',  ( 98.15313185440923860, 90.99999999863439371, 4.458734124999980786 ) ) ;
#15826=CARTESIAN_POINT ( 'NONE',  ( 99.99999999999998579, 118.4984768113314004, -47.62500000273119127 ) ) ;
#15827=CARTESIAN_POINT ( 'NONE',  ( 99.99999999999998579, 92.31249999863440792, 4.458734124999981674 ) ) ;
#15832=DIRECTION ( 'NONE',  ( -1.000000000000000000, 0.000000000000000000, 1.224646799147411139E-16 ) ) ;
#15840=CARTESIAN_POINT ( 'NONE',  ( 95.00472066334982912, 103.1245878333314323, -53.07500000273118701 ) ) ;
#15848=CARTESIAN_POINT ( 'NONE',  ( 102.0710678118654613, 95.68749999726881583, 4.999999999999983125 ) ) ;
#15851=CARTESIAN_POINT ( 'NONE',  ( 108.0825317500000011, 112.6261737610028320, -52.27500000273118275 ) ) ;
#15858=DIRECTION ( 'NONE',  ( 5.782411586589357392E-17, -0.000000000000000000, 1.000000000000000000 ) ) ;
#15875=DIRECTION ( 'NONE',  ( -0.000000000000000000, 1.000000000000000000, -0.000000000000000000 ) ) ;
#15877=CARTESIAN_POINT ( 'NONE',  ( 104.9952793366501709, 103.1245878333314465, -50.42500000273119554 ) ) ;
#15879=CYLINDRICAL_SURFACE ( 'NONE', #20989, 4.999999999999989342 ) ;
#15890=CARTESIAN_POINT ( 'NONE',  ( 98.15313185440925281, 93.99999999863439371, 4.458734124999979898 ) ) ;
#15891=CARTESIAN_POINT ( 'NONE',  ( 99.99999999999998579, 118.4984768113314004, -45.62500000273118417 ) ) ;
#15910=CARTESIAN_POINT ( 'NONE',  ( 97.50000000000000000, 124.2069999999781515, -9.540979117872439019E-15 ) ) ;
#15927=CARTESIAN_POINT ( 'NONE',  ( 95.00000000000000000, 90.50000000000000000, -7.551217303480904118E-15 ) ) ;
#15928=CARTESIAN_POINT ( 'NONE',  ( 99.67158809262824093, 122.9999999999999716, 2.482844439542343018 ) ) ;
#15931=CARTESIAN_POINT ( 'NONE',  ( 99.14382582708707048, 123.1000000010924822, 2.066987299999979211 ) ) ;
#15936=VECTOR ( 'NONE', #16033, 1000.000000000000000 ) ;
#15937=CARTESIAN_POINT ( 'NONE',  ( 96.46446609406726225, 94.37500000000000000, -3.535533905932738197 ) ) ;
#15939=CARTESIAN_POINT ( 'NONE',  ( 104.9999999999999858, 94.00000000000000000, -6.938893903907228378E-15 ) ) ;
#15941=ADVANCED_FACE ( 'NONE', ( #10651 ), #12500, .F. ) ;
#15947=EDGE_CURVE ( 'NONE', #4172, #5706, #23919, .T. ) ;
#15956=PLANE ( 'NONE',  #21335 ) ;
#15957=CARTESIAN_POINT ( 'NONE',  ( 104.4587341249999923, 92.37499999863440792, -1.846868145590737198 ) ) ;
#15958=CARTESIAN_POINT ( 'NONE',  ( 114.9999999999999858, 125.0000000000000000, 14.99999999999998934 ) ) ;
#15965=CARTESIAN_POINT ( 'NONE',  ( 104.9952793366501851, 116.8754121666685393, -47.82500000273119412 ) ) ;
#15972=DIRECTION ( 'NONE',  ( 1.000000000000000000, 0.000000000000000000, -5.782411586589357392E-17 ) ) ;
#15974=AXIS2_PLACEMENT_3D ( 'NONE', #23777, #8806, #2549 ) ;
#15980=CARTESIAN_POINT ( 'NONE',  ( 91.91746824999999887, 110.0000000000000000, -53.37500000273119838 ) ) ;
#15987=CARTESIAN_POINT ( 'NONE',  ( 101.8468681455907330, 92.37499999863440792, 4.458734124999979898 ) ) ;
#15989=CARTESIAN_POINT ( 'NONE',  ( 95.00472066334981491, 116.8754121666685393, -53.67500000273118843 ) ) ;
#16000=ORIENTED_EDGE ( 'NONE', *, *, #10691, .T. ) ;
#16002=CARTESIAN_POINT ( 'NONE',  ( 104.4587341249999781, 90.56249999863440792, -6.938893903907228378E-15 ) ) ;
#16017=CARTESIAN_POINT ( 'NONE',  ( 108.0825317500000011, 112.6261737610028320, -48.02500000273118985 ) ) ;
#16019=CARTESIAN_POINT ( 'NONE',  ( 108.0825317500000153, 110.0000000000000000, -44.25000000273119838 ) ) ;
#16033=DIRECTION ( 'NONE',  ( 0.000000000000000000, 0.000000000000000000, -1.000000000000000000 ) ) ;
#16035=LINE ( 'NONE', #7197, #10268 ) ;
#16046=B_SPLINE_CURVE_WITH_KNOTS ( 'NONE', 3,
 ( #8468, #17156, #23311, #10168 ),
 .UNSPECIFIED., .F., .F.,
 ( 4, 4 ),
 ( 0.000000000000000000, 1.000000000000000000 ),
 .UNSPECIFIED. ) ;
#16052=DIRECTION ( 'NONE',  ( -0.000000000000000000, 1.000000000000000000, -0.000000000000000000 ) ) ;
#16054=EDGE_CURVE ( 'NONE', #10198, #17238, #15323, .T. ) ;
#16073=CARTESIAN_POINT ( 'NONE',  ( 84.99999999999998579, 120.0000000000000000, -45.00000000000000711 ) ) ;
#16082=CARTESIAN_POINT ( 'NONE',  ( 103.5355339059327235, 93.87500000000000000, 3.535533905932724874 ) ) ;
#16090=CARTESIAN_POINT ( 'NONE',  ( 104.9999999999999858, 95.00000000000000000, -6.938893903907228378E-15 ) ) ;
#16100=EDGE_CURVE ( 'NONE', #11653, #24722, #6860, .T. ) ;
#16102=CARTESIAN_POINT ( 'NONE',  ( 96.84719886470463734, 91.68749999863440792, -3.152801135295366208 ) ) ;
#16110=CARTESIAN_POINT ( 'NONE',  ( 108.0825317500000153, 110.0000000000000000, -48.12500000273119838 ) ) ;
#16111=CARTESIAN_POINT ( 'NONE',  ( 95.54126587499999346, 91.12499999863439371, 1.846868145590722543 ) ) ;
#16126=CARTESIAN_POINT ( 'NONE',  ( 104.9952793366501851, 103.1245878333314323, -52.67500000273119554 ) ) ;
#16135=CARTESIAN_POINT ( 'NONE',  ( 101.8468681455907330, 91.37499999863439371, 4.458734124999979898 ) ) ;
#16137=CARTESIAN_POINT ( 'NONE',  ( 106.5389055433251002, 114.7507929638356785, -48.17500000273120264 ) ) ;
#16148=CARTESIAN_POINT ( 'NONE',  ( 104.4587341249999923, 92.49999999863440792, 1.846868145590726318 ) ) ;
#16158=DIRECTION ( 'NONE',  ( 0.000000000000000000, 0.000000000000000000, 1.000000000000000000 ) ) ;
#16165=CARTESIAN_POINT ( 'NONE',  ( 106.5389055433251002, 105.2492070361643215, -46.32500000273119412 ) ) ;
#16176=CARTESIAN_POINT ( 'NONE',  ( 93.00000000000000000, 110.0000000000000000, -55.00000000000000711 ) ) ;
#16178=CARTESIAN_POINT ( 'NONE',  ( 103.5355339059327235, 95.74999999726881583, 3.535533905932724874 ) ) ;
#16180=CARTESIAN_POINT ( 'NONE',  ( 108.0825317500000011, 107.3738262389971538, -48.22500000273118559 ) ) ;
#16188=ORIENTED_EDGE ( 'NONE', *, *, #14552, .T. ) ;
#16195=ORIENTED_EDGE ( 'NONE', *, *, #25008, .F. ) ;
#16199=CARTESIAN_POINT ( 'NONE',  ( 99.99999999999998579, 97.00000000000000000, -6.938893903907228378E-15 ) ) ;
#16204=DIRECTION ( 'NONE',  ( 0.000000000000000000, -0.000000000000000000, 1.000000000000000000 ) ) ;
#16212=LINE ( 'NONE', #20360, #19349 ) ;
#16221=CARTESIAN_POINT ( 'NONE',  ( 102.4976396683250925, 117.6869444889999841, -53.97500000273119980 ) ) ;
#16234=CIRCLE ( 'NONE', #4870, 2.999999999999989786 ) ;
#16235=CARTESIAN_POINT ( 'NONE',  ( 103.5355339059327235, 91.87500000000000000, 3.535533905932724874 ) ) ;
#16256=CARTESIAN_POINT ( 'NONE',  ( 97.83688103937537051, 103.3426043859339103, -50.10000000546237686 ) ) ;
#16257=CARTESIAN_POINT ( 'NONE',  ( 99.99999999999998579, 91.31249999863440792, 4.458734124999981674 ) ) ;
#16264=CIRCLE ( 'NONE', #19903, 5.000000000000004441 ) ;
#16265=CARTESIAN_POINT ( 'NONE',  ( 95.00000000000000000, 91.50000000000000000, -7.551217303480904118E-15 ) ) ;
#16267=EDGE_CURVE ( 'NONE', #8723, #4009, #9344, .T. ) ;
#16269=ORIENTED_EDGE ( 'NONE', *, *, #25502, .T. ) ;
#16273=CARTESIAN_POINT ( 'NONE',  ( 93.46109445667491400, 114.7507929638356785, -45.57500000273119412 ) ) ;
#16281=CARTESIAN_POINT ( 'NONE',  ( 99.99999999999998579, 91.81249999863440792, -4.458734124999994997 ) ) ;
#16283=CARTESIAN_POINT ( 'NONE',  ( 97.50236033167492167, 117.6869444889999841, -49.77500000273119696 ) ) ;
#16291=ORIENTED_EDGE ( 'NONE', *, *, #1505, .F. ) ;
#16307=AXIS2_PLACEMENT_3D ( 'NONE', #10005, #5753, #17898 ) ;
#16317=DIRECTION ( 'NONE',  ( 0.000000000000000000, -1.000000000000000000, -0.000000000000000000 ) ) ;
#16319=ORIENTED_EDGE ( 'NONE', *, *, #25549, .F. ) ;
#16327=CARTESIAN_POINT ( 'NONE',  ( 102.0710678118654329, 92.06249999726878741, -5.000000000000011546 ) ) ;
#16345=PLANE ( 'NONE',  #18953 ) ;
#16350=CARTESIAN_POINT ( 'NONE',  ( 97.50000000000000000, 125.0069999999781629, -9.540979117872439019E-15 ) ) ;
#16351=VECTOR ( 'NONE', #14566, 1000.000000000000000 ) ;
#16354=CARTESIAN_POINT ( 'NONE',  ( 104.3262379212492590, 104.0454443415356991, -47.30000000000000426 ) ) ;
#16355=DIRECTION ( 'NONE',  ( 0.000000000000000000, 0.000000000000000000, 1.000000000000000000 ) ) ;
#16365=CARTESIAN_POINT ( 'NONE',  ( 101.7677669209684552, 123.0000000000000000, 1.767766984964258992 ) ) ;
#16374=CARTESIAN_POINT ( 'NONE',  ( 99.99999999999998579, 91.25000000000000000, -4.999999999999997335 ) ) ;
#16375=VECTOR ( 'NONE', #8369, 1000.000000000000000 ) ;
#16393=CARTESIAN_POINT ( 'NONE',  ( 103.1528011352953484, 92.18749999863440792, 3.152801135295352886 ) ) ;
#16402=CARTESIAN_POINT ( 'NONE',  ( 99.99999999999998579, 102.6397644303321215, -52.00000000546236834 ) ) ;
#16403=CARTESIAN_POINT ( 'NONE',  ( 101.8468681455907330, 90.49999999863442213, -4.458734124999994997 ) ) ;
#16408=CARTESIAN_POINT ( 'NONE',  ( 114.9999999999999858, 95.00000000000000000, 14.99999999999999289 ) ) ;
#16411=ORIENTED_EDGE ( 'NONE', *, *, #23294, .T. ) ;
#16415=CARTESIAN_POINT ( 'NONE',  ( 91.91746824999999887, 110.0000000000000000, -45.37500000273119838 ) ) ;
#16421=CARTESIAN_POINT ( 'NONE',  ( 99.99999999999998579, 93.31249999863440792, 4.458734124999981674 ) ) ;
#16433=CARTESIAN_POINT ( 'NONE',  ( 98.15313185440923860, 95.24999999863437949, 4.458734124999980786 ) ) ;
#16437=FACE_OUTER_BOUND ( 'NONE', #22956, .T. ) ;
#16450=EDGE_CURVE ( 'NONE', #19200, #4367, #12406, .T. ) ;
#16462=CARTESIAN_POINT ( 'NONE',  ( 104.9999999999999716, 91.93749999726880162, -2.071067811865478170 ) ) ;
#16481=DIRECTION ( 'NONE',  ( -0.000000000000000000, -1.000000000000000000, -0.000000000000000000 ) ) ;
#16488=CARTESIAN_POINT ( 'NONE',  ( 101.7677669529663547, 123.7000000000000028, 1.767766952966350891 ) ) ;
#16492=ADVANCED_FACE ( 'NONE', ( #16726 ), #27162, .T. ) ;
#16495=CARTESIAN_POINT ( 'NONE',  ( 107.0000000000000000, 107.7255621263696241, -47.60000000546237686 ) ) ;
#16504=FACE_OUTER_BOUND ( 'NONE', #5205, .T. ) ;
#16507=CARTESIAN_POINT ( 'NONE',  ( 97.50236033167492167, 117.6869444889999841, -45.77500000273119696 ) ) ;
#16508=CARTESIAN_POINT ( 'NONE',  ( 99.99999999999998579, 93.74999999999998579, 4.999999999999984013 ) ) ;
#16510=CARTESIAN_POINT ( 'NONE',  ( 99.99999999999998579, 122.7500000010924879, -2.066987299999998751 ) ) ;
#16522=ORIENTED_EDGE ( 'NONE', *, *, #25146, .T. ) ;
#16534=CARTESIAN_POINT ( 'NONE',  ( 103.1528011352953484, 94.43749999863440792, -3.152801135295366208 ) ) ;
#16537=EDGE_CURVE ( 'NONE', #17550, #15224, #7463, .T. ) ;
#16543=CARTESIAN_POINT ( 'NONE',  ( 102.1631189606246295, 116.6573956140660897, -47.10000000546237686 ) ) ;
#16544=CARTESIAN_POINT ( 'NONE',  ( 96.84719886470463734, 94.93749999863440792, -3.152801135295366208 ) ) ;
#16546=DIRECTION ( 'NONE',  ( 0.000000000000000000, 1.000000000000000000, 0.000000000000000000 ) ) ;
#16550=CARTESIAN_POINT ( 'NONE',  ( 96.84719886470463734, 90.68749999863440792, -3.152801135295366208 ) ) ;
#16557=CARTESIAN_POINT ( 'NONE',  ( 95.00472066334982912, 116.8754121666685393, -45.67500000273119554 ) ) ;
#16564=CARTESIAN_POINT ( 'NONE',  ( 103.1528011352953484, 93.68749999863440792, -3.152801135295366208 ) ) ;
#16565=DIRECTION ( 'NONE',  ( 0.000000000000000000, 0.000000000000000000, 1.000000000000000000 ) ) ;
#16575=CARTESIAN_POINT ( 'NONE',  ( 99.99999999999998579, 92.81249999863440792, -4.458734124999994997 ) ) ;
#16586=ORIENTED_EDGE ( 'NONE', *, *, #14698, .T. ) ;
#16587=CARTESIAN_POINT ( 'NONE',  ( 105.6631189606246295, 114.1144967660473242, -54.80000000000001137 ) ) ;
#16592=( BOUNDED_CURVE ( )  B_SPLINE_CURVE ( 2, ( #16508, #1556, #27493, #23070, #23211, #1415, #5688, #10209, #20516 ),
 .UNSPECIFIED., .F., .F. ) 
 B_SPLINE_CURVE_WITH_KNOTS ( ( 3, 2, 2, 2, 3 ),
 ( 0.7500000000000006661, 0.7750000000000006883, 0.8000000000000007105, 0.8250000000000007327, 0.8500000000000007550 ),
 .UNSPECIFIED. ) 
 CURVE ( )  GEOMETRIC_REPRESENTATION_ITEM ( )  RATIONAL_B_SPLINE_CURVE ( ( 0.9999999999999980016, 0.9238795325112887369, 1.000000000000000000, 0.9238795325112867385, 1.000000000000000000, 0.9238795325112867385, 1.000000000000000000, 0.9238795325112844070, 1.000000000000002442 ) ) 
 REPRESENTATION_ITEM ( '' )  );
#16593=CARTESIAN_POINT ( 'NONE',  ( 93.00000000000000000, 107.7255621263696668, -44.40000000546237402 ) ) ;
#16610=ORIENTED_EDGE ( 'NONE', *, *, #9167, .T. ) ;
#16629=CARTESIAN_POINT ( 'NONE',  ( 102.4999999999999716, 123.0569999999781459, -1.035533905932742638 ) ) ;
#16637=VECTOR ( 'NONE', #24248, 999.9999999999998863 ) ;
#16645=CARTESIAN_POINT ( 'NONE',  ( 95.00472066334982912, 116.8754121666685393, -49.67500000273118843 ) ) ;
#16662=ORIENTED_EDGE ( 'NONE', *, *, #13926, .F. ) ;
#16665=CARTESIAN_POINT ( 'NONE',  ( 95.67376207875072680, 115.9545556584642867, -52.30000000000000426 ) ) ;
#16679=CARTESIAN_POINT ( 'NONE',  ( 104.3262379212492590, 104.0454443415356991, -45.80000000546238681 ) ) ;
#16680=CARTESIAN_POINT ( 'NONE',  ( 98.15313185440925281, 95.24999999863437949, 4.458734124999979898 ) ) ;
#16683=LINE ( 'NONE', #3853, #8899 ) ;
#16690=VECTOR ( 'NONE', #24522, 1000.000000000000000 ) ;
#16695=CARTESIAN_POINT ( 'NONE',  ( 91.91746824999999887, 110.0000000000000000, -49.37500000273119838 ) ) ;
#16697=AXIS2_PLACEMENT_3D ( 'NONE', #27132, #3316, #221 ) ;
#16700=CARTESIAN_POINT ( 'NONE',  ( 106.5389055433251002, 105.2492070361643215, -50.32500000273120122 ) ) ;
#16720=CARTESIAN_POINT ( 'NONE',  ( 104.4587341249999923, 92.62499999863439371, -1.846868145590737198 ) ) ;
#16724=ORIENTED_EDGE ( 'NONE', *, *, #8967, .T. ) ;
#16726=FACE_OUTER_BOUND ( 'NONE', #11365, .T. ) ;
#16729=CARTESIAN_POINT ( 'NONE',  ( 93.00000000000001421, 112.2744378736303332, -54.10000000000000853 ) ) ;
#16741=CARTESIAN_POINT ( 'NONE',  ( 94.33688103937537051, 105.8855032339526758, -52.30000000546237970 ) ) ;
#16742=CARTESIAN_POINT ( 'NONE',  ( 99.99999999999998579, 90.00000000000000000, -6.938893903907228378E-15 ) ) ;
#16744=DIRECTION ( 'NONE',  ( 0.000000000000000000, 0.000000000000000000, -1.000000000000000000 ) ) ;
#16754=( BOUNDED_CURVE ( )  B_SPLINE_CURVE ( 2, ( #3225, #11892, #19443, #1789, #10308 ),
 .UNSPECIFIED., .F., .F. ) 
 B_SPLINE_CURVE_WITH_KNOTS ( ( 3, 2, 3 ),
 ( 0.7499999999999997780, 0.7916666666666665186, 0.8333333333333333703 ),
 .UNSPECIFIED. ) 
 CURVE ( )  GEOMETRIC_REPRESENTATION_ITEM ( )  RATIONAL_B_SPLINE_CURVE ( ( 1.000000000000000444, 0.9238795325112862944, 1.000000000000000000, 0.9238795325112867385, 1.000000000000000000 ) ) 
 REPRESENTATION_ITEM ( '' )  );
#16758=CARTESIAN_POINT ( 'NONE',  ( 97.83688103937538472, 116.6573956140660897, -48.40000000000000568 ) ) ;
#16760=ORIENTED_EDGE ( 'NONE', *, *, #1510, .F. ) ;
#16764=CARTESIAN_POINT ( 'NONE',  ( 99.99999999999998579, 124.0000000000000000, -2.499999999999997780 ) ) ;
#16767=CARTESIAN_POINT ( 'NONE',  ( 97.93301270000000613, 124.7500000010924737, -9.540979117872439019E-15 ) ) ;
#16769=CARTESIAN_POINT ( 'NONE',  ( 108.0825317500000153, 110.0000000000000000, -46.37500000273119838 ) ) ;
#16773=CARTESIAN_POINT ( 'NONE',  ( 101.0355339059327378, 123.7500000021849615, 2.499999999999977796 ) ) ;
#16781=CARTESIAN_POINT ( 'NONE',  ( 91.91746824999999887, 110.0000000000000000, -49.37500000273119838 ) ) ;
#16783=CARTESIAN_POINT ( 'NONE',  ( 99.99999999999998579, 123.7500000010924737, -2.066987299999998751 ) ) ;
#16798=CARTESIAN_POINT ( 'NONE',  ( 104.3262379212492590, 115.9545556584642867, -52.70000000000000284 ) ) ;
#16807=CARTESIAN_POINT ( 'NONE',  ( 104.4587341249999781, 94.31249999863440792, -6.938893903907228378E-15 ) ) ;
#16817=CARTESIAN_POINT ( 'NONE',  ( 99.99999999999998579, 117.3602355696678501, -49.00000000546238965 ) ) ;
#16818=CARTESIAN_POINT ( 'NONE',  ( 95.54126587500000767, 90.81249999863440792, -7.484931351350258973E-15 ) ) ;
#16833=CARTESIAN_POINT ( 'NONE',  ( 93.46109445667491400, 105.2492070361643215, -47.17500000273119554 ) ) ;
#16837=CARTESIAN_POINT ( 'NONE',  ( 102.4976396683250925, 102.3130555110000159, -46.52500000273119696 ) ) ;
#16854=DIRECTION ( 'NONE',  ( -5.782411586589357392E-17, -0.000000000000000000, -1.000000000000000000 ) ) ;
#16855=CARTESIAN_POINT ( 'NONE',  ( 103.1528011352953484, 94.68749999863440792, -3.152801135295366208 ) ) ;
#16866=DIRECTION ( 'NONE',  ( 0.000000000000000000, 0.000000000000000000, 1.000000000000000000 ) ) ;
#16868=( BOUNDED_CURVE ( )  B_SPLINE_CURVE ( 2, ( #5439, #9972, #18261, #14107, #3297, #20403, #27387, #25231, #26969, #3432, #7846 ),
 .UNSPECIFIED., .F., .F. ) 
 B_SPLINE_CURVE_WITH_KNOTS ( ( 3, 2, 2, 2, 2, 3 ),
 ( 0.000000000000000000, 0.02000000000000000042, 0.04000000000000000083, 0.05999999999999999778, 0.08000000000000000167, 0.1000000000000000194 ),
 .UNSPECIFIED. ) 
 CURVE ( )  GEOMETRIC_REPRESENTATION_ITEM ( )  RATIONAL_B_SPLINE_CURVE ( ( 1.000000000000000000, 0.9510565162951535312, 1.000000000000000000, 0.9510565162951535312, 1.000000000000000000, 0.9510565162951535312, 1.000000000000000000, 0.9510565162951535312, 1.000000000000000000, 0.9510565162951535312, 1.000000000000000000 ) ) 
 REPRESENTATION_ITEM ( '' )  );
#16869=CARTESIAN_POINT ( 'NONE',  ( 107.0000000000000142, 110.0000000000000000, -43.50000000546237544 ) ) ;
#16870=DIRECTION ( 'NONE',  ( 1.000000000000000000, 0.000000000000000000, -5.782411586589357392E-17 ) ) ;
#16873=ORIENTED_EDGE ( 'NONE', *, *, #24827, .F. ) ;
#16877=CARTESIAN_POINT ( 'NONE',  ( 99.99999999999998579, 102.6397644303321215, -52.00000000546236834 ) ) ;
#16878=DIRECTION ( 'NONE',  ( -0.000000000000000000, 1.000000000000000000, -0.000000000000000000 ) ) ;
#16880=FACE_OUTER_BOUND ( 'NONE', #18320, .T. ) ;
#16897=CARTESIAN_POINT ( 'NONE',  ( 99.99999999999998579, 124.0000000000000000, -2.499999999999997780 ) ) ;
#16898=CARTESIAN_POINT ( 'NONE',  ( 98.23223304703363112, 124.8999999999999915, -1.767766952966370209 ) ) ;
#16900=CARTESIAN_POINT ( 'NONE',  ( 100.8561741729129437, 124.2000000010924623, 2.066987299999979655 ) ) ;
#16905=CARTESIAN_POINT ( 'NONE',  ( 97.83688103937537051, 103.3426043859339103, -53.60000000000000853 ) ) ;
#16912=CARTESIAN_POINT ( 'NONE',  ( 108.0825317500000011, 112.6261737610028320, -46.27500000273120406 ) ) ;
#16914=CARTESIAN_POINT ( 'NONE',  ( 102.0669872999999797, 122.7500000010924737, -9.794112055954760458E-15 ) ) ;
#16919=CARTESIAN_POINT ( 'NONE',  ( 99.99999999999998579, 92.62499999726881583, 4.999999999999984013 ) ) ;
#16935=CARTESIAN_POINT ( 'NONE',  ( 98.15313185440923860, 94.99999999863439371, 4.458734124999980786 ) ) ;
#16943=CARTESIAN_POINT ( 'NONE',  ( 109.0000000000000142, 110.0000000000000000, -55.00000000000000711 ) ) ;
#16944=CARTESIAN_POINT ( 'NONE',  ( 104.4587341249999923, 94.49999999863442213, 1.846868145590726318 ) ) ;
#16951=CARTESIAN_POINT ( 'NONE',  ( 104.4587341249999923, 90.37499999863440792, -1.846868145590737198 ) ) ;
#16966=EDGE_CURVE ( 'NONE', #13215, #12839, #5941, .T. ) ;
#16967=DIRECTION ( 'NONE',  ( 1.000000000000000000, -0.000000000000000000, -5.782411586589357392E-17 ) ) ;
#16985=DIRECTION ( 'NONE',  ( 1.000000000000000000, 0.000000000000000000, -0.000000000000000000 ) ) ;
#16990=EDGE_LOOP ( 'NONE', ( #25558, #19140, #22656, #11934 ) ) ;
#16996=CARTESIAN_POINT ( 'NONE',  ( 93.00000000000001421, 107.7255621263696668, -47.89999999999999858 ) ) ;
#16997=PLANE ( 'NONE',  #4248 ) ;
#16998=CARTESIAN_POINT ( 'NONE',  ( 99.99999999999998579, 93.12499999726881583, -4.999999999999997335 ) ) ;
#17010=CARTESIAN_POINT ( 'NONE',  ( 102.4999205310587058, 123.0000000000000000, 0.3311205932291627629 ) ) ;
#17011=CARTESIAN_POINT ( 'NONE',  ( 104.7293670624999748, 95.15624999931721106, -6.938893903907228378E-15 ) ) ;
#17015=ORIENTED_EDGE ( 'NONE', *, *, #1653, .T. ) ;
#17029=CARTESIAN_POINT ( 'NONE',  ( 98.23223304703363112, 124.8999999999999915, -1.767766952966370209 ) ) ;
#17031=CARTESIAN_POINT ( 'NONE',  ( 99.99999999999998579, 90.00000000000000000, 4.999999999999983125 ) ) ;
#17032=CARTESIAN_POINT ( 'NONE',  ( 97.50000000000000000, 125.0092387953251034, 0.1913417161825344548 ) ) ;
#17034=CARTESIAN_POINT ( 'NONE',  ( 102.0669872999999797, 124.3500000010924822, -9.794112055954760458E-15 ) ) ;
#17040=CARTESIAN_POINT ( 'NONE',  ( 102.4999999999999858, 123.9000000021849530, -9.847140817659276890E-15 ) ) ;
#17047=CARTESIAN_POINT ( 'NONE',  ( 91.91746824999998466, 112.6261737610028320, -45.47500000273119980 ) ) ;
#17049=CARTESIAN_POINT ( 'NONE',  ( 98.53841926354351699, 122.8500000010924680, -1.461580736456474794 ) ) ;
#17064=ORIENTED_EDGE ( 'NONE', *, *, #7584, .F. ) ;
#17070=CARTESIAN_POINT ( 'NONE',  ( 97.50000000000000000, 125.0000000000000000, -9.540979117872439019E-15 ) ) ;
#17072=LINE ( 'NONE', #10517, #21185 ) ;
#17082=CARTESIAN_POINT ( 'NONE',  ( 104.3262379212492590, 115.9545556584642867, -45.20000000546238539 ) ) ;
#17083=CARTESIAN_POINT ( 'NONE',  ( 98.15313185440925281, 94.62499999863439371, -4.458734124999994997 ) ) ;
#17095=LINE ( 'NONE', #17239, #26338 ) ;
#17102=CARTESIAN_POINT ( 'NONE',  ( 97.50000000000000000, 124.3000000021849587, -9.540979117872439019E-15 ) ) ;
#17106=EDGE_LOOP ( 'NONE', ( #11011, #24331, #23902, #8692 ) ) ;
#17112=CARTESIAN_POINT ( 'NONE',  ( 105.6631189606246295, 114.1144967660473242, -46.80000000000001137 ) ) ;
#17121=ORIENTED_EDGE ( 'NONE', *, *, #11906, .F. ) ;
#17137=CARTESIAN_POINT ( 'NONE',  ( 95.67376207875072680, 115.9545556584642867, -50.30000000000000426 ) ) ;
#17139=CARTESIAN_POINT ( 'NONE',  ( 99.99999999999998579, 123.3500000010924680, 2.066987299999980099 ) ) ;
#17145=VERTEX_POINT ( 'NONE', #2757 ) ;
#17147=VERTEX_POINT ( 'NONE', #20140 ) ;
#17155=CARTESIAN_POINT ( 'NONE',  ( 100.0000000000000000, 110.0000000000000000, -55.00000000000000711 ) ) ;
#17156=CARTESIAN_POINT ( 'NONE',  ( 102.3556624333333076, 122.9166666670308246, -9.829464563757769835E-15 ) ) ;
#17162=ORIENTED_EDGE ( 'NONE', *, *, #2338, .T. ) ;
#17163=( BOUNDED_CURVE ( )  B_SPLINE_CURVE ( 2, ( #27862, #8322, #6193, #14863, #12162, #10164, #14587, #12027, #23307 ),
 .UNSPECIFIED., .F., .F. ) 
 B_SPLINE_CURVE_WITH_KNOTS ( ( 3, 2, 2, 2, 3 ),
 ( 0.2500000000000002220, 0.2750000000000002442, 0.3000000000000002665, 0.3250000000000002887, 0.3500000000000003109 ),
 .UNSPECIFIED. ) 
 CURVE ( )  GEOMETRIC_REPRESENTATION_ITEM ( )  RATIONAL_B_SPLINE_CURVE ( ( 0.9999999999999993339, 0.9238795325112874046, 1.000000000000000000, 0.9238795325112867385, 1.000000000000000000, 0.9238795325112867385, 1.000000000000000000, 0.9238795325112857393, 1.000000000000001110 ) ) 
 REPRESENTATION_ITEM ( '' )  );
#17182=ORIENTED_EDGE ( 'NONE', *, *, #23604, .T. ) ;
#17183=CARTESIAN_POINT ( 'NONE',  ( 104.3262379212492590, 104.0454443415356991, -53.29999999999999716 ) ) ;
#17187=CARTESIAN_POINT ( 'NONE',  ( 112.9999999999999858, 102.0000000000000000, -43.00000000000000000 ) ) ;
#17190=CARTESIAN_POINT ( 'NONE',  ( 102.4976396683250925, 102.3130555110000159, -50.52500000273119696 ) ) ;
#17213=EDGE_LOOP ( 'NONE', ( #4329, #4032, #16411, #27091 ) ) ;
#17224=CARTESIAN_POINT ( 'NONE',  ( 102.1631189606246295, 103.3426043859339103, -43.90000000546237402 ) ) ;
#17225=CARTESIAN_POINT ( 'NONE',  ( 98.15313185440925281, 93.62499999863440792, -4.458734124999994997 ) ) ;
#17234=CARTESIAN_POINT ( 'NONE',  ( 99.99999999999998579, 95.06249999863440792, 4.458734124999981674 ) ) ;
#17238=VERTEX_POINT ( 'NONE', #15238 ) ;
#17239=CARTESIAN_POINT ( 'NONE',  ( 114.9999999999999858, 100.0000000000000000, -15.00000000000000711 ) ) ;
#17241=EDGE_CURVE ( 'NONE', #5424, #7349, #588, .T. ) ;
#17261=CARTESIAN_POINT ( 'NONE',  ( 95.00472066334982912, 116.8754121666685393, -51.42500000273118843 ) ) ;
#17273=CARTESIAN_POINT ( 'NONE',  ( 99.99999999999998579, 90.00000000000000000, -4.999999999999996447 ) ) ;
#17278=CARTESIAN_POINT ( 'NONE',  ( 102.1631189606246295, 103.3426043859339103, -53.40000000000001279 ) ) ;
#17280=CARTESIAN_POINT ( 'NONE',  ( 97.93301269999999192, 123.2000000010924765, 0.8561741729129329626 ) ) ;
#17295=DIRECTION ( 'NONE',  ( 1.000000000000000000, 0.000000000000000000, 0.000000000000000000 ) ) ;
#17296=LINE ( 'NONE', #8326, #11371 ) ;
#17298=CARTESIAN_POINT ( 'NONE',  ( 102.1631189606246295, 103.3426043859339103, -49.40000000000000568 ) ) ;
#17300=EDGE_LOOP ( 'NONE', ( #5078, #678, #19154 ) ) ;
#17309=EDGE_LOOP ( 'NONE', ( #13080, #19892, #17182, #7395, #11435, #12314, #15630, #6720 ) ) ;
#17316=CARTESIAN_POINT ( 'NONE',  ( 91.91746824999998466, 112.6261737610028320, -53.22500000273119269 ) ) ;
#17317=VECTOR ( 'NONE', #1891, 1000.000000000000000 ) ;
#17321=CARTESIAN_POINT ( 'NONE',  ( 101.0355339059327378, 122.4500000021849502, -2.499999999999997780 ) ) ;
#17322=EDGE_CURVE ( 'NONE', #7547, #17145, #25088, .T. ) ;
#17328=CARTESIAN_POINT ( 'NONE',  ( 97.50000000000000000, 122.6500000021849530, -1.035533905932742416 ) ) ;
#17330=FACE_OUTER_BOUND ( 'NONE', #2500, .T. ) ;
#17331=EDGE_CURVE ( 'NONE', #17145, #13309, #20681, .T. ) ;
#17337=CARTESIAN_POINT ( 'NONE',  ( 97.50236033167492167, 117.6869444889999841, -49.52500000273119696 ) ) ;
#17366=CARTESIAN_POINT ( 'NONE',  ( 104.9952793366501709, 116.8754121666685393, -46.07500000273119412 ) ) ;
#17371=CARTESIAN_POINT ( 'NONE',  ( 99.99999999999998579, 92.06249999863440792, 4.458734124999981674 ) ) ;
#17377=CARTESIAN_POINT ( 'NONE',  ( 103.1528011352953484, 92.43749999863440792, -3.152801135295366208 ) ) ;
#17395=ORIENTED_EDGE ( 'NONE', *, *, #1476, .F. ) ;
#17400=CYLINDRICAL_SURFACE ( 'NONE', #18534, 7.000000000000006217 ) ;
#17402=CARTESIAN_POINT ( 'NONE',  ( 91.91746824999998466, 107.3738262389971538, -51.02500000273119696 ) ) ;
#17404=DIRECTION ( 'NONE',  ( 0.000000000000000000, -1.000000000000000000, 0.000000000000000000 ) ) ;
#17410=DIRECTION ( 'NONE',  ( 0.000000000000000000, 0.000000000000000000, 1.000000000000000000 ) ) ;
#17411=B_SPLINE_CURVE_WITH_KNOTS ( 'NONE', 3,
 ( #275, #24352, #9381, #2838, #11222, #856, #18228, #13504, #24647, #15653, #4983, #15506, #4550, #26502, #17650, #19793, #4843, #9246, #20371, #22224, #22084, #7097, #4695, #18078, #7381, #11363, #2561, #13211, #24498, #21945, #9528, #19940, #9105, #2423, #7237, #17938, #15795, #26649, #13650, #26937, #22507, #11506, #8962, #26792, #15928, #26358, #6816, #6958, #24216, #419, #17799, #5553, #3126, #16365 ),
 .UNSPECIFIED., .F., .F.,
 ( 4, 2, 2, 2, 2, 2, 2, 2, 2, 2, 2, 2, 2, 2, 2, 2, 2, 2, 2, 2, 2, 2, 2, 2, 2, 2, 4 ),
 ( 0.7500000000000000000, 0.8046875000000001110, 0.8320312500000005551, 0.8593750000000011102, 0.8867187500000015543, 0.9140625000000019984, 0.9414062500000025535, 0.9687500000000029976, 1.023437500000001332, 1.050781250000000444, 1.078124999999999778, 1.105468749999998890, 1.132812499999998002, 1.187499999999996447, 1.242187499999994893, 1.269531249999994005, 1.296874999999993339, 1.324218749999992450, 1.351562499999991562, 1.378906249999990674, 1.406249999999989786, 1.460937499999990452, 1.488281249999992006, 1.515624999999993783, 1.542968749999995115, 1.570312499999996891, 1.625000000000000000 ),
 .UNSPECIFIED. ) ;
#17413=CYLINDRICAL_SURFACE ( 'NONE', #11670, 4.999999999999989342 ) ;
#17420=CARTESIAN_POINT ( 'NONE',  ( 105.6631189606246295, 105.8855032339526758, -49.20000000000000995 ) ) ;
#17422=CARTESIAN_POINT ( 'NONE',  ( 99.99999999999998579, 124.1500000010924651, 2.066987299999980099 ) ) ;
#17426=CARTESIAN_POINT ( 'NONE',  ( 103.5355339059327235, 94.99999999726881583, -3.535533905932738197 ) ) ;
#17428=LINE ( 'NONE', #26126, #15514 ) ;
#17458=CARTESIAN_POINT ( 'NONE',  ( 101.0355339059327378, 123.7500000021849615, 2.499999999999977796 ) ) ;
#17463=CARTESIAN_POINT ( 'NONE',  ( 100.8561741729129153, 124.3000000010924708, -2.066987299999999195 ) ) ;
#17465=DIRECTION ( 'NONE',  ( 5.782411586589357392E-17, -0.000000000000000000, 1.000000000000000000 ) ) ;
#17470=CARTESIAN_POINT ( 'NONE',  ( 99.99999999999998579, 118.4984768113314004, -49.62500000273118417 ) ) ;
#17486=FACE_OUTER_BOUND ( 'NONE', #493, .T. ) ;
#17504=CARTESIAN_POINT ( 'NONE',  ( 97.50236033167492167, 117.6869444889999841, -45.77500000273119696 ) ) ;
#17505=CARTESIAN_POINT ( 'NONE',  ( 101.1086910246750250, 117.0000000187143314, -45.05125428434656243 ) ) ;
#17508=CARTESIAN_POINT ( 'NONE',  ( 107.0000000000000142, 112.2744378736303332, -45.40000000546235981 ) ) ;
#17509=CARTESIAN_POINT ( 'NONE',  ( 101.8468681455907330, 95.12499999863439371, 4.458734124999979898 ) ) ;
#17510=EDGE_CURVE ( 'NONE', #21036, #11286, #1708, .T. ) ;
#17518=CARTESIAN_POINT ( 'NONE',  ( 101.8468681455907330, 94.12499999863439371, 4.458734124999979898 ) ) ;
#17520=ADVANCED_FACE ( 'NONE', ( #17635 ), #26344, .F. ) ;
#17538=DIRECTION ( 'NONE',  ( -0.000000000000000000, 1.000000000000000000, -0.000000000000000000 ) ) ;
#17542=CARTESIAN_POINT ( 'NONE',  ( 91.91746824999998466, 112.6261737610028320, -49.22500000273119269 ) ) ;
#17550=VERTEX_POINT ( 'NONE', #11349 ) ;
#17552=LINE ( 'NONE', #6717, #8416 ) ;
#17554=EDGE_CURVE ( 'NONE', #27581, #2056, #24630, .T. ) ;
#17560=EDGE_LOOP ( 'NONE', ( #17162, #13834, #19246, #2994 ) ) ;
#17561=CARTESIAN_POINT ( 'NONE',  ( 95.67376207875072680, 104.0454443415356991, -53.70000000000000284 ) ) ;
#17563=CARTESIAN_POINT ( 'NONE',  ( 99.14382582708707048, 124.6000000010924822, -2.066987299999999195 ) ) ;
#17566=CARTESIAN_POINT ( 'NONE',  ( 104.9999999999999716, 94.93749999726880162, -2.071067811865478170 ) ) ;
#17585=ORIENTED_EDGE ( 'NONE', *, *, #2308, .F. ) ;
#17593=CARTESIAN_POINT ( 'NONE',  ( 99.99999999999998579, 95.12499999726881583, -4.999999999999997335 ) ) ;
#17601=CARTESIAN_POINT ( 'NONE',  ( 102.4999999999999716, 123.8500000021849416, 1.035533905932722876 ) ) ;
#17603=( LENGTH_UNIT ( ) NAMED_UNIT ( * ) SI_UNIT ( .MILLI., .METRE. ) );
#17605=CARTESIAN_POINT ( 'NONE',  ( 98.23223304703363112, 123.4000000021849530, -1.767766952966370209 ) ) ;
#17609=DIRECTION ( 'NONE',  ( -1.000000000000000000, 0.000000000000000000, 0.000000000000000000 ) ) ;
#17612=CARTESIAN_POINT ( 'NONE',  ( 108.0825317500000153, 110.0000000000000000, -44.37500000273119838 ) ) ;
#17619=MANIFOLD_SOLID_BREP ( 'Thread3', #23114 ) ;
#17621=LINE ( 'NONE', #8931, #7727 ) ;
#17635=FACE_OUTER_BOUND ( 'NONE', #9150, .T. ) ;
#17646=CARTESIAN_POINT ( 'NONE',  ( 97.50236033167492167, 102.3130555110000159, -46.97500000273119269 ) ) ;
#17650=CARTESIAN_POINT ( 'NONE',  ( 100.6274934504576777, 123.0000000000000000, -2.424672454047630321 ) ) ;
#17659=CARTESIAN_POINT ( 'NONE',  ( 96.46446609406726225, 90.37500000000000000, -3.535533905932738197 ) ) ;
#17666=PLANE ( 'NONE',  #14030 ) ;
#17673=EDGE_LOOP ( 'NONE', ( #22700, #24450, #26264 ) ) ;
#17686=AXIS2_PLACEMENT_3D ( 'NONE', #27303, #12430, #16866 ) ;
#17690=CARTESIAN_POINT ( 'NONE',  ( 104.9952793366501851, 103.1245878333314323, -44.42500000273119554 ) ) ;
#17693=DIRECTION ( 'NONE',  ( -1.000000000000000000, 0.000000000000000000, 0.000000000000000000 ) ) ;
#17696=EDGE_CURVE ( 'NONE', #2410, #8127, #11377, .T. ) ;
#17698=ORIENTED_EDGE ( 'NONE', *, *, #19426, .F. ) ;
#17700=CARTESIAN_POINT ( 'NONE',  ( 99.14382582708708469, 123.1000000010924822, 2.066987299999979655 ) ) ;
#17708=CARTESIAN_POINT ( 'NONE',  ( 91.91746824999999887, 110.0000000000000000, -51.37500000273119127 ) ) ;
#17711=CARTESIAN_POINT ( 'NONE',  ( 97.50000000000000000, 124.2500000000000000, 1.035533905932725096 ) ) ;
#17715=CARTESIAN_POINT ( 'NONE',  ( 104.9999999999999858, 92.87499999726881583, -6.938893903907228378E-15 ) ) ;
#17720=CARTESIAN_POINT ( 'NONE',  ( 114.9999999999999858, 100.0000000000000000, -15.00000000000000711 ) ) ;
#17721=ORIENTED_EDGE ( 'NONE', *, *, #24980, .F. ) ;
#17748=CARTESIAN_POINT ( 'NONE',  ( 97.50000000000000000, 124.3092387975100621, 0.1913417161825344548 ) ) ;
#17755=ORIENTED_EDGE ( 'NONE', *, *, #6379, .F. ) ;
#17756=CARTESIAN_POINT ( 'NONE',  ( 100.8561741729129295, 124.0000000010925021, 2.066987299999979211 ) ) ;
#17763=CARTESIAN_POINT ( 'NONE',  ( 106.5389055433251002, 114.7507929638356785, -51.92500000273119554 ) ) ;
#17787=DIRECTION ( 'NONE',  ( 1.000000000000000000, 0.000000000000000000, -5.782411586589357392E-17 ) ) ;
#17795=CARTESIAN_POINT ( 'NONE',  ( 106.5389055433251002, 114.7507929638356785, -46.17500000273119554 ) ) ;
#17796=CARTESIAN_POINT ( 'NONE',  ( 105.6631189606246295, 114.1144967660473242, -45.30000000546237970 ) ) ;
#17799=CARTESIAN_POINT ( 'NONE',  ( 100.9398115314949393, 123.0000000000000000, 2.320989078743034284 ) ) ;
#17800=CARTESIAN_POINT ( 'NONE',  ( 99.99999999999998579, 93.62499999726881583, 4.999999999999984013 ) ) ;
#17808=CARTESIAN_POINT ( 'NONE',  ( 104.4587341249999923, 94.37499999863440792, -1.846868145590737198 ) ) ;
#17809=CARTESIAN_POINT ( 'NONE',  ( 98.15313185440925281, 95.24999999863437949, 4.458734124999979898 ) ) ;
#17813=CARTESIAN_POINT ( 'NONE',  ( 84.99999999999998579, 95.00000000000000000, 12.99999999999999467 ) ) ;
#17815=ORIENTED_EDGE ( 'NONE', *, *, #20062, .T. ) ;
#17823=CARTESIAN_POINT ( 'NONE',  ( 95.67376207875072680, 104.0454443415356991, -50.20000000546238539 ) ) ;
#17830=CARTESIAN_POINT ( 'NONE',  ( 99.99999999999998579, 101.5015231886685854, -48.62500000273119838 ) ) ;
#17838=CARTESIAN_POINT ( 'NONE',  ( 102.0669873000000081, 123.4000000010924794, -0.8561741729129508371 ) ) ;
#17844=ORIENTED_EDGE ( 'NONE', *, *, #23425, .F. ) ;
#17848=CARTESIAN_POINT ( 'NONE',  ( 99.99999999999998579, 118.4984768113314004, -53.87500000273118417 ) ) ;
#17850=CARTESIAN_POINT ( 'NONE',  ( 98.23223304703363112, 123.2999999999999972, -1.767766952966370209 ) ) ;
#17854=CARTESIAN_POINT ( 'NONE',  ( 95.00000000000000000, 95.31249999726880162, -2.071067811865479058 ) ) ;
#17857=CARTESIAN_POINT ( 'NONE',  ( 97.50236033167492167, 117.6869444889999841, -51.77500000273119696 ) ) ;
#17858=VECTOR ( 'NONE', #697, 1000.000000000000000 ) ;
#17881=ORIENTED_EDGE ( 'NONE', *, *, #21122, .T. ) ;
#17885=FACE_OUTER_BOUND ( 'NONE', #15520, .T. ) ;
#17887=CARTESIAN_POINT ( 'NONE',  ( 108.0825317500000153, 110.0000000000000000, -52.12500000273119838 ) ) ;
#17893=ORIENTED_EDGE ( 'NONE', *, *, #6379, .T. ) ;
#17894=CARTESIAN_POINT ( 'NONE',  ( 99.14382582708707048, 122.8000000010924708, -2.066987299999999195 ) ) ;
#17898=DIRECTION ( 'NONE',  ( 0.000000000000000000, -0.000000000000000000, 1.000000000000000000 ) ) ;
#17899=DIRECTION ( 'NONE',  ( 0.8660254037844418162, -0.4999999999999947264, 0.000000000000000000 ) ) ;
#17907=ORIENTED_EDGE ( 'NONE', *, *, #11234, .T. ) ;
#17925=CARTESIAN_POINT ( 'NONE',  ( 99.99999999999998579, 94.62499999726881583, 4.999999999999984013 ) ) ;
#17935=CARTESIAN_POINT ( 'NONE',  ( 102.1631189606246295, 116.6573956140660897, -45.10000000546238397 ) ) ;
#17937=CARTESIAN_POINT ( 'NONE',  ( 95.00000000000000000, 90.56249999999998579, 2.071067811865463959 ) ) ;
#17938=CARTESIAN_POINT ( 'NONE',  ( 97.83149761400481736, 122.9999999999999716, 1.253061062422446970 ) ) ;
#17940=CARTESIAN_POINT ( 'NONE',  ( 101.4615807364564546, 124.0500000010924850, 1.461580736456455476 ) ) ;
#17947=CARTESIAN_POINT ( 'NONE',  ( 96.46446609406726225, 93.37500000000000000, -3.535533905932738197 ) ) ;
#17948=CARTESIAN_POINT ( 'NONE',  ( 99.99999999999998579, 95.31249999863440792, 4.458734124999981674 ) ) ;
#17949=AXIS2_PLACEMENT_3D ( 'NONE', #24257, #9147, #8581 ) ;
#17953=CARTESIAN_POINT ( 'NONE',  ( 96.46446609406726225, 95.49999999726881583, 3.535533905932723986 ) ) ;
#17965=CARTESIAN_POINT ( 'NONE',  ( 100.0000000000000000, 110.0000000000000000, -55.00000000000000711 ) ) ;
#17967=CARTESIAN_POINT ( 'NONE',  ( 99.99999999999998579, 92.25000000000000000, -4.999999999999997335 ) ) ;
#17971=AXIS2_PLACEMENT_3D ( 'NONE', #15769, #9500, #22344 ) ;
#17973=CARTESIAN_POINT ( 'NONE',  ( 108.0825317500000153, 110.0000000000000000, -46.12500000273119838 ) ) ;
#17974=CARTESIAN_POINT ( 'NONE',  ( 103.1528011352953484, 91.68749999863440792, -3.152801135295366208 ) ) ;
#17980=CARTESIAN_POINT ( 'NONE',  ( 95.00000000000000000, 91.43750000000000000, -2.071067811865479058 ) ) ;
#17986=CARTESIAN_POINT ( 'NONE',  ( 91.91746824999998466, 112.6261737610028320, -53.47500000273119980 ) ) ;
#17993=CARTESIAN_POINT ( 'NONE',  ( 97.92893218813452449, 95.18749999726880162, -4.999999999999997335 ) ) ;
#17998=CARTESIAN_POINT ( 'NONE',  ( 104.9952793366501709, 103.1245878333314465, -52.67500000273119554 ) ) ;
#18000=EDGE_CURVE ( 'NONE', #6173, #7474, #95, .T. ) ;
#18005=DIRECTION ( 'NONE',  ( -1.000000000000000000, 0.000000000000000000, 0.000000000000000000 ) ) ;
#18015=ORIENTED_EDGE ( 'NONE', *, *, #9550, .F. ) ;
#18022=CARTESIAN_POINT ( 'NONE',  ( 97.50236033167492167, 117.6869444889999841, -47.52500000273119696 ) ) ;
#18024=ADVANCED_FACE ( 'NONE', ( #17330 ), #26167, .T. ) ;
#18038=CARTESIAN_POINT ( 'NONE',  ( 99.99999999999998579, 93.06249999863440792, 4.458734124999981674 ) ) ;
#18042=CARTESIAN_POINT ( 'NONE',  ( 112.9999999999999858, 123.0000000000000000, 12.99999999999998934 ) ) ;
#18055=CARTESIAN_POINT ( 'NONE',  ( 102.4999999999999858, 123.9500000021849502, -1.035533905932742638 ) ) ;
#18056=AXIS2_PLACEMENT_3D ( 'NONE', #20152, #26714, #22858 ) ;
#18065=DIRECTION ( 'NONE',  ( 0.000000000000000000, -0.000000000000000000, 1.000000000000000000 ) ) ;
#18067=CARTESIAN_POINT ( 'NONE',  ( 97.83688103937538472, 116.6573956140660897, -54.40000000000000568 ) ) ;
#18068=AXIS2_PLACEMENT_3D ( 'NONE', #16742, #16878, #27447 ) ;
#18077=CARTESIAN_POINT ( 'NONE',  ( 108.0825317500000153, 110.0000000000000000, -52.37500000273119838 ) ) ;
#18078=CARTESIAN_POINT ( 'NONE',  ( 98.35030804145870320, 123.0000000000000284, -1.884035693330653904 ) ) ;
#18080=CARTESIAN_POINT ( 'NONE',  ( 97.93301270000000613, 123.7500000010924879, -9.540979117872439019E-15 ) ) ;
#18087=CARTESIAN_POINT ( 'NONE',  ( 104.9999999999999858, 91.00000000000000000, -6.938893903907228378E-15 ) ) ;
#18088=LINE ( 'NONE', #3276, #15607 ) ;
#18097=VERTEX_POINT ( 'NONE', #18181 ) ;
#18102=PRODUCT_DEFINITION_SHAPE ( 'NONE', 'NONE',  #13233 ) ;
#18106=FACE_BOUND ( 'NONE', #9989, .T. ) ;
#18107=CARTESIAN_POINT ( 'NONE',  ( 104.4587341249999781, 92.31249999863440792, -6.938893903907228378E-15 ) ) ;
#18114=CARTESIAN_POINT ( 'NONE',  ( 93.00000000000001421, 107.7255621263696668, -52.40000000546238823 ) ) ;
#18126=EDGE_LOOP ( 'NONE', ( #3167, #8138, #823 ) ) ;
#18130=CARTESIAN_POINT ( 'NONE',  ( 99.99999999999998579, 101.5015231886685854, -50.87500000273119127 ) ) ;
#18132=CARTESIAN_POINT ( 'NONE',  ( 101.7677669529663547, 124.7000000000000028, -1.767766952966370209 ) ) ;
#18139=CARTESIAN_POINT ( 'NONE',  ( 104.9999999999999858, 95.87499999726881583, -6.938893903907228378E-15 ) ) ;
#18141=CARTESIAN_POINT ( 'NONE',  ( 91.91746824999998466, 107.3738262389971680, -53.27500000273119696 ) ) ;
#18148=CARTESIAN_POINT ( 'NONE',  ( 93.00000000000000000, 110.0000000000000000, -55.00000000000000711 ) ) ;
#18153=CARTESIAN_POINT ( 'NONE',  ( 99.99999999999998579, 92.31249999863440792, 4.458734124999981674 ) ) ;
#18169=CARTESIAN_POINT ( 'NONE',  ( 99.99999999999998579, 90.00000000000000000, -4.999999999999996447 ) ) ;
#18171=CARTESIAN_POINT ( 'NONE',  ( 91.91746824999998466, 107.3738262389971680, -45.02500000273118985 ) ) ;
#18181=CARTESIAN_POINT ( 'NONE',  ( 87.00000000000000000, 97.00000000000000000, 12.99999999999999467 ) ) ;
#18183=CARTESIAN_POINT ( 'NONE',  ( 99.99999999999998579, 94.62499999726881583, 4.999999999999984013 ) ) ;
#18184=CARTESIAN_POINT ( 'NONE',  ( 102.0710678118655181, 95.68749999726881583, 4.999999999999919176 ) ) ;
#18185=EDGE_CURVE ( 'NONE', #370, #9199, #11747, .T. ) ;
#18186=CARTESIAN_POINT ( 'NONE',  ( 106.5389055433251002, 105.2492070361643215, -46.32500000273119412 ) ) ;
#18210=CARTESIAN_POINT ( 'NONE',  ( 97.50000000000000000, 125.0162387953032663, 0.1913417161825344548 ) ) ;
#18218=( BOUNDED_CURVE ( )  B_SPLINE_CURVE ( 2, ( #2558, #19648, #17796, #130, #17935, #17505, #26206 ),
 .UNSPECIFIED., .F., .T. ) 
 B_SPLINE_CURVE_WITH_KNOTS ( ( 3, 2, 2, 3 ),
 ( 0.8000000000000000444, 0.8199999999999999512, 0.8399999999999999689, 0.8500000005328695041 ),
 .UNSPECIFIED. ) 
 CURVE ( )  GEOMETRIC_REPRESENTATION_ITEM ( )  RATIONAL_B_SPLINE_CURVE ( ( 1.000000000000000000, 0.9510565162951535312, 1.000000000000000000, 0.9510565162951535312, 1.000000000000000000, 0.9755282568435521551, 0.9755282581475768211 ) ) 
 REPRESENTATION_ITEM ( '' )  );
#18228=CARTESIAN_POINT ( 'NONE',  ( 102.0244715095044512, 123.0000000000000000, -1.474530169995667883 ) ) ;
#18232=ORIENTED_EDGE ( 'NONE', *, *, #8133, .F. ) ;
#18237=CARTESIAN_POINT ( 'NONE',  ( 96.46446609406726225, 93.62500000000000000, 3.535533905932723986 ) ) ;
#18255=CARTESIAN_POINT ( 'NONE',  ( 93.00000000000001421, 107.7255621263696668, -50.40000000546238113 ) ) ;
#18256=CARTESIAN_POINT ( 'NONE',  ( 103.1528011352953484, 90.43749999863440792, -3.152801135295366208 ) ) ;
#18261=CARTESIAN_POINT ( 'NONE',  ( 105.6631189606246295, 114.1144967660473242, -53.30000000546237970 ) ) ;
#18262=CIRCLE ( 'NONE', #26916, 4.999999999999989342 ) ;
#18264=CARTESIAN_POINT ( 'NONE',  ( 95.00472066334982912, 116.8754121666685393, -45.42500000273119554 ) ) ;
#18265=CARTESIAN_POINT ( 'NONE',  ( 98.15313185440925281, 92.24999999863439371, 4.458734124999979898 ) ) ;
#18274=EDGE_CURVE ( 'NONE', #19519, #8183, #17163, .T. ) ;
#18280=CARTESIAN_POINT ( 'NONE',  ( 102.1631189606246295, 103.3426043859339103, -45.40000000000001279 ) ) ;
#18282=CARTESIAN_POINT ( 'NONE',  ( 101.7677669529663547, 124.5000000000000000, 1.767766952966350891 ) ) ;
#18287=CARTESIAN_POINT ( 'NONE',  ( 95.54126587499999346, 90.99999999863439371, -1.846868145590737864 ) ) ;
#18289=CARTESIAN_POINT ( 'NONE',  ( 93.46109445667491400, 105.2492070361643215, -51.17500000273119554 ) ) ;
#18299=CARTESIAN_POINT ( 'NONE',  ( 96.84719886470463734, 90.93749999863440792, -3.152801135295366208 ) ) ;
#18302=ORIENTED_EDGE ( 'NONE', *, *, #7618, .T. ) ;
#18309=CARTESIAN_POINT ( 'NONE',  ( 100.8561741729129295, 122.9000000010924794, -2.066987299999998751 ) ) ;
#18316=CARTESIAN_POINT ( 'NONE',  ( 106.5389055433251002, 114.7507929638356785, -45.92500000273119554 ) ) ;
#18318=LINE ( 'NONE', #27026, #3246 ) ;
#18320=EDGE_LOOP ( 'NONE', ( #24399, #7992, #11813, #21727 ) ) ;
#18321=EDGE_CURVE ( 'NONE', #28194, #4535, #1542, .T. ) ;
#18323=FILL_AREA_STYLE_COLOUR ( '', #4528 ) ;
#18332=CARTESIAN_POINT ( 'NONE',  ( 102.4976396683250925, 102.3130555110000159, -48.52500000273119696 ) ) ;
#18353=CARTESIAN_POINT ( 'NONE',  ( 98.23223304703363112, 124.9069999999781402, -1.767766952966370209 ) ) ;
#18357=CYLINDRICAL_SURFACE ( 'NONE', #24704, 2.499999999999995115 ) ;
#18369=CARTESIAN_POINT ( 'NONE',  ( 95.00472066334982912, 116.8754121666685393, -53.67500000273118843 ) ) ;
#18375=ORIENTED_EDGE ( 'NONE', *, *, #5863, .F. ) ;
#18379=CARTESIAN_POINT ( 'NONE',  ( 95.00000000000000000, 90.43750000000000000, -2.071067811865479058 ) ) ;
#18381=EDGE_CURVE ( 'NONE', #22191, #14907, #21014, .T. ) ;
#18382=VECTOR ( 'NONE', #16204, 1000.000000000000000 ) ;
#18405=CARTESIAN_POINT ( 'NONE',  ( 104.3262379212492590, 115.9545556584642867, -51.20000000546237828 ) ) ;
#18406=CYLINDRICAL_SURFACE ( 'NONE', #23197, 7.000000000000006217 ) ;
#18410=ADVANCED_FACE ( 'NONE', ( #20010 ), #22147, .T. ) ;
#18420=EDGE_LOOP ( 'NONE', ( #5167, #6714, #2495, #7427 ) ) ;
#18421=CARTESIAN_POINT ( 'NONE',  ( 91.91746824999998466, 112.6261737610028320, -49.47500000273119269 ) ) ;
#18428=AXIS2_PLACEMENT_3D ( 'NONE', #14009, #7752, #27160 ) ;
#18429=CARTESIAN_POINT ( 'NONE',  ( 96.84719886470463734, 93.93749999863440792, -3.152801135295366208 ) ) ;
#18430=DIRECTION ( 'NONE',  ( 0.000000000000000000, 4.625929269271485914E-16, 1.000000000000000000 ) ) ;
#18431=CARTESIAN_POINT ( 'NONE',  ( 93.46109445667491400, 114.7507929638356785, -53.57500000273119412 ) ) ;
#18441=DIRECTION ( 'NONE',  ( 0.000000000000000000, 1.000000000000000000, -1.156482317317871478E-16 ) ) ;
#18443=EDGE_LOOP ( 'NONE', ( #3587, #5028, #9334, #13865 ) ) ;
#18446=CARTESIAN_POINT ( 'NONE',  ( 95.54126587499999346, 93.12499999863439371, 1.846868145590722543 ) ) ;
#18466=VERTEX_POINT ( 'NONE', #19271 ) ;
#18467=ORIENTED_EDGE ( 'NONE', *, *, #7618, .F. ) ;
#18475=CARTESIAN_POINT ( 'NONE',  ( 108.0825317500000011, 112.6261737610028320, -48.02500000273118985 ) ) ;
#18477=AXIS2_PLACEMENT_3D ( 'NONE', #20555, #9844, #9707 ) ;
#18480=CARTESIAN_POINT ( 'NONE',  ( 96.46446609406726225, 91.24999999726880162, -3.535533905932738197 ) ) ;
#18494=DIRECTION ( 'NONE',  ( -1.000000000000000000, 0.000000000000000000, 0.000000000000000000 ) ) ;
#18501=DIRECTION ( 'NONE',  ( -0.000000000000000000, 1.000000000000000000, -0.000000000000000000 ) ) ;
#18509=LINE ( 'NONE', #20083, #2660 ) ;
#18511=DIRECTION ( 'NONE',  ( 5.782411586589357392E-17, 0.000000000000000000, 1.000000000000000000 ) ) ;
#18513=VECTOR ( 'NONE', #628, 1000.000000000000000 ) ;
#18524=CARTESIAN_POINT ( 'NONE',  ( 103.5355339059327235, 90.87500000000000000, 3.535533905932724874 ) ) ;
#18534=AXIS2_PLACEMENT_3D ( 'NONE', #25673, #12824, #12541 ) ;
#18547=CARTESIAN_POINT ( 'NONE',  ( 95.67376207875072680, 115.9545556584642867, -46.80000000546237970 ) ) ;
#18548=CARTESIAN_POINT ( 'NONE',  ( 101.8468681455907330, 94.37499999863440792, 4.458734124999979898 ) ) ;
#18552=ORIENTED_EDGE ( 'NONE', *, *, #5869, .F. ) ;
#18560=EDGE_CURVE ( 'NONE', #7349, #9247, #8712, .T. ) ;
#18564=ORIENTED_EDGE ( 'NONE', *, *, #16100, .F. ) ;
#18565=CARTESIAN_POINT ( 'NONE',  ( 102.4976396683250925, 102.3130555110000159, -46.77500000273119696 ) ) ;
#18572=CARTESIAN_POINT ( 'NONE',  ( 104.4587341249999923, 91.49999999863440792, 1.846868145590726318 ) ) ;
#18573=DIRECTION ( 'NONE',  ( 1.000000000000000000, -0.000000000000000000, -5.782411586589357392E-17 ) ) ;
#18583=CARTESIAN_POINT ( 'NONE',  ( 103.1528011352953484, 92.68749999863440792, -3.152801135295366208 ) ) ;
#18587=CARTESIAN_POINT ( 'NONE',  ( 95.00000000000000000, 93.56250000000000000, 2.071067811865463959 ) ) ;
#18592=DIRECTION ( 'NONE',  ( -0.000000000000000000, 1.000000000000000000, -0.000000000000000000 ) ) ;
#18609=CARTESIAN_POINT ( 'NONE',  ( 103.5355339059327235, 90.87500000000000000, 3.535533905932724874 ) ) ;
#18617=CARTESIAN_POINT ( 'NONE',  ( 104.9999999999999716, 93.81249999726880162, 2.071067811865467956 ) ) ;
#18632=CARTESIAN_POINT ( 'NONE',  ( 105.6631189606246295, 114.1144967660473242, -48.80000000000001137 ) ) ;
#18636=CARTESIAN_POINT ( 'NONE',  ( 97.50000000000000000, 124.2000000000000028, -9.540979117872439019E-15 ) ) ;
#18637=CARTESIAN_POINT ( 'NONE',  ( 102.4999999999999858, 122.9906688167216373, 0.1932551333443592867 ) ) ;
#18643=EDGE_LOOP ( 'NONE', ( #26442, #27141 ) ) ;
#18652=CARTESIAN_POINT ( 'NONE',  ( 99.99999999999998579, 118.4984768113314004, -45.87500000273118417 ) ) ;
#18655=CARTESIAN_POINT ( 'NONE',  ( 102.0669872999999797, 124.3500000010924822, -9.794112055954760458E-15 ) ) ;
#18674=CARTESIAN_POINT ( 'NONE',  ( 107.5412658750000077, 110.0000000000000000, -53.81250000409679046 ) ) ;
#18679=CARTESIAN_POINT ( 'NONE',  ( 98.15313185440923860, 93.99999999863439371, 4.458734124999980786 ) ) ;
#18682=DIRECTION ( 'NONE',  ( -1.000000000000000000, 0.000000000000000000, 0.000000000000000000 ) ) ;
#18684=ADVANCED_FACE ( 'NONE', ( #314 ), #20121, .F. ) ;
#18686=CARTESIAN_POINT ( 'NONE',  ( 94.33688103937537051, 105.8855032339526758, -48.30000000546237970 ) ) ;
#18687=CARTESIAN_POINT ( 'NONE',  ( 98.15313185440925281, 92.87499999863440792, -4.458734124999994997 ) ) ;
#18689=CARTESIAN_POINT ( 'NONE',  ( 102.4999999999999858, 122.9375000002731184, -9.847140817659276890E-15 ) ) ;
#18693=CARTESIAN_POINT ( 'NONE',  ( 95.54126587499999346, 90.87499999863439371, 1.846868145590722543 ) ) ;
#18698=ORIENTED_EDGE ( 'NONE', *, *, #19400, .F. ) ;
#18699=CARTESIAN_POINT ( 'NONE',  ( 91.91746824999998466, 107.3738262389971538, -47.27500000273118275 ) ) ;
#18705=CARTESIAN_POINT ( 'NONE',  ( 98.15313185440925281, 92.24999999863439371, 4.458734124999979898 ) ) ;
#18710=( BOUNDED_CURVE ( )  B_SPLINE_CURVE ( 2, ( #2453, #6568, #23826, #26248, #23968, #22117, #13100, #21696, #2597 ),
 .UNSPECIFIED., .F., .T. ) 
 B_SPLINE_CURVE_WITH_KNOTS ( ( 3, 2, 2, 2, 3 ),
 ( 0.4166666666666667407, 0.4583333333333334259, 0.5000000000000002220, 0.5416666666666668517, 0.5833333333333337034 ),
 .UNSPECIFIED. ) 
 CURVE ( )  GEOMETRIC_REPRESENTATION_ITEM ( )  RATIONAL_B_SPLINE_CURVE ( ( 0.9999999999999998890, 0.9238795325112868495, 1.000000000000000000, 0.9238795325112867385, 1.000000000000000000, 0.9238795325112867385, 1.000000000000000000, 0.9238795325112861834, 1.000000000000000666 ) ) 
 REPRESENTATION_ITEM ( '' )  );
#18718=EDGE_CURVE ( 'NONE', #20101, #923, #19377, .T. ) ;
#18721=CARTESIAN_POINT ( 'NONE',  ( 103.1528011352953484, 93.43749999863440792, 3.152801135295352886 ) ) ;
#18731=ORIENTED_EDGE ( 'NONE', *, *, #28113, .T. ) ;
#18732=DIRECTION ( 'NONE',  ( -2.674902700537828060E-32, 1.000000000000000000, -4.625929269271485914E-16 ) ) ;
#18733=CYLINDRICAL_SURFACE ( 'NONE', #15394, 7.000000000000006217 ) ;
#18736=CYLINDRICAL_SURFACE ( 'NONE', #12831, 4.999999999999989342 ) ;
#18741=ORIENTED_EDGE ( 'NONE', *, *, #27102, .F. ) ;
#18755=EDGE_CURVE ( 'NONE', #13582, #7547, #6993, .T. ) ;
#18771=CARTESIAN_POINT ( 'NONE',  ( 101.7677669529663547, 123.7069999999781515, 1.767766952966350891 ) ) ;
#18776=CARTESIAN_POINT ( 'NONE',  ( 99.99999999999998579, 102.6397644303321215, -48.00000000546237544 ) ) ;
#18785=CARTESIAN_POINT ( 'NONE',  ( 102.4976396683250925, 117.6869444889999841, -49.97500000273119269 ) ) ;
#18787=CARTESIAN_POINT ( 'NONE',  ( 98.53841926354351699, 124.6500000010924651, -1.461580736456474794 ) ) ;
#18788=DIRECTION ( 'NONE',  ( -0.000000000000000000, 1.000000000000000000, -0.000000000000000000 ) ) ;
#18799=ORIENTED_EDGE ( 'NONE', *, *, #18274, .T. ) ;
#18800=AXIS2_PLACEMENT_3D ( 'NONE', #13997, #13570, #18005 ) ;
#18810=CARTESIAN_POINT ( 'NONE',  ( 96.84719886470463734, 92.93749999863440792, 3.152801135295351997 ) ) ;
#18818=CARTESIAN_POINT ( 'NONE',  ( 93.00000000000001421, 112.2744378736303332, -50.60000000546236976 ) ) ;
#18819=CARTESIAN_POINT ( 'NONE',  ( 96.84719886470463734, 95.18749999863440792, 3.152801135295351997 ) ) ;
#18826=ORIENTED_EDGE ( 'NONE', *, *, #13303, .F. ) ;
#18827=ORIENTED_EDGE ( 'NONE', *, *, #8942, .T. ) ;
#18836=CARTESIAN_POINT ( 'NONE',  ( 93.46109445667491400, 105.2492070361643215, -50.92500000273119554 ) ) ;
#18842=PLANE ( 'NONE',  #23508 ) ;
#18852=CARTESIAN_POINT ( 'NONE',  ( 104.4587341249999781, 95.56249999863440792, -6.938893903907228378E-15 ) ) ;
#18876=DIRECTION ( 'NONE',  ( 0.000000000000000000, -1.000000000000000000, 0.000000000000000000 ) ) ;
#18877=CARTESIAN_POINT ( 'NONE',  ( 99.99999999999998579, 94.25000000000000000, -4.999999999999997335 ) ) ;
#18895=CARTESIAN_POINT ( 'NONE',  ( 107.0000000000000142, 112.2744378736303048, -48.89999999999999858 ) ) ;
#18901=CARTESIAN_POINT ( 'NONE',  ( 102.4999999999999858, 124.6000000000000085, -9.847140817659276890E-15 ) ) ;
#18904=CARTESIAN_POINT ( 'NONE',  ( 100.8561741729129295, 124.5000000010924737, -2.066987299999998751 ) ) ;
#18918=CARTESIAN_POINT ( 'NONE',  ( 104.9952793366501851, 103.1245878333314323, -48.67500000273119554 ) ) ;
#18919=CARTESIAN_POINT ( 'NONE',  ( 99.99999999999998579, 89.99899999999999523, -9.540979117872439019E-15 ) ) ;
#18920=CARTESIAN_POINT ( 'NONE',  ( 97.93301269999999192, 124.0000000010924879, 0.8561741729129329626 ) ) ;
#18925=CARTESIAN_POINT ( 'NONE',  ( 93.00000000000000000, 110.0000000000000000, -50.00000000000000711 ) ) ;
#18951=CARTESIAN_POINT ( 'NONE',  ( 97.83688103937537051, 103.3426043859339103, -52.10000000546238397 ) ) ;
#18952=CARTESIAN_POINT ( 'NONE',  ( 95.54126587499999346, 90.87499999863439371, 1.846868145590722543 ) ) ;
#18953=AXIS2_PLACEMENT_3D ( 'NONE', #25044, #18494, #14472 ) ;
#18957=EDGE_LOOP ( 'NONE', ( #2120, #12171, #18375, #24928 ) ) ;
#18963=ORIENTED_EDGE ( 'NONE', *, *, #10525, .F. ) ;
#18968=CARTESIAN_POINT ( 'NONE',  ( 102.4976396683250925, 117.6869444889999841, -49.97500000273119269 ) ) ;
#18972=CARTESIAN_POINT ( 'NONE',  ( 106.5389055433251002, 105.2492070361643215, -48.32500000273119412 ) ) ;
#18973=CARTESIAN_POINT ( 'NONE',  ( 94.33688103937537051, 105.8855032339526758, -51.80000000000000426 ) ) ;
#18976=ORIENTED_EDGE ( 'NONE', *, *, #24484, .F. ) ;
#18978=CYLINDRICAL_SURFACE ( 'NONE', #19103, 7.000000000000006217 ) ;
#18990=CARTESIAN_POINT ( 'NONE',  ( 97.93301270000000613, 123.7000000010924765, -0.8561741729129506151 ) ) ;
#18991=CARTESIAN_POINT ( 'NONE',  ( 101.8468681455907330, 93.37499999863440792, 4.458734124999980786 ) ) ;
#19000=CARTESIAN_POINT ( 'NONE',  ( 96.46446609406726225, 92.62500000000000000, 3.535533905932723986 ) ) ;
#19002=VECTOR ( 'NONE', #6486, 1000.000000000000000 ) ;
#19005=CARTESIAN_POINT ( 'NONE',  ( 114.9999999999999858, 120.0000000000000000, -15.00000000000000711 ) ) ;
#19010=CARTESIAN_POINT ( 'NONE',  ( 104.9999999999999716, 91.06250000000000000, -2.071067811865478170 ) ) ;
#19013=CARTESIAN_POINT ( 'NONE',  ( 102.4364866161514556, 122.9999999999999574, 0.6508234534886077061 ) ) ;
#19015=FACE_BOUND ( 'NONE', #13663, .T. ) ;
#19030=( BOUNDED_SURFACE ( )  B_SPLINE_SURFACE ( 1, 2, ( 
 ( #5489, #14158, #16587, #12150, #27430, #27571, #20875, #1360, #8031, #16729, #23293, #2046, #15122, #17561, #28124, #8448, #17278, #21715, #19289, #4463, #21991, #14846, #26265, #23985, #25695, #10850, #13119, #2189, #2468, #8728, #10715, #4047, #6178, #23567, #8589, #10989, #19423, #19563, #1914, #19145, #12844, #12710, #21434, #25980, #23844, #6725, #6451, #17137, #4320, #46, #27987, #21856, #27850, #12979, #6313, #8869, #10579, #25838, #17420, #14989, #15411, #26119, #2331, #6584, #15266, #19701, #187, #24127, #4599, #13259, #8306, #16996, #23706, #4182, #21572, #11273, #15701, #24549, #9431, #24264, #473, #6869, #5172, #24694, #614, #9290, #26551, #22704, #22132, #2611, #13554, #22560, #26986, #11416, #5315, #7146, #18280, #9576, #24403, #22415, #19993 ),
 ( #2753, #9155, #20135, #11696, #13835, #17848, #22278, #3027, #7431, #17986, #15980, #26696, #20421, #15840, #7006, #20271, #5032, #16126, #13698, #4891, #24832, #2884, #905, #13976, #13405, #11129, #19843, #330, #9016, #11555, #17708, #26411, #757, #15555, #4746, #18130, #26842, #7291, #25248, #11984, #6009, #11844, #8139, #10258, #18968, #9719, #5738, #25529, #27539, #18421, #16695, #14673, #1323, #10119, #7863, #22985, #20708, #3452, #3734, #25394, #1190, #14265, #14545, #27675, #12118, #7996, #20845, #5875, #9990, #9858, #12255, #18699, #16833, #27402, #7723, #3172, #18565, #23260, #20567, #5455, #21115, #12394, #1602, #1047, #27267, #27128, #7579, #16557, #16273, #24971, #16415, #14405, #23122, #3597, #25112, #14125, #22846, #3313, #5599, #20982, #1462 ) ),
 .UNSPECIFIED., .F., .F., .F. ) 
 B_SPLINE_SURFACE_WITH_KNOTS ( ( 2, 2 ),
 ( 3, 2, 2, 2, 2, 2, 2, 2, 2, 2, 2, 2, 2, 2, 2, 2, 2, 2, 2, 2, 2, 2, 2, 2, 2, 2, 2, 2, 2, 2, 2, 2, 2, 2, 2, 2, 2, 2, 2, 2, 2, 2, 2, 2, 2, 2, 2, 2, 2, 2, 3 ),
 ( 0.000000000000000000, 1.000000000000000000 ),
 ( 0.000000000000000000, 0.02000000000000000042, 0.04000000000000000083, 0.05999999999999999778, 0.08000000000000000167, 0.1000000000000000056, 0.1199999999999999956, 0.1400000000000000133, 0.1600000000000000033, 0.1799999999999999933, 0.2000000000000000111, 0.2200000000000000011, 0.2399999999999999911, 0.2600000000000000089, 0.2800000000000000266, 0.2999999999999999889, 0.3200000000000000067, 0.3400000000000000244, 0.3599999999999999867, 0.3800000000000000044, 0.4000000000000000222, 0.4199999999999999845, 0.4400000000000000022, 0.4600000000000000200, 0.4799999999999999822, 0.5000000000000000000, 0.5200000000000000178, 0.5400000000000000355, 0.5600000000000000533, 0.5799999999999999600, 0.5999999999999999778, 0.6199999999999999956, 0.6400000000000000133, 0.6600000000000000311, 0.6800000000000000488, 0.6999999999999999556, 0.7199999999999999734, 0.7399999999999999911, 0.7600000000000000089, 0.7800000000000000266, 0.8000000000000000444, 0.8199999999999999512, 0.8399999999999999689, 0.8599999999999999867, 0.8800000000000000044, 0.9000000000000000222, 0.9200000000000000400, 0.9399999999999999467, 0.9599999999999999645, 0.9799999999999999822, 1.000000000000000000 ),
 .UNSPECIFIED. ) 
 GEOMETRIC_REPRESENTATION_ITEM ( )  RATIONAL_B_SPLINE_SURFACE ( (
 ( 1.000000000000000000, 0.9510565162951535312, 1.000000000000000000, 0.9510565162951535312, 1.000000000000000000, 0.9510565162951535312, 1.000000000000000000, 0.9510565162951535312, 1.000000000000000000, 0.9510565162951535312, 1.000000000000000000, 0.9510565162951535312, 1.000000000000000000, 0.9510565162951535312, 1.000000000000000000, 0.9510565162951535312, 1.000000000000000000, 0.9510565162951535312, 1.000000000000000000, 0.9510565162951535312, 1.000000000000000000, 0.9510565162951535312, 1.000000000000000000, 0.9510565162951535312, 1.000000000000000000, 0.9510565162951535312, 1.000000000000000000, 0.9510565162951535312, 1.000000000000000000, 0.9510565162951535312, 1.000000000000000000, 0.9510565162951535312, 1.000000000000000000, 0.9510565162951535312, 1.000000000000000000, 0.9510565162951535312, 1.000000000000000000, 0.9510565162951535312, 1.000000000000000000, 0.9510565162951535312, 1.000000000000000000, 0.9510565162951535312, 1.000000000000000000, 0.9510565162951535312, 1.000000000000000000, 0.9510565162951535312, 1.000000000000000000, 0.9510565162951535312, 1.000000000000000000, 0.9510565162951535312, 1.000000000000000000, 0.9510565162951535312, 1.000000000000000000, 0.9510565162951535312, 1.000000000000000000, 0.9510565162951535312, 1.000000000000000000, 0.9510565162951535312, 1.000000000000000000, 0.9510565162951535312, 1.000000000000000000, 0.9510565162951535312, 1.000000000000000000, 0.9510565162951535312, 1.000000000000000000, 0.9510565162951535312, 1.000000000000000000, 0.9510565162951535312, 1.000000000000000000, 0.9510565162951535312, 1.000000000000000000, 0.9510565162951535312, 1.000000000000000000, 0.9510565162951535312, 1.000000000000000000, 0.9510565162951535312, 1.000000000000000000, 0.9510565162951535312, 1.000000000000000000, 0.9510565162951535312, 1.000000000000000000, 0.9510565162951535312, 1.000000000000000000, 0.9510565162951535312, 1.000000000000000000, 0.9510565162951535312, 1.000000000000000000, 0.9510565162951535312, 1.000000000000000000, 0.9510565162951535312, 1.000000000000000000, 0.9510565162951535312, 1.000000000000000000, 0.9510565162951535312, 1.000000000000000000, 0.9510565162951535312, 1.000000000000000000, 0.9510565162951535312, 1.000000000000000000, 0.9510565162951535312, 1.000000000000000000),
 ( 1.000000000000000000, 0.9510565162951535312, 1.000000000000000000, 0.9510565162951535312, 1.000000000000000000, 0.9510565162951535312, 1.000000000000000000, 0.9510565162951535312, 1.000000000000000000, 0.9510565162951535312, 1.000000000000000000, 0.9510565162951535312, 1.000000000000000000, 0.9510565162951535312, 1.000000000000000000, 0.9510565162951535312, 1.000000000000000000, 0.9510565162951535312, 1.000000000000000000, 0.9510565162951535312, 1.000000000000000000, 0.9510565162951535312, 1.000000000000000000, 0.9510565162951535312, 1.000000000000000000, 0.9510565162951535312, 1.000000000000000000, 0.9510565162951535312, 1.000000000000000000, 0.9510565162951535312, 1.000000000000000000, 0.9510565162951535312, 1.000000000000000000, 0.9510565162951535312, 1.000000000000000000, 0.9510565162951535312, 1.000000000000000000, 0.9510565162951535312, 1.000000000000000000, 0.9510565162951535312, 1.000000000000000000, 0.9510565162951535312, 1.000000000000000000, 0.9510565162951535312, 1.000000000000000000, 0.9510565162951535312, 1.000000000000000000, 0.9510565162951535312, 1.000000000000000000, 0.9510565162951535312, 1.000000000000000000, 0.9510565162951535312, 1.000000000000000000, 0.9510565162951535312, 1.000000000000000000, 0.9510565162951535312, 1.000000000000000000, 0.9510565162951535312, 1.000000000000000000, 0.9510565162951535312, 1.000000000000000000, 0.9510565162951535312, 1.000000000000000000, 0.9510565162951535312, 1.000000000000000000, 0.9510565162951535312, 1.000000000000000000, 0.9510565162951535312, 1.000000000000000000, 0.9510565162951535312, 1.000000000000000000, 0.9510565162951535312, 1.000000000000000000, 0.9510565162951535312, 1.000000000000000000, 0.9510565162951535312, 1.000000000000000000, 0.9510565162951535312, 1.000000000000000000, 0.9510565162951535312, 1.000000000000000000, 0.9510565162951535312, 1.000000000000000000, 0.9510565162951535312, 1.000000000000000000, 0.9510565162951535312, 1.000000000000000000, 0.9510565162951535312, 1.000000000000000000, 0.9510565162951535312, 1.000000000000000000, 0.9510565162951535312, 1.000000000000000000, 0.9510565162951535312, 1.000000000000000000, 0.9510565162951535312, 1.000000000000000000, 0.9510565162951535312, 1.000000000000000000, 0.9510565162951535312, 1.000000000000000000) ) ) 
 REPRESENTATION_ITEM ( '' )  SURFACE ( )  );
#19037=CARTESIAN_POINT ( 'NONE',  ( 98.23223304703363112, 124.1000000000000085, -1.767766952966370209 ) ) ;
#19040=CARTESIAN_POINT ( 'NONE',  ( 98.53841926354351699, 123.2500000010924737, 1.461580736456455920 ) ) ;
#19045=CARTESIAN_POINT ( 'NONE',  ( 99.99999999999998579, 125.0000000000000000, -9.540979117872439019E-15 ) ) ;
#19046=EDGE_LOOP ( 'NONE', ( #6450, #17907 ) ) ;
#19047=CARTESIAN_POINT ( 'NONE',  ( 99.99999999999998579, 123.7000000021849502, 2.499999999999978684 ) ) ;
#19054=CARTESIAN_POINT ( 'NONE',  ( 106.5389055433251002, 114.7507929638356785, -46.17500000273119554 ) ) ;
#19058=CARTESIAN_POINT ( 'NONE',  ( 102.0669872999999939, 123.5000000010924595, 0.8561741729129311862 ) ) ;
#19064=FACE_BOUND ( 'NONE', #14395, .T. ) ;
#19068=ADVANCED_FACE ( 'NONE', ( #9647, #2684 ), #5245, .F. ) ;
#19082=CARTESIAN_POINT ( 'NONE',  ( 96.84719886470463734, 93.68749999863440792, -3.152801135295366208 ) ) ;
#19091=CARTESIAN_POINT ( 'NONE',  ( 97.83688103937537051, 103.3426043859339103, -44.10000000546238397 ) ) ;
#19092=CARTESIAN_POINT ( 'NONE',  ( 101.8468681455907330, 91.12499999863439371, 4.458734124999979898 ) ) ;
#19100=CARTESIAN_POINT ( 'NONE',  ( 98.15313185440925281, 91.62499999863440792, -4.458734124999994997 ) ) ;
#19103=AXIS2_PLACEMENT_3D ( 'NONE', #20716, #23270, #6020 ) ;
#19106=ORIENTED_EDGE ( 'NONE', *, *, #606, .F. ) ;
#19120=VERTEX_POINT ( 'NONE', #2871 ) ;
#19122=LINE ( 'NONE', #23962, #17317 ) ;
#19140=ORIENTED_EDGE ( 'NONE', *, *, #2221, .F. ) ;
#19145=CARTESIAN_POINT ( 'NONE',  ( 107.0000000000000142, 107.7255621263696526, -51.10000000000000142 ) ) ;
#19147=CARTESIAN_POINT ( 'NONE',  ( 98.53841926354351699, 123.8500000010924680, -1.461580736456474794 ) ) ;
#19154=ORIENTED_EDGE ( 'NONE', *, *, #2547, .F. ) ;
#19155=ORIENTED_EDGE ( 'NONE', *, *, #17241, .T. ) ;
#19163=DIRECTION ( 'NONE',  ( 0.000000000000000000, 0.000000000000000000, -1.000000000000000000 ) ) ;
#19165=CARTESIAN_POINT ( 'NONE',  ( 99.99999999999998579, 93.62499999726881583, 4.999999999999984013 ) ) ;
#19183=CARTESIAN_POINT ( 'NONE',  ( 101.7677669529663547, 124.5000000000000000, 1.767766952966350891 ) ) ;
#19191=CARTESIAN_POINT ( 'NONE',  ( 98.23223304703363112, 124.2000000021849502, -1.767766952966370209 ) ) ;
#19198=CARTESIAN_POINT ( 'NONE',  ( 93.46109445667491400, 105.2492070361643215, -47.17500000273119554 ) ) ;
#19200=VERTEX_POINT ( 'NONE', #22836 ) ;
#19201=CARTESIAN_POINT ( 'NONE',  ( 98.53841926354351699, 124.0500000010924708, 1.461580736456455920 ) ) ;
#19205=VERTEX_POINT ( 'NONE', #9979 ) ;
#19215=CARTESIAN_POINT ( 'NONE',  ( 93.00000000000000000, 110.0000000000000000, -46.50000000546238255 ) ) ;
#19222=EDGE_CURVE ( 'NONE', #17238, #12623, #1178, .T. ) ;
#19224=CARTESIAN_POINT ( 'NONE',  ( 96.84719886470463734, 94.93749999863440792, 3.152801135295351997 ) ) ;
#19233=CARTESIAN_POINT ( 'NONE',  ( 105.6631189606246295, 105.8855032339526758, -45.70000000546237828 ) ) ;
#19234=CARTESIAN_POINT ( 'NONE',  ( 104.4587341249999923, 94.37499999863440792, -1.846868145590737198 ) ) ;
#19238=EDGE_CURVE ( 'NONE', #12415, #1189, #14344, .T. ) ;
#19239=ORIENTED_EDGE ( 'NONE', *, *, #19952, .T. ) ;
#19242=ORIENTED_EDGE ( 'NONE', *, *, #7041, .T. ) ;
#19246=ORIENTED_EDGE ( 'NONE', *, *, #3410, .F. ) ;
#19247=DIRECTION ( 'NONE',  ( -0.000000000000000000, 4.625929269271485914E-16, 1.000000000000000000 ) ) ;
#19253=EDGE_CURVE ( 'NONE', #24513, #17238, #724, .T. ) ;
#19260=EDGE_LOOP ( 'NONE', ( #7399, #8442, #24820, #21709 ) ) ;
#19269=CARTESIAN_POINT ( 'NONE',  ( 102.4976396683250925, 117.6869444889999841, -49.72500000273119269 ) ) ;
#19271=CARTESIAN_POINT ( 'NONE',  ( 99.99999999999998579, 123.2000000000000028, -2.499999999999997780 ) ) ;
#19278=CARTESIAN_POINT ( 'NONE',  ( 99.14382582708708469, 123.6000000010924680, -2.066987299999998751 ) ) ;
#19289=CARTESIAN_POINT ( 'NONE',  ( 105.6631189606246295, 105.8855032339526758, -53.20000000000000284 ) ) ;
#19309=ORIENTED_EDGE ( 'NONE', *, *, #24151, .T. ) ;
#19322=DIRECTION ( 'NONE',  ( -0.000000000000000000, 1.000000000000000000, -0.000000000000000000 ) ) ;
#19323=CARTESIAN_POINT ( 'NONE',  ( 102.4999999999999858, 122.2906688189065818, 0.1932551333443592867 ) ) ;
#19328=CARTESIAN_POINT ( 'NONE',  ( 105.6631189606246295, 105.8855032339526758, -53.20000000000000284 ) ) ;
#19336=CARTESIAN_POINT ( 'NONE',  ( 99.99999999999998579, 101.5015231886685854, -50.62500000273119838 ) ) ;
#19349=VECTOR ( 'NONE', #5111, 1000.000000000000000 ) ;
#19365=CARTESIAN_POINT ( 'NONE',  ( 97.50236033167492167, 117.6869444889999841, -47.77500000273119696 ) ) ;
#19370=CARTESIAN_POINT ( 'NONE',  ( 107.0000000000000142, 110.0000000000000000, -45.50000000546238255 ) ) ;
#19371=CARTESIAN_POINT ( 'NONE',  ( 101.8468681455907330, 93.12499999863439371, 4.458734124999979898 ) ) ;
#19375=ORIENTED_EDGE ( 'NONE', *, *, #20938, .F. ) ;
#19377=CIRCLE ( 'NONE', #11608, 4.999999999999989342 ) ;
#19378=CARTESIAN_POINT ( 'NONE',  ( 95.54126587499999346, 94.87499999863440792, 1.846868145590722543 ) ) ;
#19379=ORIENTED_EDGE ( 'NONE', *, *, #2921, .F. ) ;
#19391=CARTESIAN_POINT ( 'NONE',  ( 107.0000000000000284, 107.7255621263696810, -51.10000000000000142 ) ) ;
#19400=EDGE_CURVE ( 'NONE', #24826, #7547, #16683, .T. ) ;
#19402=CARTESIAN_POINT ( 'NONE',  ( 102.4976396683250925, 117.6869444889999841, -51.72500000273119980 ) ) ;
#19409=CARTESIAN_POINT ( 'NONE',  ( 99.99999999999998579, 117.3602355696678643, -51.00000000546237544 ) ) ;
#19410=CARTESIAN_POINT ( 'NONE',  ( 102.0669873000000081, 124.2000000010924623, -0.8561741729129508371 ) ) ;
#19414=EDGE_CURVE ( 'NONE', #5734, #20470, #1452, .T. ) ;
#19423=CARTESIAN_POINT ( 'NONE',  ( 102.1631189606246295, 103.3426043859339103, -51.40000000000000568 ) ) ;
#19425=CARTESIAN_POINT ( 'NONE',  ( 97.93301270000000613, 124.7500000010924737, -9.540979117872439019E-15 ) ) ;
#19426=EDGE_CURVE ( 'NONE', #210, #23799, #25458, .T. ) ;
#19442=CARTESIAN_POINT ( 'NONE',  ( 107.0000000000000142, 110.0000000000000000, -45.00000000000000711 ) ) ;
#19443=CARTESIAN_POINT ( 'NONE',  ( 101.7677669529663547, 123.0999999999999943, -1.767766952966370209 ) ) ;
#19457=CARTESIAN_POINT ( 'NONE',  ( 104.3262379212492590, 104.0454443415356991, -45.80000000546237970 ) ) ;
#19463=CARTESIAN_POINT ( 'NONE',  ( 104.9952793366501709, 116.8754121666685393, -51.82500000273120122 ) ) ;
#19466=CARTESIAN_POINT ( 'NONE',  ( 102.4999999999999716, 123.9500000021849502, -1.035533905932742638 ) ) ;
#19470=CARTESIAN_POINT ( 'NONE',  ( 93.00000000000000000, 110.0000000000000000, -54.00000000000000711 ) ) ;
#19477=CARTESIAN_POINT ( 'NONE',  ( 108.0825317500000153, 110.0000000000000000, -50.12500000273119127 ) ) ;
#19493=CIRCLE ( 'NONE', #5392, 7.000000000000006217 ) ;
#19500=CARTESIAN_POINT ( 'NONE',  ( 101.7677669209684552, 123.0000000000000000, 1.767766984964258992 ) ) ;
#19514=CARTESIAN_POINT ( 'NONE',  ( 103.1528011352953484, 93.18749999863440792, 3.152801135295352886 ) ) ;
#19515=CARTESIAN_POINT ( 'NONE',  ( 96.46446609406726225, 93.49999999726881583, 3.535533905932723986 ) ) ;
#19519=VERTEX_POINT ( 'NONE', #420 ) ;
#19522=CARTESIAN_POINT ( 'NONE',  ( 103.1528011352953484, 93.18749999863440792, 3.152801135295352886 ) ) ;
#19526=ORIENTED_EDGE ( 'NONE', *, *, #19426, .T. ) ;
#19527=DIRECTION ( 'NONE',  ( -0.000000000000000000, 1.000000000000000000, -0.000000000000000000 ) ) ;
#19539=EDGE_CURVE ( 'NONE', #210, #11286, #2562, .T. ) ;
#19547=CARTESIAN_POINT ( 'NONE',  ( 104.9952793366501851, 103.1245878333314323, -50.42500000273119554 ) ) ;
#19563=CARTESIAN_POINT ( 'NONE',  ( 104.3262379212492590, 104.0454443415356991, -51.29999999999999716 ) ) ;
#19565=CIRCLE ( 'NONE', #25033, 9.000000000000007105 ) ;
#19568=CARTESIAN_POINT ( 'NONE',  ( 95.00000000000000000, 94.37499999726881583, -7.551217303480904118E-15 ) ) ;
#19585=CARTESIAN_POINT ( 'NONE',  ( 105.6631189606246295, 105.8855032339526758, -49.20000000000000995 ) ) ;
#19595=CARTESIAN_POINT ( 'NONE',  ( 107.0000000000000142, 110.0000000000000000, -45.50000000546238255 ) ) ;
#19600=CARTESIAN_POINT ( 'NONE',  ( 104.9952793366501709, 103.1245878333314465, -52.42500000273119554 ) ) ;
#19604=DIRECTION ( 'NONE',  ( -5.782411586589357392E-17, 0.000000000000000000, -1.000000000000000000 ) ) ;
#19607=ORIENTED_EDGE ( 'NONE', *, *, #3410, .T. ) ;
#19608=CARTESIAN_POINT ( 'NONE',  ( 102.0669872999999939, 122.6000000010924964, -0.8561741729129507261 ) ) ;
#19613=DIRECTION ( 'NONE',  ( -1.000000000000000000, 0.000000000000000000, 5.782411586589357392E-17 ) ) ;
#19616=CARTESIAN_POINT ( 'NONE',  ( 97.50236033167492167, 102.3130555110000159, -52.72500000273119980 ) ) ;
#19620=DIRECTION ( 'NONE',  ( 0.8660254037844418162, 0.4999999999999947264, -0.000000000000000000 ) ) ;
#19625=CARTESIAN_POINT ( 'NONE',  ( 99.99999999999998579, 125.0000000000000000, -2.500000000000004885 ) ) ;
#19637=CARTESIAN_POINT ( 'NONE',  ( 102.0710678118654897, 92.81249999999998579, 4.999999999999953815 ) ) ;
#19638=CARTESIAN_POINT ( 'NONE',  ( 101.0355339059327235, 122.4500000021849502, -2.499999999999997780 ) ) ;
#19647=CARTESIAN_POINT ( 'NONE',  ( 95.00472066334981491, 103.1245878333314465, -45.07500000273119412 ) ) ;
#19648=CARTESIAN_POINT ( 'NONE',  ( 107.0000000000000142, 112.2744378736303190, -45.40000000546237402 ) ) ;
#19650=CARTESIAN_POINT ( 'NONE',  ( 99.99999999999998579, 90.00000000000000000, 4.999999999999983125 ) ) ;
#19651=CARTESIAN_POINT ( 'NONE',  ( 94.33688103937537051, 105.8855032339526758, -44.30000000546237970 ) ) ;
#19652=CARTESIAN_POINT ( 'NONE',  ( 95.54126587499999346, 94.74999999863440792, -1.846868145590737864 ) ) ;
#19656=EDGE_LOOP ( 'NONE', ( #15472, #22443, #23576 ) ) ;
#19657=ORIENTED_EDGE ( 'NONE', *, *, #19238, .F. ) ;
#19660=CARTESIAN_POINT ( 'NONE',  ( 104.4587341249999923, 92.37499999863440792, -1.846868145590737198 ) ) ;
#19666=CARTESIAN_POINT ( 'NONE',  ( 97.92893218813448186, 95.18749999726880162, -4.999999999999948486 ) ) ;
#19682=DIRECTION ( 'NONE',  ( 0.000000000000000000, -1.000000000000000000, 0.000000000000000000 ) ) ;
#19684=CARTESIAN_POINT ( 'NONE',  ( 97.50236033167492167, 117.6869444889999841, -51.52500000273119696 ) ) ;
#19692=LINE ( 'NONE', #179, #20730 ) ;
#19693=CARTESIAN_POINT ( 'NONE',  ( 99.99999999999998579, 90.00000000000000000, -6.938893903907228378E-15 ) ) ;
#19701=CARTESIAN_POINT ( 'NONE',  ( 99.99999999999998579, 117.3602355696678501, -48.50000000000000000 ) ) ;
#19704=CIRCLE ( 'NONE', #23360, 9.000000000000007105 ) ;
#19708=CARTESIAN_POINT ( 'NONE',  ( 104.9999999999999716, 91.81249999726880162, 2.071067811865467956 ) ) ;
#19732=ADVANCED_FACE ( 'NONE', ( #22366 ), #24373, .F. ) ;
#19739=CARTESIAN_POINT ( 'NONE',  ( 108.0825317500000153, 110.0000000000000000, -54.12500000273119838 ) ) ;
#19741=CARTESIAN_POINT ( 'NONE',  ( 99.99999999999998579, 95.00000000000000000, -6.938893903907228378E-15 ) ) ;
#19747=CARTESIAN_POINT ( 'NONE',  ( 97.93301269999999192, 123.0000000010925163, 0.8561741729129329626 ) ) ;
#19755=CARTESIAN_POINT ( 'NONE',  ( 108.0825317500000153, 110.0000000000000000, -54.12500000273119838 ) ) ;
#19769=ORIENTED_EDGE ( 'NONE', *, *, #7425, .F. ) ;
#19784=( BOUNDED_CURVE ( )  B_SPLINE_CURVE ( 2, ( #14217, #22654, #27218, #26936, #15927, #17937, #5552, #7380, #9527 ),
 .UNSPECIFIED., .F., .F. ) 
 B_SPLINE_CURVE_WITH_KNOTS ( ( 3, 2, 2, 2, 3 ),
 ( 0.05000000000000004441, 0.07500000000000006661, 0.1000000000000000888, 0.1250000000000001110, 0.1500000000000001332 ),
 .UNSPECIFIED. ) 
 CURVE ( )  GEOMETRIC_REPRESENTATION_ITEM ( )  RATIONAL_B_SPLINE_CURVE ( ( 0.9999999999999998890, 0.9238795325112868495, 1.000000000000000000, 0.9238795325112867385, 1.000000000000000000, 0.9238795325112867385, 1.000000000000000000, 0.9238795325112862944, 1.000000000000000444 ) ) 
 REPRESENTATION_ITEM ( '' )  );
#19793=CARTESIAN_POINT ( 'NONE',  ( 100.2089334463084072, 123.0000000000000142, -2.507929215363408293 ) ) ;
#19798=ORIENTED_EDGE ( 'NONE', *, *, #19414, .T. ) ;
#19802=CARTESIAN_POINT ( 'NONE',  ( 97.92893218813452449, 90.31250000000001421, -4.999999999999997335 ) ) ;
#19833=ORIENTED_EDGE ( 'NONE', *, *, #16267, .T. ) ;
#19834=CARTESIAN_POINT ( 'NONE',  ( 93.00000000000000000, 110.0000000000000000, -50.50000000546237544 ) ) ;
#19843=CARTESIAN_POINT ( 'NONE',  ( 97.50236033167492167, 117.6869444889999841, -51.77500000273119696 ) ) ;
#19846=CARTESIAN_POINT ( 'NONE',  ( 101.7677669529663547, 123.7000000000000028, 1.767766952966350891 ) ) ;
#19849=CARTESIAN_POINT ( 'NONE',  ( 95.00000000000000000, 94.43749999726878741, 2.071067811865463959 ) ) ;
#19855=ORIENTED_EDGE ( 'NONE', *, *, #1318, .F. ) ;
#19868=ORIENTED_EDGE ( 'NONE', *, *, #7208, .T. ) ;
#19884=CARTESIAN_POINT ( 'NONE',  ( 99.99999999999998579, 124.7999999999999972, -2.499999999999997780 ) ) ;
#19892=ORIENTED_EDGE ( 'NONE', *, *, #13459, .T. ) ;
#19893=CARTESIAN_POINT ( 'NONE',  ( 99.99999999999998579, 122.5000000021849615, -2.499999999999997780 ) ) ;
#19900=CARTESIAN_POINT ( 'NONE',  ( 106.5389055433251002, 114.7507929638356785, -53.92500000273119554 ) ) ;
#19902=ADVANCED_BREP_SHAPE_REPRESENTATION ( '', ( #17619, #26844 ), #4064 ) ;
#19903=AXIS2_PLACEMENT_3D ( 'NONE', #14884, #14473, #21468 ) ;
#19904=CARTESIAN_POINT ( 'NONE',  ( 114.9999999999999858, 120.0000000000000000, -15.00000000000000711 ) ) ;
#19940=CARTESIAN_POINT ( 'NONE',  ( 97.53586499902618812, 122.9999999999999716, 0.4483706153950356987 ) ) ;
#19945=VERTEX_POINT ( 'NONE', #6641 ) ;
#19949=CARTESIAN_POINT ( 'NONE',  ( 104.4587341249999781, 92.31249999863440792, -6.938893903907228378E-15 ) ) ;
#19952=EDGE_CURVE ( 'NONE', #25694, #17550, #11048, .T. ) ;
#19959=ORIENTED_EDGE ( 'NONE', *, *, #17331, .F. ) ;
#19965=EDGE_CURVE ( 'NONE', #11839, #8168, #11185, .T. ) ;
#19976=CARTESIAN_POINT ( 'NONE',  ( 102.4976396683250925, 117.6869444889999841, -47.72500000273119269 ) ) ;
#19986=CARTESIAN_POINT ( 'NONE',  ( 102.0669873000000081, 122.6000000010924822, -0.8561741729129508371 ) ) ;
#19993=CARTESIAN_POINT ( 'NONE',  ( 107.0000000000000142, 110.0000000000000000, -45.00000000000000711 ) ) ;
#19996=CARTESIAN_POINT ( 'NONE',  ( 98.96446609406727646, 123.2500000000000000, -2.499999999999997780 ) ) ;
#20000=CARTESIAN_POINT ( 'NONE',  ( 102.0710678118654613, 94.68749999726883004, 4.999999999999983125 ) ) ;
#20003=CARTESIAN_POINT ( 'NONE',  ( 106.5389055433251002, 114.7507929638356785, -54.17500000273119554 ) ) ;
#20010=FACE_OUTER_BOUND ( 'NONE', #857, .T. ) ;
#20011=CARTESIAN_POINT ( 'NONE',  ( 84.99999999999998579, 95.00000000000000000, -15.00000000000000533 ) ) ;
#20015=( BOUNDED_SURFACE ( )  B_SPLINE_SURFACE ( 1, 2, ( 
 ( #3159, #11829, #20120, #26830, #27113, #11401, #24680, #7563, #22262, #16111, #13964, #598, #16257, #24957, #9278, #892, #14110, #20406, #17974, #7416, #9562, #26682, #7130, #22834, #5157, #3300, #9416, #18265, #15827, #5018, #11540, #13683, #22400, #24816, #5299, #27801, #10106, #18687, #27526, #3721, #1306, #14659, #3996, #7982, #27390, #12659, #21101, #1176, #8257, #7849, #5725, #9841, #3852, #14529, #12383, #20967, #25379, #25645, #1723, #12513, #23244, #18548, #27252, #16944, #1589, #9976, #14390, #10244, #27661, #14251, #16544, #25101, #23380, #21241, #18819, #16680, #25234, #7710, #12102, #20829, #3581 ),
 ( #23107, #1450, #8123, #16403, #5586, #10385, #22972, #5859, #16818, #18952, #25515, #12239, #5994, #19092, #6129, #14794, #23517, #3436, #12928, #26067, #26211, #21660, #6673, #10801, #28074, #2282, #4945, #26751, #17371, #25930, #9343, #10663, #13607, #24606, #23657, #11467, #20186, #8681, #670, #1996, #27935, #5084, #6536, #22329, #18038, #19371, #19514, #2136, #15214, #8539, #21385, #15359, #23933, #17225, #10940, #4412, #7193, #13067, #6405, #15890, #15074, #2800, #1863, #4133, #10528, #19234, #21804, #8394, #23792, #17083, #25785, #19652, #6263, #14936, #4269, #134, #8820, #17509, #24074, #12797, #21517 ) ),
 .UNSPECIFIED., .F., .F., .F. ) 
 B_SPLINE_SURFACE_WITH_KNOTS ( ( 2, 2 ),
 ( 3, 2, 2, 2, 2, 2, 2, 2, 2, 2, 2, 2, 2, 2, 2, 2, 2, 2, 2, 2, 2, 2, 2, 2, 2, 2, 2, 2, 2, 2, 2, 2, 2, 2, 2, 2, 2, 2, 2, 2, 3 ),
 ( 0.000000000000000000, 1.000000000000000000 ),
 ( 0.000000000000000000, 0.02500000000000000139, 0.05000000000000000278, 0.07499999999999999722, 0.1000000000000000056, 0.1250000000000000000, 0.1499999999999999944, 0.1749999999999999889, 0.2000000000000000111, 0.2250000000000000056, 0.2500000000000000000, 0.2750000000000000222, 0.2999999999999999889, 0.3250000000000000111, 0.3499999999999999778, 0.3750000000000000000, 0.4000000000000000222, 0.4249999999999999889, 0.4500000000000000111, 0.4749999999999999778, 0.5000000000000000000, 0.5250000000000000222, 0.5500000000000000444, 0.5749999999999999556, 0.5999999999999999778, 0.6250000000000000000, 0.6500000000000000222, 0.6750000000000000444, 0.6999999999999999556, 0.7249999999999999778, 0.7500000000000000000, 0.7750000000000000222, 0.8000000000000000444, 0.8249999999999999556, 0.8499999999999999778, 0.8750000000000000000, 0.9000000000000000222, 0.9250000000000000444, 0.9499999999999999556, 0.9749999999999999778, 1.000000000000000000 ),
 .UNSPECIFIED. ) 
 GEOMETRIC_REPRESENTATION_ITEM ( )  RATIONAL_B_SPLINE_SURFACE ( (
 ( 1.000000000000000000, 0.9238795325112867385, 1.000000000000000000, 0.9238795325112867385, 1.000000000000000000, 0.9238795325112867385, 1.000000000000000000, 0.9238795325112867385, 1.000000000000000000, 0.9238795325112867385, 1.000000000000000000, 0.9238795325112867385, 1.000000000000000000, 0.9238795325112867385, 1.000000000000000000, 0.9238795325112867385, 1.000000000000000000, 0.9238795325112867385, 1.000000000000000000, 0.9238795325112867385, 1.000000000000000000, 0.9238795325112867385, 1.000000000000000000, 0.9238795325112867385, 1.000000000000000000, 0.9238795325112867385, 1.000000000000000000, 0.9238795325112867385, 1.000000000000000000, 0.9238795325112867385, 1.000000000000000000, 0.9238795325112867385, 1.000000000000000000, 0.9238795325112867385, 1.000000000000000000, 0.9238795325112867385, 1.000000000000000000, 0.9238795325112867385, 1.000000000000000000, 0.9238795325112867385, 1.000000000000000000, 0.9238795325112867385, 1.000000000000000000, 0.9238795325112867385, 1.000000000000000000, 0.9238795325112867385, 1.000000000000000000, 0.9238795325112867385, 1.000000000000000000, 0.9238795325112867385, 1.000000000000000000, 0.9238795325112867385, 1.000000000000000000, 0.9238795325112867385, 1.000000000000000000, 0.9238795325112867385, 1.000000000000000000, 0.9238795325112867385, 1.000000000000000000, 0.9238795325112867385, 1.000000000000000000, 0.9238795325112867385, 1.000000000000000000, 0.9238795325112867385, 1.000000000000000000, 0.9238795325112867385, 1.000000000000000000, 0.9238795325112867385, 1.000000000000000000, 0.9238795325112867385, 1.000000000000000000, 0.9238795325112867385, 1.000000000000000000, 0.9238795325112867385, 1.000000000000000000, 0.9238795325112867385, 1.000000000000000000, 0.9238795325112867385, 1.000000000000000000, 0.9238795325112867385, 1.000000000000000000),
 ( 1.000000000000000000, 0.9238795325112867385, 1.000000000000000000, 0.9238795325112867385, 1.000000000000000000, 0.9238795325112867385, 1.000000000000000000, 0.9238795325112867385, 1.000000000000000000, 0.9238795325112867385, 1.000000000000000000, 0.9238795325112867385, 1.000000000000000000, 0.9238795325112867385, 1.000000000000000000, 0.9238795325112867385, 1.000000000000000000, 0.9238795325112867385, 1.000000000000000000, 0.9238795325112867385, 1.000000000000000000, 0.9238795325112867385, 1.000000000000000000, 0.9238795325112867385, 1.000000000000000000, 0.9238795325112867385, 1.000000000000000000, 0.9238795325112867385, 1.000000000000000000, 0.9238795325112867385, 1.000000000000000000, 0.9238795325112867385, 1.000000000000000000, 0.9238795325112867385, 1.000000000000000000, 0.9238795325112867385, 1.000000000000000000, 0.9238795325112867385, 1.000000000000000000, 0.9238795325112867385, 1.000000000000000000, 0.9238795325112867385, 1.000000000000000000, 0.9238795325112867385, 1.000000000000000000, 0.9238795325112867385, 1.000000000000000000, 0.9238795325112867385, 1.000000000000000000, 0.9238795325112867385, 1.000000000000000000, 0.9238795325112867385, 1.000000000000000000, 0.9238795325112867385, 1.000000000000000000, 0.9238795325112867385, 1.000000000000000000, 0.9238795325112867385, 1.000000000000000000, 0.9238795325112867385, 1.000000000000000000, 0.9238795325112867385, 1.000000000000000000, 0.9238795325112867385, 1.000000000000000000, 0.9238795325112867385, 1.000000000000000000, 0.9238795325112867385, 1.000000000000000000, 0.9238795325112867385, 1.000000000000000000, 0.9238795325112867385, 1.000000000000000000, 0.9238795325112867385, 1.000000000000000000, 0.9238795325112867385, 1.000000000000000000, 0.9238795325112867385, 1.000000000000000000, 0.9238795325112867385, 1.000000000000000000) ) ) 
 REPRESENTATION_ITEM ( '' )  SURFACE ( )  );
#20032=CARTESIAN_POINT ( 'NONE',  ( 102.4976396683250925, 102.3130555110000159, -52.52500000273119696 ) ) ;
#20036=AXIS2_PLACEMENT_3D ( 'NONE', #17011, #25998, #25714 ) ;
#20040=CARTESIAN_POINT ( 'NONE',  ( 97.93301269999999192, 123.7000000010924765, -0.8561741729129505041 ) ) ;
#20049=( BOUNDED_CURVE ( )  B_SPLINE_CURVE ( 2, ( #25091, #5435, #18256, #24948, #20398, #26964, #24672, #14102, #11821, #20684, #2863, #15820, #3426, #1167, #7408, #5578, #13955, #14243, #20544, #735, #24808, #24526, #16102, #11531, #5291, #22964, #20248, #5011, #9407, #12093, #16393, #3152, #18107, #15957, #5149, #27104, #13813, #1026, #9697, #7555, #14784, #12229, #18810, #1853, #8247, #10098, #12502, #8112, #1579, #3572, #23369, #25635, #1714, #20957, #19082, #1440, #5715, #3711, #21505, #18679, #27517, #7972, #14381, #21374, #16807, #25774, #16534, #14650, #23506, #21230, #27652, #10516, #10375, #27788, #19224, #16935, #23097, #25505, #12787, #21091, #27381 ),
 .UNSPECIFIED., .F., .F. ) 
 B_SPLINE_CURVE_WITH_KNOTS ( ( 3, 2, 2, 2, 2, 2, 2, 2, 2, 2, 2, 2, 2, 2, 2, 2, 2, 2, 2, 2, 2, 2, 2, 2, 2, 2, 2, 2, 2, 2, 2, 2, 2, 2, 2, 2, 2, 2, 2, 2, 3 ),
 ( 0.000000000000000000, 0.02500000000000000139, 0.05000000000000000278, 0.07499999999999999722, 0.1000000000000000056, 0.1250000000000000000, 0.1499999999999999944, 0.1749999999999999889, 0.2000000000000000111, 0.2250000000000000056, 0.2500000000000000000, 0.2750000000000000222, 0.2999999999999999889, 0.3250000000000000111, 0.3499999999999999778, 0.3750000000000000000, 0.4000000000000000222, 0.4249999999999999889, 0.4500000000000000111, 0.4749999999999999778, 0.5000000000000000000, 0.5250000000000000222, 0.5500000000000000444, 0.5749999999999999556, 0.5999999999999999778, 0.6250000000000000000, 0.6500000000000000222, 0.6750000000000000444, 0.6999999999999999556, 0.7249999999999999778, 0.7500000000000000000, 0.7750000000000000222, 0.8000000000000000444, 0.8249999999999999556, 0.8499999999999999778, 0.8750000000000000000, 0.9000000000000000222, 0.9250000000000000444, 0.9499999999999999556, 0.9749999999999999778, 1.000000000000000000 ),
 .UNSPECIFIED. ) 
 CURVE ( )  GEOMETRIC_REPRESENTATION_ITEM ( )  RATIONAL_B_SPLINE_CURVE ( ( 1.000000000000000000, 0.9238795325112867385, 1.000000000000000000, 0.9238795325112867385, 1.000000000000000000, 0.9238795325112867385, 1.000000000000000000, 0.9238795325112867385, 1.000000000000000000, 0.9238795325112867385, 1.000000000000000000, 0.9238795325112867385, 1.000000000000000000, 0.9238795325112867385, 1.000000000000000000, 0.9238795325112867385, 1.000000000000000000, 0.9238795325112867385, 1.000000000000000000, 0.9238795325112867385, 1.000000000000000000, 0.9238795325112867385, 1.000000000000000000, 0.9238795325112867385, 1.000000000000000000, 0.9238795325112867385, 1.000000000000000000, 0.9238795325112867385, 1.000000000000000000, 0.9238795325112867385, 1.000000000000000000, 0.9238795325112867385, 1.000000000000000000, 0.9238795325112867385, 1.000000000000000000, 0.9238795325112867385, 1.000000000000000000, 0.9238795325112867385, 1.000000000000000000, 0.9238795325112867385, 1.000000000000000000, 0.9238795325112867385, 1.000000000000000000, 0.9238795325112867385, 1.000000000000000000, 0.9238795325112867385, 1.000000000000000000, 0.9238795325112867385, 1.000000000000000000, 0.9238795325112867385, 1.000000000000000000, 0.9238795325112867385, 1.000000000000000000, 0.9238795325112867385, 1.000000000000000000, 0.9238795325112867385, 1.000000000000000000, 0.9238795325112867385, 1.000000000000000000, 0.9238795325112867385, 1.000000000000000000, 0.9238795325112867385, 1.000000000000000000, 0.9238795325112867385, 1.000000000000000000, 0.9238795325112867385, 1.000000000000000000, 0.9238795325112867385, 1.000000000000000000, 0.9238795325112867385, 1.000000000000000000, 0.9238795325112867385, 1.000000000000000000, 0.9238795325112867385, 1.000000000000000000, 0.9238795325112867385, 1.000000000000000000, 0.9238795325112867385, 1.000000000000000000, 0.9238795325112867385, 1.000000000000000000 ) ) 
 REPRESENTATION_ITEM ( '' )  );
#20062=EDGE_CURVE ( 'NONE', #3615, #2259, #20775, .T. ) ;
#20071=CARTESIAN_POINT ( 'NONE',  ( 101.7677669529663547, 124.7069999999781515, -1.767766952966370209 ) ) ;
#20072=( LENGTH_UNIT ( ) NAMED_UNIT ( * ) SI_UNIT ( .MILLI., .METRE. ) );
#20083=CARTESIAN_POINT ( 'NONE',  ( 91.00000000000000000, 110.0000000000000000, -55.00000000000000711 ) ) ;
#20084=CARTESIAN_POINT ( 'NONE',  ( 107.0000000000000142, 110.0000000000000000, -45.50000000546238255 ) ) ;
#20096=CARTESIAN_POINT ( 'NONE',  ( 103.5355339059327235, 93.12500000000000000, -3.535533905932738197 ) ) ;
#20097=CARTESIAN_POINT ( 'NONE',  ( 104.4587341249999923, 94.49999999863442213, 1.846868145590726318 ) ) ;
#20101=VERTEX_POINT ( 'NONE', #20332 ) ;
#20110=CARTESIAN_POINT ( 'NONE',  ( 114.9999999999999858, 125.0000000000000000, 14.99999999999998934 ) ) ;
#20119=CARTESIAN_POINT ( 'NONE',  ( 95.00472066334982912, 103.1245878333314323, -48.82500000273118701 ) ) ;
#20120=CARTESIAN_POINT ( 'NONE',  ( 103.1528011352953484, 90.68749999863440792, -3.152801135295366208 ) ) ;
#20121=CYLINDRICAL_SURFACE ( 'NONE', #12519, 5.000000000000004441 ) ;
#20125=DIRECTION ( 'NONE',  ( -0.000000000000000000, -0.000000000000000000, 1.000000000000000000 ) ) ;
#20129=( BOUNDED_CURVE ( )  B_SPLINE_CURVE ( 2, ( #15244, #12405, #17112, #25816, #1751, #3880, #23823, #10829, #14823, #2166, #6291 ),
 .UNSPECIFIED., .F., .T. ) 
 B_SPLINE_CURVE_WITH_KNOTS ( ( 3, 2, 2, 2, 2, 3 ),
 ( 0.8000000000000000444, 0.8199999999999999512, 0.8399999999999999689, 0.8599999999999999867, 0.8800000000000000044, 0.9000000000000000222 ),
 .UNSPECIFIED. ) 
 CURVE ( )  GEOMETRIC_REPRESENTATION_ITEM ( )  RATIONAL_B_SPLINE_CURVE ( ( 1.000000000000000000, 0.9510565162951535312, 1.000000000000000000, 0.9510565162951535312, 1.000000000000000000, 0.9510565162951535312, 1.000000000000000000, 0.9510565162951535312, 1.000000000000000000, 0.9510565162951535312, 1.000000000000000000 ) ) 
 REPRESENTATION_ITEM ( '' )  );
#20135=CARTESIAN_POINT ( 'NONE',  ( 106.5389055433251002, 114.7507929638356785, -54.17500000273119554 ) ) ;
#20137=CARTESIAN_POINT ( 'NONE',  ( 98.96446609406727646, 124.8500000000000085, -2.499999999999997780 ) ) ;
#20140=CARTESIAN_POINT ( 'NONE',  ( 84.99999999999998579, 125.0000000000000000, -15.00000000000000888 ) ) ;
#20142=CARTESIAN_POINT ( 'NONE',  ( 95.00000000000000000, 95.43749999726880162, 2.071067811865463959 ) ) ;
#20145=CARTESIAN_POINT ( 'NONE',  ( 95.00472066334981491, 103.1245878333314465, -53.07500000273118701 ) ) ;
#20148=EDGE_CURVE ( 'NONE', #27429, #613, #16035, .T. ) ;
#20152=CARTESIAN_POINT ( 'NONE',  ( 99.99999999999998579, 90.00000000000000000, -6.938893903907228378E-15 ) ) ;
#20157=CARTESIAN_POINT ( 'NONE',  ( 98.15313185440923860, 91.24999999863439371, 4.458734124999980786 ) ) ;
#20163=ORIENTED_EDGE ( 'NONE', *, *, #8912, .T. ) ;
#20174=CARTESIAN_POINT ( 'NONE',  ( 95.00472066334981491, 116.8754121666685393, -47.42500000273119554 ) ) ;
#20175=CARTESIAN_POINT ( 'NONE',  ( 84.99999999999998579, 125.0000000000000000, -15.00000000000000888 ) ) ;
#20180=CARTESIAN_POINT ( 'NONE',  ( 101.0355339059327378, 122.9500000021849502, 2.499999999999977796 ) ) ;
#20186=CARTESIAN_POINT ( 'NONE',  ( 99.99999999999998579, 92.56249999863440792, -4.458734124999994997 ) ) ;
#20187=CARTESIAN_POINT ( 'NONE',  ( 104.9952793366501851, 103.1245878333314323, -44.42500000273119554 ) ) ;
#20201=CARTESIAN_POINT ( 'NONE',  ( 104.4587341249999781, 95.43749999863440792, -6.938893903907228378E-15 ) ) ;
#20213=CARTESIAN_POINT ( 'NONE',  ( 104.3262379212492590, 115.9545556584642867, -54.70000000000000284 ) ) ;
#20223=CARTESIAN_POINT ( 'NONE',  ( 104.9952793366501851, 103.1245878333314323, -52.67500000273119554 ) ) ;
#20225=ORIENTED_EDGE ( 'NONE', *, *, #14698, .F. ) ;
#20226=CARTESIAN_POINT ( 'NONE',  ( 99.99999999999998579, 123.9500000010924765, 2.066987299999980099 ) ) ;
#20233=CARTESIAN_POINT ( 'NONE',  ( 97.92893218813452449, 90.68749999999998579, 4.999999999999983125 ) ) ;
#20234=CARTESIAN_POINT ( 'NONE',  ( 104.4587341249999781, 95.56249999863440792, -6.938893903907228378E-15 ) ) ;
#20248=CARTESIAN_POINT ( 'NONE',  ( 96.84719886470463734, 91.93749999863440792, 3.152801135295351997 ) ) ;
#20253=EDGE_CURVE ( 'NONE', #8168, #3810, #20617, .T. ) ;
#20256=CARTESIAN_POINT ( 'NONE',  ( 93.00000000000001421, 112.2744378736303332, -52.60000000546237686 ) ) ;
#20257=FACE_OUTER_BOUND ( 'NONE', #19656, .T. ) ;
#20258=CARTESIAN_POINT ( 'NONE',  ( 99.99999999999998579, 110.0000000000000000, 15.00099999999999412 ) ) ;
#20270=ORIENTED_EDGE ( 'NONE', *, *, #3693, .F. ) ;
#20271=CARTESIAN_POINT ( 'NONE',  ( 99.99999999999998579, 101.5015231886685854, -52.87500000273119838 ) ) ;
#20274=CARTESIAN_POINT ( 'NONE',  ( 97.50000000000000000, 124.2000000000000028, -9.540979117872439019E-15 ) ) ;
#20279=CARTESIAN_POINT ( 'NONE',  ( 98.15313185440925281, 91.87499999863439371, -4.458734124999994997 ) ) ;
#20281=CARTESIAN_POINT ( 'NONE',  ( 99.99999999999998579, 101.5015231886685712, -50.87500000273119127 ) ) ;
#20288=EDGE_CURVE ( 'NONE', #19120, #756, #9638, .T. ) ;
#20290=CARTESIAN_POINT ( 'NONE',  ( 103.5355339059327235, 90.99999999726880162, -3.535533905932738197 ) ) ;
#20296=CARTESIAN_POINT ( 'NONE',  ( 96.84719886470463734, 91.93749999863440792, -3.152801135295366208 ) ) ;
#20310=CARTESIAN_POINT ( 'NONE',  ( 99.99999999999998579, 91.62499999726880162, 4.999999999999984013 ) ) ;
#20313=CARTESIAN_POINT ( 'NONE',  ( 97.50236033167492167, 117.6869444889999841, -45.52500000273119696 ) ) ;
#20318=EDGE_LOOP ( 'NONE', ( #5868, #9387, #2671, #7475 ) ) ;
#20329=CARTESIAN_POINT ( 'NONE',  ( 108.0825317500000153, 110.0000000000000000, -44.12500000273119127 ) ) ;
#20332=CARTESIAN_POINT ( 'NONE',  ( 99.99999999999998579, 95.00000000000000000, -4.999999999999996447 ) ) ;
#20334=CARTESIAN_POINT ( 'NONE',  ( 97.92893218813452449, 91.56249999726883004, 4.999999999999983125 ) ) ;
#20336=VERTEX_POINT ( 'NONE', #10169 ) ;
#20355=CARTESIAN_POINT ( 'NONE',  ( 99.99999999999998579, 124.4069999999781402, 2.499999999999978684 ) ) ;
#20360=CARTESIAN_POINT ( 'NONE',  ( 109.0000000000000142, 110.0000000000000000, -55.00000000000000711 ) ) ;
#20370=CARTESIAN_POINT ( 'NONE',  ( 95.00472066334982912, 116.8754121666685393, -51.67500000273118133 ) ) ;
#20371=CARTESIAN_POINT ( 'NONE',  ( 99.35312936802752404, 123.0000000000000284, -2.419468906465395364 ) ) ;
#20372=ORIENTED_EDGE ( 'NONE', *, *, #25061, .F. ) ;
#20373=CARTESIAN_POINT ( 'NONE',  ( 98.53841926354351699, 123.6500000010924794, -1.461580736456474794 ) ) ;
#20380=CARTESIAN_POINT ( 'NONE',  ( 102.0710678118654613, 90.81249999999998579, 4.999999999999983125 ) ) ;
#20388=VERTEX_POINT ( 'NONE', #4341 ) ;
#20398=CARTESIAN_POINT ( 'NONE',  ( 99.99999999999998579, 90.56249999863440792, -4.458734124999994997 ) ) ;
#20403=CARTESIAN_POINT ( 'NONE',  ( 99.99999999999998579, 117.3602355696678643, -53.00000000546238255 ) ) ;
#20405=CARTESIAN_POINT ( 'NONE',  ( 106.5389055433251002, 105.2492070361643215, -46.32500000273119412 ) ) ;
#20406=CARTESIAN_POINT ( 'NONE',  ( 104.4587341249999923, 91.62499999863440792, -1.846868145590737198 ) ) ;
#20413=LINE ( 'NONE', #9569, #21148 ) ;
#20421=CARTESIAN_POINT ( 'NONE',  ( 93.46109445667491400, 105.2492070361643215, -53.17500000273119554 ) ) ;
#20430=CARTESIAN_POINT ( 'NONE',  ( 95.54126587500000767, 91.06249999863440792, -7.484931351350258973E-15 ) ) ;
#20432=CARTESIAN_POINT ( 'NONE',  ( 108.0825317500000153, 110.0000000000000000, -54.37500000273119838 ) ) ;
#20439=CARTESIAN_POINT ( 'NONE',  ( 99.99999999999998579, 91.12499999726880162, -4.999999999999997335 ) ) ;
#20441=VERTEX_POINT ( 'NONE', #28006 ) ;
#20445=CARTESIAN_POINT ( 'NONE',  ( 101.8468681455907330, 91.74999999863439371, -4.458734124999994997 ) ) ;
#20457=PLANE ( 'NONE',  #17686 ) ;
#20460=CARTESIAN_POINT ( 'NONE',  ( 108.0825317500000011, 112.6261737610028320, -50.02500000273118985 ) ) ;
#20465=EDGE_LOOP ( 'NONE', ( #25991, #19868, #28183, #19607, #13289, #24867, #12393, #10667 ) ) ;
#20470=VERTEX_POINT ( 'NONE', #6471 ) ;
#20476=CARTESIAN_POINT ( 'NONE',  ( 104.9999999999999716, 94.81249999726880162, 2.071067811865467956 ) ) ;
#20513=CARTESIAN_POINT ( 'NONE',  ( 99.99999999999998579, 97.00000000000000000, 2.999999999999982681 ) ) ;
#20515=CARTESIAN_POINT ( 'NONE',  ( 104.9952793366501851, 116.8754121666685393, -54.07500000273119412 ) ) ;
#20516=CARTESIAN_POINT ( 'NONE',  ( 99.99999999999998579, 94.25000000000000000, -4.999999999999997335 ) ) ;
#20517=CARTESIAN_POINT ( 'NONE',  ( 100.8561741729129153, 124.3000000010924708, -2.066987299999999195 ) ) ;
#20523=CARTESIAN_POINT ( 'NONE',  ( 104.3262379212492590, 115.9545556584642867, -50.70000000000000284 ) ) ;
#20524=AXIS2_PLACEMENT_3D ( 'NONE', #27765, #28177, #23622 ) ;
#20527=CARTESIAN_POINT ( 'NONE',  ( 96.46446609406726225, 94.37500000000000000, -3.535533905932738197 ) ) ;
#20544=CARTESIAN_POINT ( 'NONE',  ( 103.1528011352953484, 91.43749999863440792, -3.152801135295366208 ) ) ;
#20552=CARTESIAN_POINT ( 'NONE',  ( 97.83688103937538472, 116.6573956140660897, -48.90000000546238113 ) ) ;
#20553=CARTESIAN_POINT ( 'NONE',  ( 98.23223304703363112, 124.2000000021849502, -1.767766952966370209 ) ) ;
#20555=CARTESIAN_POINT ( 'NONE',  ( 99.99999999999998579, 90.00000000000000000, -6.938893903907228378E-15 ) ) ;
#20567=CARTESIAN_POINT ( 'NONE',  ( 106.5389055433251002, 105.2492070361643215, -46.57500000273119412 ) ) ;
#20573=CARTESIAN_POINT ( 'NONE',  ( 95.54126587499999346, 91.99999999863439371, -1.846868145590737864 ) ) ;
#20575=CARTESIAN_POINT ( 'NONE',  ( 106.5389055433251002, 105.2492070361643215, -50.57500000273120122 ) ) ;
#20586=CARTESIAN_POINT ( 'NONE',  ( 103.1528011352953484, 91.68749999863440792, -3.152801135295366208 ) ) ;
#20591=VERTEX_POINT ( 'NONE', #6198 ) ;
#20606=ORIENTED_EDGE ( 'NONE', *, *, #24542, .T. ) ;
#20614=CARTESIAN_POINT ( 'NONE',  ( 112.9999999999999858, 102.0000000000000142, -13.00000000000000711 ) ) ;
#20615=CARTESIAN_POINT ( 'NONE',  ( 99.99999999999998579, 101.5015231886685854, -44.62500000273119838 ) ) ;
#20617=LINE ( 'NONE', #24890, #5300 ) ;
#20643=CARTESIAN_POINT ( 'NONE',  ( 95.67376207875072680, 104.0454443415356991, -47.70000000000000284 ) ) ;
#20657=CARTESIAN_POINT ( 'NONE',  ( 99.14382582708707048, 123.9000000010924794, 2.066987299999979211 ) ) ;
#20662=CARTESIAN_POINT ( 'NONE',  ( 97.83688103937538472, 116.6573956140660897, -50.40000000000000568 ) ) ;
#20666=CARTESIAN_POINT ( 'NONE',  ( 104.9999999999999716, 91.93749999999998579, 2.071067811865467956 ) ) ;
#20668=EDGE_CURVE ( 'NONE', #20336, #20844, #9597, .T. ) ;
#20669=VECTOR ( 'NONE', #23602, 1000.000000000000000 ) ;
#20681=LINE ( 'NONE', #2860, #1634 ) ;
#20684=CARTESIAN_POINT ( 'NONE',  ( 95.54126587499999346, 90.87499999863439371, 1.846868145590722543 ) ) ;
#20686=EDGE_CURVE ( 'NONE', #5734, #24831, #12699, .T. ) ;
#20692=CARTESIAN_POINT ( 'NONE',  ( 105.6631189606246295, 105.8855032339526758, -47.70000000546237828 ) ) ;
#20693=CARTESIAN_POINT ( 'NONE',  ( 99.99999999999998579, 124.1000000021849416, -2.499999999999997780 ) ) ;
#20701=CARTESIAN_POINT ( 'NONE',  ( 99.99999999999998579, 91.25000000000000000, -4.999999999999997335 ) ) ;
#20708=CARTESIAN_POINT ( 'NONE',  ( 102.4976396683250925, 102.3130555110000159, -48.77500000273119696 ) ) ;
#20715=CARTESIAN_POINT ( 'NONE',  ( 98.15313185440925281, 90.87499999863439371, -4.458734124999994997 ) ) ;
#20716=CARTESIAN_POINT ( 'NONE',  ( 100.0000000000000000, 110.0000000000000000, -55.00000000000000711 ) ) ;
#20727=CARTESIAN_POINT ( 'NONE',  ( 98.15313185440923860, 93.87499999863439371, -4.458734124999994997 ) ) ;
#20730=VECTOR ( 'NONE', #26258, 1000.000000000000000 ) ;
#20742=EDGE_CURVE ( 'NONE', #6897, #26002, #6034, .T. ) ;
#20748=ORIENTED_EDGE ( 'NONE', *, *, #23297, .F. ) ;
#20759=ORIENTED_EDGE ( 'NONE', *, *, #25297, .T. ) ;
#20770=FACE_OUTER_BOUND ( 'NONE', #17309, .T. ) ;
#20775=CIRCLE ( 'NONE', #8469, 2.999999999999989786 ) ;
#20777=CARTESIAN_POINT ( 'NONE',  ( 98.23223304703363112, 123.5069999999781487, 1.767766952966351557 ) ) ;
#20784=LINE ( 'NONE', #9929, #3433 ) ;
#20792=CARTESIAN_POINT ( 'NONE',  ( 99.99999999999998579, 118.4984768113314004, -47.87500000273119127 ) ) ;
#20795=CARTESIAN_POINT ( 'NONE',  ( 102.0669872999999939, 124.1000000010924964, 0.8561741729129311862 ) ) ;
#20801=CARTESIAN_POINT ( 'NONE',  ( 99.99999999999998579, 92.25000000000000000, -4.999999999999997335 ) ) ;
#20812=AXIS2_PLACEMENT_3D ( 'NONE', #26679, #19682, #11398 ) ;
#20828=CARTESIAN_POINT ( 'NONE',  ( 107.0000000000000142, 112.2744378736303332, -49.40000000546237402 ) ) ;
#20829=CARTESIAN_POINT ( 'NONE',  ( 104.4587341249999923, 95.49999999863442213, 1.846868145590726318 ) ) ;
#20843=ADVANCED_FACE ( 'NONE', ( #25971 ), #2038, .F. ) ;
#20844=VERTEX_POINT ( 'NONE', #22232 ) ;
#20845=CARTESIAN_POINT ( 'NONE',  ( 97.50236033167492167, 117.6869444889999841, -47.77500000273119696 ) ) ;
#20851=CARTESIAN_POINT ( 'NONE',  ( 103.1528011352953484, 90.68749999863440792, -3.152801135295366208 ) ) ;
#20854=VERTEX_POINT ( 'NONE', #14835 ) ;
#20861=ORIENTED_EDGE ( 'NONE', *, *, #25711, .T. ) ;
#20867=DIRECTION ( 'NONE',  ( 5.782411586589357392E-17, -0.000000000000000000, 1.000000000000000000 ) ) ;
#20875=CARTESIAN_POINT ( 'NONE',  ( 97.83688103937538472, 116.6573956140660897, -54.40000000000000568 ) ) ;
#20884=ORIENTED_EDGE ( 'NONE', *, *, #13236, .T. ) ;
#20885=SHAPE_REPRESENTATION_RELATIONSHIP ( 'NONE' , 'NONE' ,  #26810, #19902 ) ;
#20900=ORIENTED_EDGE ( 'NONE', *, *, #26414, .F. ) ;
#20901=LINE ( 'NONE', #7642, #867 ) ;
#20908=DIRECTION ( 'NONE',  ( -0.000000000000000000, 1.000000000000000000, -0.000000000000000000 ) ) ;
#20912=CARTESIAN_POINT ( 'NONE',  ( 93.00000000000000000, 110.0000000000000000, -52.50000000546237544 ) ) ;
#20916=CARTESIAN_POINT ( 'NONE',  ( 101.0355339059327378, 124.4500000000000028, 2.499999999999977796 ) ) ;
#20923=ORIENTED_EDGE ( 'NONE', *, *, #24846, .T. ) ;
#20930=CARTESIAN_POINT ( 'NONE',  ( 91.91746824999998466, 112.6261737610028320, -49.47500000273119269 ) ) ;
#20931=CYLINDRICAL_SURFACE ( 'NONE', #24144, 2.499999999999995115 ) ;
#20932=CARTESIAN_POINT ( 'NONE',  ( 101.4615807364564546, 123.4500000010924765, 1.461580736456455476 ) ) ;
#20938=EDGE_CURVE ( 'NONE', #6173, #25694, #27841, .T. ) ;
#20939=( BOUNDED_CURVE ( )  B_SPLINE_CURVE ( 2, ( #20432, #2763, #20003, #13706, #4902, #26562, #2895, #15989, #18431, #767, #9301, #18141, #22572, #20145, #13988, #23235, #26854, #17998, #3712, #11708, #483, #15851, #24845, #13564, #7014, #11564, #17857, #22713, #15710, #7302, #7590, #3183, #18289, #9728, #11853, #20281, #3038, #626, #20575, #9165, #24703, #27139, #24560, #1056, #5849, #5042, #16283, #22287, #24412, #9441, #11426, #24984, #26706, #5183, #14520, #7155, #26995, #22424, #13846, #915, #9585, #7441, #16137, #21511, #4263, #21798, #19365, #4407, #15649, #28068, #21655, #2557, #12793, #15068, #17646, #6954, #26205, #11218, #10936, #8675, #16769, #22080, #17795, #17366, #24069, #2131, #17504, #4545, #12923, #21941, #24348, #13207, #26062, #19647, #10658, #2419, #1991, #23787, #129, #24212, #6531 ),
 .UNSPECIFIED., .F., .F. ) 
 B_SPLINE_CURVE_WITH_KNOTS ( ( 3, 2, 2, 2, 2, 2, 2, 2, 2, 2, 2, 2, 2, 2, 2, 2, 2, 2, 2, 2, 2, 2, 2, 2, 2, 2, 2, 2, 2, 2, 2, 2, 2, 2, 2, 2, 2, 2, 2, 2, 2, 2, 2, 2, 2, 2, 2, 2, 2, 2, 3 ),
 ( 0.000000000000000000, 0.02000000000000000042, 0.04000000000000000083, 0.05999999999999999778, 0.08000000000000000167, 0.1000000000000000056, 0.1199999999999999956, 0.1400000000000000133, 0.1600000000000000033, 0.1799999999999999933, 0.2000000000000000111, 0.2200000000000000011, 0.2399999999999999911, 0.2600000000000000089, 0.2800000000000000266, 0.2999999999999999889, 0.3200000000000000067, 0.3400000000000000244, 0.3599999999999999867, 0.3800000000000000044, 0.4000000000000000222, 0.4199999999999999845, 0.4400000000000000022, 0.4600000000000000200, 0.4799999999999999822, 0.5000000000000000000, 0.5200000000000000178, 0.5400000000000000355, 0.5600000000000000533, 0.5799999999999999600, 0.5999999999999999778, 0.6199999999999999956, 0.6400000000000000133, 0.6600000000000000311, 0.6800000000000000488, 0.6999999999999999556, 0.7199999999999999734, 0.7399999999999999911, 0.7600000000000000089, 0.7800000000000000266, 0.8000000000000000444, 0.8199999999999999512, 0.8399999999999999689, 0.8599999999999999867, 0.8800000000000000044, 0.9000000000000000222, 0.9200000000000000400, 0.9399999999999999467, 0.9599999999999999645, 0.9799999999999999822, 1.000000000000000000 ),
 .UNSPECIFIED. ) 
 CURVE ( )  GEOMETRIC_REPRESENTATION_ITEM ( )  RATIONAL_B_SPLINE_CURVE ( ( 1.000000000000000000, 0.9510565162951535312, 1.000000000000000000, 0.9510565162951535312, 1.000000000000000000, 0.9510565162951535312, 1.000000000000000000, 0.9510565162951535312, 1.000000000000000000, 0.9510565162951535312, 1.000000000000000000, 0.9510565162951535312, 1.000000000000000000, 0.9510565162951535312, 1.000000000000000000, 0.9510565162951535312, 1.000000000000000000, 0.9510565162951535312, 1.000000000000000000, 0.9510565162951535312, 1.000000000000000000, 0.9510565162951535312, 1.000000000000000000, 0.9510565162951535312, 1.000000000000000000, 0.9510565162951535312, 1.000000000000000000, 0.9510565162951535312, 1.000000000000000000, 0.9510565162951535312, 1.000000000000000000, 0.9510565162951535312, 1.000000000000000000, 0.9510565162951535312, 1.000000000000000000, 0.9510565162951535312, 1.000000000000000000, 0.9510565162951535312, 1.000000000000000000, 0.9510565162951535312, 1.000000000000000000, 0.9510565162951535312, 1.000000000000000000, 0.9510565162951535312, 1.000000000000000000, 0.9510565162951535312, 1.000000000000000000, 0.9510565162951535312, 1.000000000000000000, 0.9510565162951535312, 1.000000000000000000, 0.9510565162951535312, 1.000000000000000000, 0.9510565162951535312, 1.000000000000000000, 0.9510565162951535312, 1.000000000000000000, 0.9510565162951535312, 1.000000000000000000, 0.9510565162951535312, 1.000000000000000000, 0.9510565162951535312, 1.000000000000000000, 0.9510565162951535312, 1.000000000000000000, 0.9510565162951535312, 1.000000000000000000, 0.9510565162951535312, 1.000000000000000000, 0.9510565162951535312, 1.000000000000000000, 0.9510565162951535312, 1.000000000000000000, 0.9510565162951535312, 1.000000000000000000, 0.9510565162951535312, 1.000000000000000000, 0.9510565162951535312, 1.000000000000000000, 0.9510565162951535312, 1.000000000000000000, 0.9510565162951535312, 1.000000000000000000, 0.9510565162951535312, 1.000000000000000000, 0.9510565162951535312, 1.000000000000000000, 0.9510565162951535312, 1.000000000000000000, 0.9510565162951535312, 1.000000000000000000, 0.9510565162951535312, 1.000000000000000000, 0.9510565162951535312, 1.000000000000000000, 0.9510565162951535312, 1.000000000000000000, 0.9510565162951535312, 1.000000000000000000, 0.9510565162951535312, 1.000000000000000000 ) ) 
 REPRESENTATION_ITEM ( '' )  );
#20942=CARTESIAN_POINT ( 'NONE',  ( 97.92893218813452449, 94.68749999999998579, 4.999999999999983125 ) ) ;
#20946=ORIENTED_EDGE ( 'NONE', *, *, #13074, .T. ) ;
#20957=CARTESIAN_POINT ( 'NONE',  ( 98.15313185440923860, 93.62499999863439371, -4.458734124999994997 ) ) ;
#20961=FACE_OUTER_BOUND ( 'NONE', #3484, .T. ) ;
#20963=CARTESIAN_POINT ( 'NONE',  ( 98.96446609406724804, 123.2499999999999716, -2.499999999999993339 ) ) ;
#20966=CARTESIAN_POINT ( 'NONE',  ( 95.67376207875072680, 104.0454443415356991, -46.20000000546237118 ) ) ;
#20967=CARTESIAN_POINT ( 'NONE',  ( 95.54126587499999346, 93.99999999863439371, -1.846868145590737864 ) ) ;
#20969=CARTESIAN_POINT ( 'NONE',  ( 102.4999999999999858, 122.3000000021849587, -9.847140817659276890E-15 ) ) ;
#20973=VECTOR ( 'NONE', #17465, 1000.000000000000000 ) ;
#20982=CARTESIAN_POINT ( 'NONE',  ( 108.0825317500000011, 107.3738262389971538, -44.47500000273118559 ) ) ;
#20984=CYLINDRICAL_SURFACE ( 'NONE', #12215, 4.999999999999989342 ) ;
#20986=CARTESIAN_POINT ( 'NONE',  ( 95.00472066334981491, 103.1245878333314465, -48.82500000273119412 ) ) ;
#20989=AXIS2_PLACEMENT_3D ( 'NONE', #11595, #9754, #6909 ) ;
#21000=LINE ( 'NONE', #8014, #4229 ) ;
#21005=CARTESIAN_POINT ( 'NONE',  ( 101.8468681455907330, 92.74999999863439371, -4.458734124999994997 ) ) ;
#21014=( BOUNDED_CURVE ( )  B_SPLINE_CURVE ( 2, ( #15284, #15427, #8463, #6742, #11143 ),
 .UNSPECIFIED., .F., .F. ) 
 B_SPLINE_CURVE_WITH_KNOTS ( ( 3, 2, 3 ),
 ( 0.9500000000000009548, 0.9750000000000005329, 1.000000000000000000 ),
 .UNSPECIFIED. ) 
 CURVE ( )  GEOMETRIC_REPRESENTATION_ITEM ( )  RATIONAL_B_SPLINE_CURVE ( ( 0.9999999999999970024, 0.9238795325112897361, 1.000000000000000000, 0.9238795325112867385, 1.000000000000000000 ) ) 
 REPRESENTATION_ITEM ( '' )  );
#21027=CARTESIAN_POINT ( 'NONE',  ( 104.9999999999999716, 90.93749999999998579, 2.071067811865467956 ) ) ;
#21029=CARTESIAN_POINT ( 'NONE',  ( 99.99999999999998579, 89.99899999999999523, -9.540979117872439019E-15 ) ) ;
#21031=CARTESIAN_POINT ( 'NONE',  ( 84.99999999999998579, 120.0000000000000000, -15.00000000000000533 ) ) ;
#21036=VERTEX_POINT ( 'NONE', #24930 ) ;
#21054=CARTESIAN_POINT ( 'NONE',  ( 102.4999999999999716, 123.7569999999781771, 1.035533905932722876 ) ) ;
#21062=VECTOR ( 'NONE', #8808, 1000.000000000000000 ) ;
#21067=CARTESIAN_POINT ( 'NONE',  ( 95.00472066334982912, 103.1245878333314323, -47.07500000273119412 ) ) ;
#21081=VERTEX_POINT ( 'NONE', #20801 ) ;
#21084=CARTESIAN_POINT ( 'NONE',  ( 107.0000000000000142, 112.2744378736303332, -52.90000000000001279 ) ) ;
#21091=CARTESIAN_POINT ( 'NONE',  ( 104.4587341249999923, 95.24999999863437949, 1.846868145590726318 ) ) ;
#21100=CARTESIAN_POINT ( 'NONE',  ( 97.83688103937537051, 103.3426043859339103, -46.10000000546238397 ) ) ;
#21101=CARTESIAN_POINT ( 'NONE',  ( 103.1528011352953484, 93.43749999863440792, 3.152801135295352886 ) ) ;
#21108=CARTESIAN_POINT ( 'NONE',  ( 101.8468681455907330, 90.49999999863442213, -4.458734124999994997 ) ) ;
#21109=ORIENTED_EDGE ( 'NONE', *, *, #13826, .F. ) ;
#21114=ORIENTED_EDGE ( 'NONE', *, *, #11950, .T. ) ;
#21115=CARTESIAN_POINT ( 'NONE',  ( 108.0825317500000153, 110.0000000000000000, -46.37500000273119838 ) ) ;
#21119=CARTESIAN_POINT ( 'NONE',  ( 97.50236033167492167, 117.6869444889999841, -49.52500000273119696 ) ) ;
#21122=EDGE_CURVE ( 'NONE', #14157, #22191, #4907, .T. ) ;
#21130=( BOUNDED_CURVE ( )  B_SPLINE_CURVE ( 2, ( #524, #9205, #16741, #5644, #6059, #16877, #3780, #1373, #6194, #23308, #14864 ),
 .UNSPECIFIED., .F., .F. ) 
 B_SPLINE_CURVE_WITH_KNOTS ( ( 3, 2, 2, 2, 2, 3 ),
 ( 0.1000000000000000056, 0.1200000000000000233, 0.1400000000000000688, 0.1600000000000001144, 0.1800000000000001044, 0.2000000000000001776 ),
 .UNSPECIFIED. ) 
 CURVE ( )  GEOMETRIC_REPRESENTATION_ITEM ( )  RATIONAL_B_SPLINE_CURVE ( ( 1.000000000000000000, 0.9510565162951535312, 1.000000000000000000, 0.9510565162951535312, 1.000000000000000000, 0.9510565162951535312, 1.000000000000000000, 0.9510565162951535312, 1.000000000000000000, 0.9510565162951530871, 1.000000000000000444 ) ) 
 REPRESENTATION_ITEM ( '' )  );
#21138=CARTESIAN_POINT ( 'NONE',  ( 99.99999999999998579, 91.12499999726880162, -4.999999999999997335 ) ) ;
#21145=EDGE_CURVE ( 'NONE', #12415, #11020, #25073, .T. ) ;
#21147=FACE_OUTER_BOUND ( 'NONE', #23315, .T. ) ;
#21148=VECTOR ( 'NONE', #26979, 1000.000000000000000 ) ;
#21156=EDGE_LOOP ( 'NONE', ( #2722, #19959, #21891, #1921 ) ) ;
#21164=CYLINDRICAL_SURFACE ( 'NONE', #798, 2.499999999999995115 ) ;
#21165=DIRECTION ( 'NONE',  ( 5.782411586589357392E-17, -0.000000000000000000, 1.000000000000000000 ) ) ;
#21167=VECTOR ( 'NONE', #23874, 1000.000000000000000 ) ;
#21183=ADVANCED_FACE ( 'NONE', ( #19064, #3554 ), #12630, .T. ) ;
#21185=VECTOR ( 'NONE', #3843, 1000.000000000000000 ) ;
#21188=CARTESIAN_POINT ( 'NONE',  ( 98.96446609406727646, 123.2500000000000000, -2.499999999999997780 ) ) ;
#21190=CARTESIAN_POINT ( 'NONE',  ( 101.4615807364564546, 123.6500000010924651, -1.461580736456474794 ) ) ;
#21194=DIRECTION ( 'NONE',  ( 0.000000000000000000, 0.000000000000000000, 1.000000000000000000 ) ) ;
#21196=ORIENTED_EDGE ( 'NONE', *, *, #2308, .T. ) ;
#21205=CARTESIAN_POINT ( 'NONE',  ( 95.00472066334982912, 103.1245878333314323, -49.07500000273118701 ) ) ;
#21207=CARTESIAN_POINT ( 'NONE',  ( 102.0669872999999939, 124.3000000010924566, 0.8561741729129311862 ) ) ;
#21214=( BOUNDED_CURVE ( )  B_SPLINE_CURVE ( 2, ( #23326, #8343, #17029, #21605, #19884 ),
 .UNSPECIFIED., .F., .F. ) 
 B_SPLINE_CURVE_WITH_KNOTS ( ( 3, 2, 3 ),
 ( 0.000000000000000000, 0.04166666666666694885, 0.08333333333333389770 ),
 .UNSPECIFIED. ) 
 CURVE ( )  GEOMETRIC_REPRESENTATION_ITEM ( )  RATIONAL_B_SPLINE_CURVE ( ( 1.000000000000000000, 0.9238795325112867385, 1.000000000000000000, 0.9238795325112857393, 1.000000000000001110 ) ) 
 REPRESENTATION_ITEM ( '' )  );
#21216=CARTESIAN_POINT ( 'NONE',  ( 95.00000000000000000, 94.43750000000001421, -2.071067811865479058 ) ) ;
#21230=CARTESIAN_POINT ( 'NONE',  ( 98.15313185440923860, 94.62499999863439371, -4.458734124999994997 ) ) ;
#21241=CARTESIAN_POINT ( 'NONE',  ( 95.54126587499999346, 95.12499999863439371, 1.846868145590722543 ) ) ;
#21249=ORIENTED_EDGE ( 'NONE', *, *, #2022, .T. ) ;
#21253=CIRCLE ( 'NONE', #24898, 7.000000000000006217 ) ;
#21267=DIRECTION ( 'NONE',  ( -0.8660254037844380415, 0.5000000000000013323, 0.000000000000000000 ) ) ;
#21271=CIRCLE ( 'NONE', #818, 2.999999999999989786 ) ;
#21276=ORIENTED_EDGE ( 'NONE', *, *, #25620, .F. ) ;
#21280=CARTESIAN_POINT ( 'NONE',  ( 100.0000000000000000, 110.0000000000000000, -45.00000000000000711 ) ) ;
#21289=FACE_OUTER_BOUND ( 'NONE', #13737, .T. ) ;
#21290=DIRECTION ( 'NONE',  ( 1.000000000000000000, 0.000000000000000000, 0.000000000000000000 ) ) ;
#21291=CARTESIAN_POINT ( 'NONE',  ( 100.8561741729129295, 123.4000000010924794, 2.066987299999979211 ) ) ;
#21297=CARTESIAN_POINT ( 'NONE',  ( 84.99999999999998579, 118.0000000000000000, -43.00000000000000000 ) ) ;
#21299=ORIENTED_EDGE ( 'NONE', *, *, #27513, .T. ) ;
#21314=PRODUCT_DEFINITION_FORMATION_WITH_SPECIFIED_SOURCE ( 'ANY', '', #11714, .NOT_KNOWN. ) ;
#21320=EDGE_CURVE ( 'NONE', #7134, #4950, #3621, .T. ) ;
#21329=CARTESIAN_POINT ( 'NONE',  ( 102.4999999999999858, 123.8069999999781459, -9.847140817659276890E-15 ) ) ;
#21332=EDGE_CURVE ( 'NONE', #11286, #20591, #4737, .T. ) ;
#21334=CARTESIAN_POINT ( 'NONE',  ( 99.99999999999998579, 123.7500000010924737, -2.066987299999998751 ) ) ;
#21335=AXIS2_PLACEMENT_3D ( 'NONE', #5148, #13812, #22534 ) ;
#21339=CARTESIAN_POINT ( 'NONE',  ( 95.67376207875072680, 104.0454443415356991, -53.69999999999999574 ) ) ;
#21347=CARTESIAN_POINT ( 'NONE',  ( 104.9952793366501851, 116.8754121666685393, -48.07500000273119412 ) ) ;
#21350=CARTESIAN_POINT ( 'NONE',  ( 101.4615807364564546, 124.2500000010924737, 1.461580736456455476 ) ) ;
#21374=CARTESIAN_POINT ( 'NONE',  ( 104.4587341249999923, 94.24999999863439371, 1.846868145590726318 ) ) ;
#21383=CARTESIAN_POINT ( 'NONE',  ( 95.67376207875072680, 104.0454443415356991, -44.20000000546236407 ) ) ;
#21385=CARTESIAN_POINT ( 'NONE',  ( 103.1528011352953484, 93.43749999863440792, -3.152801135295366208 ) ) ;
#21389=CARTESIAN_POINT ( 'NONE',  ( 93.00000000000000000, 107.7255621263696668, -45.90000000000000568 ) ) ;
#21416=CARTESIAN_POINT ( 'NONE',  ( 99.99999999999998579, 118.4984768113314004, -51.62500000273119127 ) ) ;
#21424=CARTESIAN_POINT ( 'NONE',  ( 100.8561741729129295, 124.3000000010924850, -2.066987299999998751 ) ) ;
#21434=CARTESIAN_POINT ( 'NONE',  ( 105.6631189606246295, 114.1144967660473242, -50.80000000000000426 ) ) ;
#21436=CARTESIAN_POINT ( 'NONE',  ( 104.9999999999999716, 92.81249999726880162, 2.071067811865467956 ) ) ;
#21440=VECTOR ( 'NONE', #14782, 1000.000000000000000 ) ;
#21449=CARTESIAN_POINT ( 'NONE',  ( 101.7677669209684552, 123.0000000000000000, 1.767766984964258992 ) ) ;
#21451=DIRECTION ( 'NONE',  ( 1.000000000000000000, 0.000000000000000000, -5.782411586589357392E-17 ) ) ;
#21455=ORIENTED_EDGE ( 'NONE', *, *, #19965, .T. ) ;
#21468=DIRECTION ( 'NONE',  ( 1.000000000000000000, 0.000000000000000000, 0.000000000000000000 ) ) ;
#21472=CARTESIAN_POINT ( 'NONE',  ( 98.23223304703363112, 122.6000000021849559, -1.767766952966370209 ) ) ;
#21475=CARTESIAN_POINT ( 'NONE',  ( 104.3262379212492590, 104.0454443415356991, -47.80000000546237260 ) ) ;
#21481=CARTESIAN_POINT ( 'NONE',  ( 108.0825317500000011, 112.6261737610028320, -52.02500000273118985 ) ) ;
#21483=CARTESIAN_POINT ( 'NONE',  ( 100.8561741729129153, 122.7000000010924623, -2.066987299999999195 ) ) ;
#21500=VECTOR ( 'NONE', #7330, 1000.000000000000000 ) ;
#21503=( BOUNDED_CURVE ( )  B_SPLINE_CURVE ( 2, ( #9271, #26676, #24101, #7268, #2592, #15387, #4579, #22254, #17967 ),
 .UNSPECIFIED., .F., .F. ) 
 B_SPLINE_CURVE_WITH_KNOTS ( ( 3, 2, 2, 2, 3 ),
 ( 0.3500000000000003109, 0.3750000000000003331, 0.4000000000000003553, 0.4250000000000003775, 0.4500000000000003997 ),
 .UNSPECIFIED. ) 
 CURVE ( )  GEOMETRIC_REPRESENTATION_ITEM ( )  RATIONAL_B_SPLINE_CURVE ( ( 0.9999999999999990008, 0.9238795325112877377, 1.000000000000000000, 0.9238795325112867385, 1.000000000000000000, 0.9238795325112867385, 1.000000000000000000, 0.9238795325112855172, 1.000000000000001110 ) ) 
 REPRESENTATION_ITEM ( '' )  );
#21505=CARTESIAN_POINT ( 'NONE',  ( 96.84719886470463734, 93.93749999863440792, 3.152801135295351997 ) ) ;
#21511=CARTESIAN_POINT ( 'NONE',  ( 104.9952793366501709, 116.8754121666685393, -48.07500000273119412 ) ) ;
#21517=CARTESIAN_POINT ( 'NONE',  ( 104.4587341249999781, 95.31249999863440792, -6.938893903907228378E-15 ) ) ;
#21523=CARTESIAN_POINT ( 'NONE',  ( 98.15313185440925281, 91.99999999863439371, 4.458734124999979898 ) ) ;
#21525=VECTOR ( 'NONE', #15858, 1000.000000000000000 ) ;
#21527=LINE ( 'NONE', #7612, #3858 ) ;
#21539=CARTESIAN_POINT ( 'NONE',  ( 99.99999999999998579, 102.6397644303321215, -51.50000000000000711 ) ) ;
#21550=LINE ( 'NONE', #2024, #25797 ) ;
#21553=CARTESIAN_POINT ( 'NONE',  ( 108.0825317500000011, 112.6261737610028320, -52.02500000273118985 ) ) ;
#21562=CARTESIAN_POINT ( 'NONE',  ( 94.99999999999998579, 110.0000000000000000, 15.00099999999999412 ) ) ;
#21564=CYLINDRICAL_SURFACE ( 'NONE', #14749, 7.000000000000006217 ) ;
#21572=CARTESIAN_POINT ( 'NONE',  ( 97.83688103937537051, 103.3426043859339103, -47.60000000000000142 ) ) ;
#21574=CARTESIAN_POINT ( 'NONE',  ( 98.53841926354351699, 123.2500000010924737, 1.461580736456455920 ) ) ;
#21579=VERTEX_POINT ( 'NONE', #4180 ) ;
#21587=CARTESIAN_POINT ( 'NONE',  ( 102.1829110464049535, 123.0000000000000284, 1.262593708336817500 ) ) ;
#21588=PLANE ( 'NONE',  #6823 ) ;
#21605=CARTESIAN_POINT ( 'NONE',  ( 98.96446609406724804, 124.8499999999999943, -2.500000000000008438 ) ) ;
#21608=CARTESIAN_POINT ( 'NONE',  ( 101.7677669529663547, 124.0000000021849615, -1.767766952966370209 ) ) ;
#21611=ORIENTED_EDGE ( 'NONE', *, *, #25541, .T. ) ;
#21615=PLANE ( 'NONE',  #11148 ) ;
#21619=FACE_OUTER_BOUND ( 'NONE', #19046, .T. ) ;
#21622=CARTESIAN_POINT ( 'NONE',  ( 108.0825317500000011, 107.3738262389971538, -52.22500000273118559 ) ) ;
#21630=ORIENTED_EDGE ( 'NONE', *, *, #5170, .T. ) ;
#21648=DIRECTION ( 'NONE',  ( -0.000000000000000000, 1.000000000000000000, -0.000000000000000000 ) ) ;
#21655=CARTESIAN_POINT ( 'NONE',  ( 91.91746824999999887, 110.0000000000000000, -47.37500000273119838 ) ) ;
#21659=CARTESIAN_POINT ( 'NONE',  ( 107.0000000000000142, 107.7255621263696526, -45.60000000546237686 ) ) ;
#21660=CARTESIAN_POINT ( 'NONE',  ( 98.15313185440925281, 91.62499999863440792, -4.458734124999994997 ) ) ;
#21663=CARTESIAN_POINT ( 'NONE',  ( 94.33688103937537051, 105.8855032339526758, -45.80000000000000426 ) ) ;
#21664=B_SPLINE_CURVE_WITH_KNOTS ( 'NONE', 3,
 ( #1512, #23443, #12579, #10454 ),
 .UNSPECIFIED., .F., .F.,
 ( 4, 4 ),
 ( 0.000000000000000000, 1.000000000000000000 ),
 .UNSPECIFIED. ) ;
#21667=VECTOR ( 'NONE', #25685, 1000.000000000000000 ) ;
#21668=CARTESIAN_POINT ( 'NONE',  ( 104.9999999999999716, 90.06249999999998579, -2.071067811865478170 ) ) ;
#21676=EDGE_CURVE ( 'NONE', #1287, #24831, #255, .T. ) ;
#21677=ORIENTED_EDGE ( 'NONE', *, *, #7569, .T. ) ;
#21690=CARTESIAN_POINT ( 'NONE',  ( 97.71650635000000307, 124.4250000016387219, -9.540979117872439019E-15 ) ) ;
#21693=CARTESIAN_POINT ( 'NONE',  ( 114.9999999999999858, 95.00000000000000000, -15.00000000000000711 ) ) ;
#21695=CARTESIAN_POINT ( 'NONE',  ( 106.5389055433251002, 114.7507929638356785, -53.92500000273119554 ) ) ;
#21696=CARTESIAN_POINT ( 'NONE',  ( 101.0355339059327093, 123.6500000000000057, 2.499999999999984457 ) ) ;
#21706=EDGE_CURVE ( 'NONE', #2910, #2056, #22384, .T. ) ;
#21709=ORIENTED_EDGE ( 'NONE', *, *, #24980, .T. ) ;
#21715=CARTESIAN_POINT ( 'NONE',  ( 104.3262379212492590, 104.0454443415356991, -53.29999999999999716 ) ) ;
#21717=CARTESIAN_POINT ( 'NONE',  ( 100.8561741729129153, 123.7000000010924765, -2.066987299999999195 ) ) ;
#21721=CARTESIAN_POINT ( 'NONE',  ( 95.00000000000000000, 92.37499999726880162, -7.551217303480904118E-15 ) ) ;
#21727=ORIENTED_EDGE ( 'NONE', *, *, #21676, .F. ) ;
#21737=CARTESIAN_POINT ( 'NONE',  ( 93.00000000000000000, 110.0000000000000000, -50.00000000000000711 ) ) ;
#21756=CARTESIAN_POINT ( 'NONE',  ( 97.50000000000000000, 122.7000000021849502, -9.540979117872439019E-15 ) ) ;
#21757=CARTESIAN_POINT ( 'NONE',  ( 99.99999999999998579, 110.0000000000000000, -45.00000000000000711 ) ) ;
#21761=CARTESIAN_POINT ( 'NONE',  ( 100.8561741729129295, 123.2000000010924765, 2.066987299999979211 ) ) ;
#21768=CARTESIAN_POINT ( 'NONE',  ( 95.00472066334982912, 103.1245878333314323, -52.82500000273118701 ) ) ;
#21771=LINE ( 'NONE', #2249, #3136 ) ;
#21780=ORIENTED_EDGE ( 'NONE', *, *, #19238, .T. ) ;
#21789=CARTESIAN_POINT ( 'NONE',  ( 98.96446609406726225, 122.8500000021849416, 2.499999999999977796 ) ) ;
#21798=CARTESIAN_POINT ( 'NONE',  ( 99.99999999999998579, 118.4984768113314146, -47.87500000273119127 ) ) ;
#21803=DIRECTION ( 'NONE',  ( -0.000000000000000000, 1.000000000000000000, -0.000000000000000000 ) ) ;
#21804=CARTESIAN_POINT ( 'NONE',  ( 103.1528011352953484, 94.43749999863440792, -3.152801135295366208 ) ) ;
#21814=CARTESIAN_POINT ( 'NONE',  ( 104.4587341249999923, 93.24999999863439371, 1.846868145590726318 ) ) ;
#21815=CARTESIAN_POINT ( 'NONE',  ( 103.1528011352953484, 95.43749999863440792, 3.152801135295352886 ) ) ;
#21839=CARTESIAN_POINT ( 'NONE',  ( 108.0825317500000153, 110.0000000000000000, -54.12500000273119838 ) ) ;
#21848=CARTESIAN_POINT ( 'NONE',  ( 100.0000000000000000, 110.0000000000000000, -55.00000000000000711 ) ) ;
#21856=CARTESIAN_POINT ( 'NONE',  ( 93.00000000000001421, 107.7255621263696668, -49.89999999999999858 ) ) ;
#21858=CARTESIAN_POINT ( 'NONE',  ( 103.5355339059327235, 92.74999999726881583, 3.535533905932724874 ) ) ;
#21861=ADVANCED_FACE ( 'NONE', ( #20770 ), #16345, .T. ) ;
#21862=CARTESIAN_POINT ( 'NONE',  ( 96.46446609406726225, 95.24999999726881583, -3.535533905932738197 ) ) ;
#21866=ORIENTED_EDGE ( 'NONE', *, *, #19253, .T. ) ;
#21889=EDGE_CURVE ( 'NONE', #25660, #24967, #16234, .T. ) ;
#21891=ORIENTED_EDGE ( 'NONE', *, *, #17322, .F. ) ;
#21898=LINE ( 'NONE', #23879, #19002 ) ;
#21902=VECTOR ( 'NONE', #16870, 1000.000000000000000 ) ;
#21905=CARTESIAN_POINT ( 'NONE',  ( 98.53841926354351699, 123.8500000010924680, 1.461580736456455920 ) ) ;
#21912=CARTESIAN_POINT ( 'NONE',  ( 95.00472066334982912, 103.1245878333314323, -48.82500000273118701 ) ) ;
#21914=CARTESIAN_POINT ( 'NONE',  ( 107.5412658750000077, 110.0000000000000000, -54.68750000136559919 ) ) ;
#21925=PLANE ( 'NONE',  #689 ) ;
#21930=DIRECTION ( 'NONE',  ( -0.000000000000000000, 1.000000000000000000, -0.000000000000000000 ) ) ;
#21941=CARTESIAN_POINT ( 'NONE',  ( 91.91746824999998466, 112.6261737610028320, -45.47500000273119980 ) ) ;
#21945=CARTESIAN_POINT ( 'NONE',  ( 97.49603539231829075, 123.0000000000000000, 0.01993142876900604391 ) ) ;
#21952=CARTESIAN_POINT ( 'NONE',  ( 102.0710678118654613, 90.18749999999998579, -4.999999999999997335 ) ) ;
#21966=CARTESIAN_POINT ( 'NONE',  ( 99.99999999999998579, 110.0000000000000000, -43.00000000000000000 ) ) ;
#21975=CARTESIAN_POINT ( 'NONE',  ( 106.5389055433251002, 114.7507929638356785, -49.92500000273119554 ) ) ;
#21982=CARTESIAN_POINT ( 'NONE',  ( 105.6631189606246295, 114.1144967660473242, -51.30000000546237970 ) ) ;
#21989=EDGE_CURVE ( 'NONE', #19945, #12986, #24545, .T. ) ;
#21991=CARTESIAN_POINT ( 'NONE',  ( 107.0000000000000142, 110.0000000000000000, -53.00000000000000711 ) ) ;
#21993=CARTESIAN_POINT ( 'NONE',  ( 102.4999999999999858, 124.6000000000000085, -9.847140817659276890E-15 ) ) ;
#21997=CARTESIAN_POINT ( 'NONE',  ( 96.46446609406726225, 94.24999999726881583, -3.535533905932738197 ) ) ;
#22000=EDGE_LOOP ( 'NONE', ( #27986, #7027, #2672, #24187, #24468, #10726, #20748, #6583, #10391 ) ) ;
#22010=DIRECTION ( 'NONE',  ( 0.000000000000000000, -1.000000000000000000, 3.469446951953611231E-16 ) ) ;
#22012=CARTESIAN_POINT ( 'NONE',  ( 99.99999999999998579, 102.6397644303321215, -49.50000000000000711 ) ) ;
#22031=CARTESIAN_POINT ( 'NONE',  ( 99.99999999999998579, 123.3000000021849587, -2.499999999999997780 ) ) ;
#22037=CARTESIAN_POINT ( 'NONE',  ( 98.96446609406727646, 122.5500000021849587, -2.499999999999997780 ) ) ;
#22042=DIRECTION ( 'NONE',  ( -5.782411586589357392E-17, 0.000000000000000000, -1.000000000000000000 ) ) ;
#22045=CARTESIAN_POINT ( 'NONE',  ( 102.4976396683250925, 102.3130555110000159, -52.52500000273119696 ) ) ;
#22068=ADVANCED_FACE ( 'NONE', ( #28020 ), #10750, .F. ) ;
#22080=CARTESIAN_POINT ( 'NONE',  ( 108.0825317500000011, 112.6261737610028320, -46.27500000273120406 ) ) ;
#22084=CARTESIAN_POINT ( 'NONE',  ( 98.94657102337468757, 123.0000000000000284, -2.271811130025750192 ) ) ;
#22088=ORIENTED_EDGE ( 'NONE', *, *, #21145, .T. ) ;
#22093=CARTESIAN_POINT ( 'NONE',  ( 104.4587341249999781, 93.31249999863440792, -6.938893903907228378E-15 ) ) ;
#22094=CARTESIAN_POINT ( 'NONE',  ( 98.15313185440925281, 94.87499999863440792, -4.458734124999994997 ) ) ;
#22116=CARTESIAN_POINT ( 'NONE',  ( 91.91746824999998466, 107.3738262389971538, -47.02500000273118275 ) ) ;
#22117=CARTESIAN_POINT ( 'NONE',  ( 102.4999999999999858, 123.7500000000000142, 1.035533905932722876 ) ) ;
#22123=ORIENTED_EDGE ( 'NONE', *, *, #7781, .T. ) ;
#22125=CARTESIAN_POINT ( 'NONE',  ( 97.93301270000000613, 122.9000000010924794, -0.8561741729129506151 ) ) ;
#22128=ORIENTED_EDGE ( 'NONE', *, *, #4796, .T. ) ;
#22132=CARTESIAN_POINT ( 'NONE',  ( 94.33688103937537051, 114.1144967660473242, -46.20000000000000284 ) ) ;
#22135=CARTESIAN_POINT ( 'NONE',  ( 98.23223304703363112, 123.5000000000000000, 1.767766952966351557 ) ) ;
#22138=CARTESIAN_POINT ( 'NONE',  ( 104.9999999999999716, 92.93749999726880162, -2.071067811865478170 ) ) ;
#22147=CYLINDRICAL_SURFACE ( 'NONE', #18056, 4.999999999999989342 ) ;
#22148=CARTESIAN_POINT ( 'NONE',  ( 112.9999999999999858, 95.00000000000000000, 12.99999999999999289 ) ) ;
#22154=VECTOR ( 'NONE', #1281, 1000.000000000000000 ) ;
#22155=CARTESIAN_POINT ( 'NONE',  ( 95.54126587500000767, 91.06249999863440792, -7.484931351350258973E-15 ) ) ;
#22161=ORIENTED_EDGE ( 'NONE', *, *, #23487, .F. ) ;
#22178=CARTESIAN_POINT ( 'NONE',  ( 102.4999999999999716, 123.1500000021849672, -1.035533905932742638 ) ) ;
#22185=CARTESIAN_POINT ( 'NONE',  ( 106.5389055433251002, 105.2492070361643215, -44.32500000273119412 ) ) ;
#22191=VERTEX_POINT ( 'NONE', #761 ) ;
#22210=CARTESIAN_POINT ( 'NONE',  ( 95.00000000000000000, 94.31249999726880162, -2.071067811865479058 ) ) ;
#22224=CARTESIAN_POINT ( 'NONE',  ( 99.08087592991887504, 123.0000000000000426, -2.329274081706632415 ) ) ;
#22225=ORIENTED_EDGE ( 'NONE', *, *, #5935, .T. ) ;
#22231=CARTESIAN_POINT ( 'NONE',  ( 95.67376207875072680, 115.9545556584642867, -50.30000000000000426 ) ) ;
#22232=CARTESIAN_POINT ( 'NONE',  ( 87.00000000000000000, 102.0000000000000000, -43.00000000000000000 ) ) ;
#22234=CARTESIAN_POINT ( 'NONE',  ( 102.0710678118654613, 91.81250000000000000, 4.999999999999983125 ) ) ;
#22235=CARTESIAN_POINT ( 'NONE',  ( 96.84719886470463734, 94.93749999863440792, -3.152801135295366208 ) ) ;
#22254=CARTESIAN_POINT ( 'NONE',  ( 102.0710678118654329, 92.18749999999998579, -5.000000000000023093 ) ) ;
#22260=CARTESIAN_POINT ( 'NONE',  ( 108.0825317500000011, 112.6261737610028320, -48.02500000273118985 ) ) ;
#22262=CARTESIAN_POINT ( 'NONE',  ( 95.54126587500000767, 91.06249999863440792, -7.484931351350258973E-15 ) ) ;
#22271=CARTESIAN_POINT ( 'NONE',  ( 98.96446609406724804, 123.3500000021849274, -2.499999999999996447 ) ) ;
#22278=CARTESIAN_POINT ( 'NONE',  ( 97.50236033167492167, 117.6869444889999841, -53.77500000273119696 ) ) ;
#22280=CARTESIAN_POINT ( 'NONE',  ( 98.23223304703363112, 124.8999999999999915, -1.767766952966370209 ) ) ;
#22284=CARTESIAN_POINT ( 'NONE',  ( 99.99999999999998579, 94.62499999726881583, 4.999999999999984013 ) ) ;
#22287=CARTESIAN_POINT ( 'NONE',  ( 95.00472066334981491, 116.8754121666685393, -49.67500000273119554 ) ) ;
#22297=CARTESIAN_POINT ( 'NONE',  ( 95.54126587499999346, 91.12499999863439371, 1.846868145590722543 ) ) ;
#22307=VECTOR ( 'NONE', #12861, 1000.000000000000000 ) ;
#22314=CARTESIAN_POINT ( 'NONE',  ( 108.0825317500000153, 110.0000000000000000, -50.12500000273119127 ) ) ;
#22315=ADVANCED_FACE ( 'NONE', ( #11987 ), #7294, .F. ) ;
#22317=LINE ( 'NONE', #7182, #516 ) ;
#22323=CARTESIAN_POINT ( 'NONE',  ( 99.99999999999998579, 123.1500000010924794, 2.066987299999980099 ) ) ;
#22329=CARTESIAN_POINT ( 'NONE',  ( 98.15313185440925281, 92.99999999863439371, 4.458734124999979898 ) ) ;
#22330=CARTESIAN_POINT ( 'NONE',  ( 108.0825317500000011, 107.3738262389971538, -46.22500000273118559 ) ) ;
#22335=CARTESIAN_POINT ( 'NONE',  ( 104.9999999999999858, 90.87499999726880162, -6.938893903907228378E-15 ) ) ;
#22344=DIRECTION ( 'NONE',  ( 1.000000000000000000, 0.000000000000000000, 0.000000000000000000 ) ) ;
#22352=DIRECTION ( 'NONE',  ( -0.000000000000000000, 1.000000000000000000, -0.000000000000000000 ) ) ;
#22363=CARTESIAN_POINT ( 'NONE',  ( 97.50236033167492167, 102.3130555110000159, -52.97500000273119980 ) ) ;
#22366=FACE_OUTER_BOUND ( 'NONE', #14404, .T. ) ;
#22370=CARTESIAN_POINT ( 'NONE',  ( 106.9999999999999858, 112.2744378736303617, -50.90000000000000568 ) ) ;
#22373=CARTESIAN_POINT ( 'NONE',  ( 104.9999999999999858, 92.00000000000000000, -6.938893903907228378E-15 ) ) ;
#22384=( BOUNDED_CURVE ( )  B_SPLINE_CURVE ( 2, ( #4676, #26914, #7359, #18055, #544, #26771, #15633, #13338, #2543 ),
 .UNSPECIFIED., .F., .F. ) 
 B_SPLINE_CURVE_WITH_KNOTS ( ( 3, 2, 2, 2, 3 ),
 ( 0.08333333333333307891, 0.1249999999999999167, 0.1666666666666667407, 0.2083333333333335924, 0.2500000000000004441 ),
 .UNSPECIFIED. ) 
 CURVE ( )  GEOMETRIC_REPRESENTATION_ITEM ( )  RATIONAL_B_SPLINE_CURVE ( ( 1.000000000000000444, 0.9238795325112862944, 1.000000000000000000, 0.9238795325112867385, 1.000000000000000000, 0.9238795325112867385, 1.000000000000000000, 0.9238795325112859613, 1.000000000000000888 ) ) 
 REPRESENTATION_ITEM ( '' )  );
#22399=CARTESIAN_POINT ( 'NONE',  ( 97.50236033167492167, 102.3130555110000159, -48.72500000273119269 ) ) ;
#22400=CARTESIAN_POINT ( 'NONE',  ( 104.4587341249999781, 92.56249999863440792, -6.938893903907228378E-15 ) ) ;
#22407=DIRECTION ( 'NONE',  ( -1.224646799147411139E-16, 0.000000000000000000, -1.000000000000000000 ) ) ;
#22408=CARTESIAN_POINT ( 'NONE',  ( 97.50000000000000000, 123.5500000021849587, 1.035533905932725096 ) ) ;
#22415=CARTESIAN_POINT ( 'NONE',  ( 107.0000000000000142, 107.7255621263696526, -45.10000000000001563 ) ) ;
#22417=CARTESIAN_POINT ( 'NONE',  ( 102.4999999999999858, 123.7999999999999972, -9.847140817659276890E-15 ) ) ;
#22422=CARTESIAN_POINT ( 'NONE',  ( 104.4587341249999781, 90.56249999863440792, -6.938893903907228378E-15 ) ) ;
#22424=CARTESIAN_POINT ( 'NONE',  ( 104.9952793366501709, 103.1245878333314465, -48.67500000273120264 ) ) ;
#22425=EDGE_CURVE ( 'NONE', #27429, #4858, #4413, .T. ) ;
#22428=CARTESIAN_POINT ( 'NONE',  ( 102.4999999999999858, 123.0500000021849587, 1.035533905932722876 ) ) ;
#22435=DIRECTION ( 'NONE',  ( 1.000000000000000000, -0.000000000000000000, -5.782411586589357392E-17 ) ) ;
#22443=ORIENTED_EDGE ( 'NONE', *, *, #25389, .T. ) ;
#22450=ORIENTED_EDGE ( 'NONE', *, *, #23604, .F. ) ;
#22454=LINE ( 'NONE', #5208, #10390 ) ;
#22457=CARTESIAN_POINT ( 'NONE',  ( 108.0825317500000011, 107.3738262389971680, -46.22500000273118559 ) ) ;
#22471=CARTESIAN_POINT ( 'NONE',  ( 104.9999999999999858, 91.87499999726880162, -6.938893903907228378E-15 ) ) ;
#22472=CARTESIAN_POINT ( 'NONE',  ( 108.0825317500000011, 112.6261737610028320, -46.02500000273120406 ) ) ;
#22476=CARTESIAN_POINT ( 'NONE',  ( 99.99999999999998579, 91.12499999726880162, -4.999999999999997335 ) ) ;
#22496=FACE_OUTER_BOUND ( 'NONE', #3441, .T. ) ;
#22506=CARTESIAN_POINT ( 'NONE',  ( 97.50236033167492167, 117.6869444889999841, -51.77500000273119696 ) ) ;
#22507=CARTESIAN_POINT ( 'NONE',  ( 98.49227936199515909, 122.9999999999999858, 1.999863547705611477 ) ) ;
#22509=CARTESIAN_POINT ( 'NONE',  ( 98.53841926354351699, 123.0500000010924850, 1.461580736456455920 ) ) ;
#22518=CARTESIAN_POINT ( 'NONE',  ( 97.92893218813452449, 92.68749999999998579, 4.999999999999983125 ) ) ;
#22531=DIRECTION ( 'NONE',  ( 1.000000000000000000, 0.000000000000000000, 0.000000000000000000 ) ) ;
#22534=DIRECTION ( 'NONE',  ( 1.000000000000000000, 0.000000000000000000, -5.782411586589357392E-17 ) ) ;
#22543=CARTESIAN_POINT ( 'NONE',  ( 93.46109445667491400, 114.7507929638356785, -47.32500000273119412 ) ) ;
#22544=CARTESIAN_POINT ( 'NONE',  ( 98.96446609406724804, 124.1500000021849672, -2.499999999999992450 ) ) ;
#22552=CARTESIAN_POINT ( 'NONE',  ( 99.99999999999998579, 90.00000000000000000, -4.999999999999996447 ) ) ;
#22560=CARTESIAN_POINT ( 'NONE',  ( 93.00000000000001421, 107.7255621263696668, -45.89999999999999858 ) ) ;
#22568=CARTESIAN_POINT ( 'NONE',  ( 99.99999999999998579, 94.31249999863440792, 4.458734124999981674 ) ) ;
#22570=AXIS2_PLACEMENT_3D ( 'NONE', #13909, #9506, #546 ) ;
#22572=CARTESIAN_POINT ( 'NONE',  ( 93.46109445667491400, 105.2492070361643215, -53.17500000273119554 ) ) ;
#22577=CARTESIAN_POINT ( 'NONE',  ( 102.4999999999999858, 124.5500000000000256, 1.035533905932722876 ) ) ;
#22579=ORIENTED_EDGE ( 'NONE', *, *, #18755, .T. ) ;
#22594=EDGE_CURVE ( 'NONE', #15224, #6173, #3837, .T. ) ;
#22601=CARTESIAN_POINT ( 'NONE',  ( 93.46109445667491400, 114.7507929638356785, -49.32500000273120122 ) ) ;
#22616=CARTESIAN_POINT ( 'NONE',  ( 95.00472066334982912, 103.1245878333314323, -46.82500000273118701 ) ) ;
#22618=CARTESIAN_POINT ( 'NONE',  ( 99.99999999999998579, 90.00000000000000000, -6.938893903907228378E-15 ) ) ;
#22623=CARTESIAN_POINT ( 'NONE',  ( 99.99999999999998579, 94.12499999726881583, -4.999999999999997335 ) ) ;
#22640=CARTESIAN_POINT ( 'NONE',  ( 101.7677669529663547, 123.9069999999781402, -1.767766952966370209 ) ) ;
#22652=LINE ( 'NONE', #11789, #22900 ) ;
#22654=CARTESIAN_POINT ( 'NONE',  ( 97.92893218813453871, 90.31249999999998579, -4.999999999999994671 ) ) ;
#22656=ORIENTED_EDGE ( 'NONE', *, *, #11709, .F. ) ;
#22664=CARTESIAN_POINT ( 'NONE',  ( 99.99999999999998579, 90.75000000000000000, 4.999999999999984013 ) ) ;
#22678=CARTESIAN_POINT ( 'NONE',  ( 107.0000000000000142, 110.0000000000000000, -44.25000000273119127 ) ) ;
#22688=CARTESIAN_POINT ( 'NONE',  ( 95.00472066334982912, 103.1245878333314323, -44.82500000273117990 ) ) ;
#22695=LINE ( 'NONE', #16408, #12259 ) ;
#22700=ORIENTED_EDGE ( 'NONE', *, *, #7569, .F. ) ;
#22704=CARTESIAN_POINT ( 'NONE',  ( 95.67376207875072680, 115.9545556584642867, -46.30000000000001137 ) ) ;
#22711=CARTESIAN_POINT ( 'NONE',  ( 101.8468681455907330, 93.74999999863439371, -4.458734124999994997 ) ) ;
#22713=CARTESIAN_POINT ( 'NONE',  ( 95.00472066334981491, 116.8754121666685393, -51.67500000273118843 ) ) ;
#22719=( BOUNDED_CURVE ( )  B_SPLINE_CURVE ( 2, ( #24812, #22830, #7560, #9838, #5296, #27523, #13817, #20963, #23104 ),
 .UNSPECIFIED., .F., .F. ) 
 B_SPLINE_CURVE_WITH_KNOTS ( ( 3, 2, 2, 2, 3 ),
 ( 0.5833333333333337034, 0.6250000000000002220, 0.6666666666666667407, 0.7083333333333332593, 0.7499999999999997780 ),
 .UNSPECIFIED. ) 
 CURVE ( )  GEOMETRIC_REPRESENTATION_ITEM ( )  RATIONAL_B_SPLINE_CURVE ( ( 0.9999999999999994449, 0.9238795325112872936, 1.000000000000000000, 0.9238795325112867385, 1.000000000000000000, 0.9238795325112867385, 1.000000000000000000, 0.9238795325112871826, 0.9999999999999995559 ) ) 
 REPRESENTATION_ITEM ( '' )  );
#22722=CARTESIAN_POINT ( 'NONE',  ( 93.00000000000000000, 110.0000000000000000, -50.00000000000000711 ) ) ;
#22732=ORIENTED_EDGE ( 'NONE', *, *, #8313, .T. ) ;
#22747=ADVANCED_FACE ( 'NONE', ( #6656 ), #24058, .T. ) ;
#22757=CARTESIAN_POINT ( 'NONE',  ( 104.9999999999999716, 95.81249999726880162, 2.071067811865467956 ) ) ;
#22759=CARTESIAN_POINT ( 'NONE',  ( 104.9952793366501851, 103.1245878333314323, -46.42500000273119554 ) ) ;
#22761=DIRECTION ( 'NONE',  ( 0.000000000000000000, 0.000000000000000000, -1.000000000000000000 ) ) ;
#22763=CARTESIAN_POINT ( 'NONE',  ( 112.9999999999999858, 123.0000000000000000, -13.00000000000001066 ) ) ;
#22775=CARTESIAN_POINT ( 'NONE',  ( 99.99999999999998579, 90.00000000000000000, -6.938893903907228378E-15 ) ) ;
#22784=CARTESIAN_POINT ( 'NONE',  ( 94.33688103937537051, 105.8855032339526758, -47.80000000000001137 ) ) ;
#22796=CARTESIAN_POINT ( 'NONE',  ( 91.91746824999999887, 110.0000000000000000, -53.37500000273119838 ) ) ;
#22804=VECTOR ( 'NONE', #10554, 999.9999999999997726 ) ;
#22807=CARTESIAN_POINT ( 'NONE',  ( 99.99999999999998579, 91.75000000000000000, 4.999999999999984013 ) ) ;
#22830=CARTESIAN_POINT ( 'NONE',  ( 98.96446609406726225, 123.5500000000000114, 2.499999999999972022 ) ) ;
#22833=CARTESIAN_POINT ( 'NONE',  ( 95.67376207875072680, 115.9545556584642867, -48.80000000546237260 ) ) ;
#22834=CARTESIAN_POINT ( 'NONE',  ( 95.54126587499999346, 91.99999999863439371, -1.846868145590737864 ) ) ;
#22836=CARTESIAN_POINT ( 'NONE',  ( 97.93301270000000613, 124.7500000010924737, -9.540979117872439019E-15 ) ) ;
#22838=EDGE_LOOP ( 'NONE', ( #17121, #6912, #8458, #8979, #23695, #25837, #4488, #21109 ) ) ;
#22846=CARTESIAN_POINT ( 'NONE',  ( 102.4976396683250925, 102.3130555110000159, -44.77500000273119696 ) ) ;
#22853=CARTESIAN_POINT ( 'NONE',  ( 104.9999999999999716, 95.81249999726881583, 2.071067811865467956 ) ) ;
#22854=DIRECTION ( 'NONE',  ( -0.000000000000000000, 1.000000000000000000, -0.000000000000000000 ) ) ;
#22858=DIRECTION ( 'NONE',  ( 0.000000000000000000, 0.000000000000000000, 1.000000000000000000 ) ) ;
#22865=CARTESIAN_POINT ( 'NONE',  ( 95.54126587500000767, 94.06249999863440792, -7.484931351350258973E-15 ) ) ;
#22866=DIRECTION ( 'NONE',  ( -1.000000000000000000, 0.000000000000000000, 0.000000000000000000 ) ) ;
#22878=CARTESIAN_POINT ( 'NONE',  ( 97.92893218813453871, 91.18749999726880162, -4.999999999999994671 ) ) ;
#22882=( BOUNDED_CURVE ( )  B_SPLINE_CURVE ( 2, ( #20701, #9712, #3445, #17980, #16265, #9283, #5024, #26689, #7137 ),
 .UNSPECIFIED., .F., .T. ) 
 B_SPLINE_CURVE_WITH_KNOTS ( ( 3, 2, 2, 2, 3 ),
 ( 0.2500000000000002220, 0.2750000000000002442, 0.3000000000000002665, 0.3250000000000002887, 0.3500000000000003109 ),
 .UNSPECIFIED. ) 
 CURVE ( )  GEOMETRIC_REPRESENTATION_ITEM ( )  RATIONAL_B_SPLINE_CURVE ( ( 0.9999999999999993339, 0.9238795325112874046, 1.000000000000000000, 0.9238795325112867385, 1.000000000000000000, 0.9238795325112867385, 1.000000000000000000, 0.9238795325112857393, 1.000000000000001110 ) ) 
 REPRESENTATION_ITEM ( '' )  );
#22887=( NAMED_UNIT ( * ) PLANE_ANGLE_UNIT ( ) SI_UNIT ( $, .RADIAN. ) );
#22899=ORIENTED_EDGE ( 'NONE', *, *, #1003, .T. ) ;
#22900=VECTOR ( 'NONE', #11930, 1000.000000000000000 ) ;
#22910=CARTESIAN_POINT ( 'NONE',  ( 99.99999999999998579, 89.99899999999999523, 2.499999999999985789 ) ) ;
#22918=CARTESIAN_POINT ( 'NONE',  ( 97.50000000000000000, 124.2500000000000000, 1.035533905932725096 ) ) ;
#22919=CARTESIAN_POINT ( 'NONE',  ( 99.99999999999998579, 123.2000000000000028, -2.499999999999997780 ) ) ;
#22926=EDGE_LOOP ( 'NONE', ( #6054, #17815, #3832, #6821 ) ) ;
#22956=EDGE_LOOP ( 'NONE', ( #3059, #16610, #6055, #17755 ) ) ;
#22959=CARTESIAN_POINT ( 'NONE',  ( 99.99999999999998579, 125.0000000000000000, -9.540979117872439019E-15 ) ) ;
#22964=CARTESIAN_POINT ( 'NONE',  ( 95.54126587499999346, 91.87499999863439371, 1.846868145590722543 ) ) ;
#22971=CARTESIAN_POINT ( 'NONE',  ( 97.83688103937538472, 116.6573956140660897, -46.90000000546238113 ) ) ;
#22972=CARTESIAN_POINT ( 'NONE',  ( 96.84719886470463734, 90.68749999863440792, -3.152801135295366208 ) ) ;
#22976=ORIENTED_EDGE ( 'NONE', *, *, #1318, .T. ) ;
#22984=ORIENTED_EDGE ( 'NONE', *, *, #13303, .T. ) ;
#22985=CARTESIAN_POINT ( 'NONE',  ( 99.99999999999998579, 101.5015231886685854, -48.87500000273119838 ) ) ;
#22990=CARTESIAN_POINT ( 'NONE',  ( 103.1528011352953484, 92.68749999863440792, -3.152801135295366208 ) ) ;
#22999=EDGE_LOOP ( 'NONE', ( #18564, #2610 ) ) ;
#23002=CARTESIAN_POINT ( 'NONE',  ( 104.4587341249999923, 94.62499999863439371, -1.846868145590737198 ) ) ;
#23013=VERTEX_POINT ( 'NONE', #26633 ) ;
#23054=CARTESIAN_POINT ( 'NONE',  ( 98.23223304703363112, 123.2999999999999972, -1.767766952966370209 ) ) ;
#23069=CARTESIAN_POINT ( 'NONE',  ( 104.9952793366501851, 103.1245878333314323, -50.67500000273119554 ) ) ;
#23070=CARTESIAN_POINT ( 'NONE',  ( 104.9999999999999716, 93.93750000000000000, 2.071067811865467956 ) ) ;
#23072=CARTESIAN_POINT ( 'NONE',  ( 97.93301269999999192, 123.9000000010924794, -0.8561741729129505041 ) ) ;
#23097=CARTESIAN_POINT ( 'NONE',  ( 99.99999999999998579, 95.06249999863440792, 4.458734124999981674 ) ) ;
#23104=CARTESIAN_POINT ( 'NONE',  ( 99.99999999999998579, 123.2000000000000028, -2.499999999999997780 ) ) ;
#23106=CARTESIAN_POINT ( 'NONE',  ( 93.00000000000000000, 110.0000000000000000, -46.50000000546238255 ) ) ;
#23107=CARTESIAN_POINT ( 'NONE',  ( 104.4587341249999781, 90.31249999863440792, -6.938893903907228378E-15 ) ) ;
#23114=CLOSED_SHELL ( 'NONE', ( #22068, #3207, #27117, #12295, #4388, #20843, #26737, #2013, #3220, #13096, #22315, #7449, #11032, #15086, #14534, #12416, #7766, #22747, #15575, #9347, #12426, #18410, #16492, #18024, #11737, #2534, #14036, #9946, #13313, #15941, #24645, #1251, #25519, #12023, #3242, #1846, #19068, #12304, #17520, #9679, #21861, #15211, #10532, #21183, #14853, #13847, #14161, #11240, #27126, #5184, #9296, #26734, #3981, #4273, #2579, #18684, #9635, #13487, #7222, #26557, #9499, #6577, #1349, #5309, #13040, #23972, #5662, #13983, #3908, #7256, #26130, #24595, #3635, #15406, #19732, #6623, #11547 ) ) ;
#23122=CARTESIAN_POINT ( 'NONE',  ( 93.46109445667491400, 105.2492070361643215, -45.17500000273119554 ) ) ;
#23126=CARTESIAN_POINT ( 'NONE',  ( 91.91746824999999887, 110.0000000000000000, -45.12500000273119838 ) ) ;
#23142=FACE_OUTER_BOUND ( 'NONE', #27709, .T. ) ;
#23143=CARTESIAN_POINT ( 'NONE',  ( 98.15313185440923860, 93.24999999863439371, 4.458734124999980786 ) ) ;
#23162=B_SPLINE_CURVE_WITH_KNOTS ( 'NONE', 3,
 ( #21449, #14590, #21587, #19013, #17010, #23169 ),
 .UNSPECIFIED., .F., .F.,
 ( 4, 2, 4 ),
 ( 0.6250000000000000000, 0.6875000000000000000, 0.7500000000000000000 ),
 .UNSPECIFIED. ) ;
#23169=CARTESIAN_POINT ( 'NONE',  ( 102.4999999999999858, 123.0000000000000000, -8.724596124144689908E-15 ) ) ;
#23196=CARTESIAN_POINT ( 'NONE',  ( 101.0355339059327378, 123.1569999999781402, -2.499999999999997780 ) ) ;
#23197=AXIS2_PLACEMENT_3D ( 'NONE', #3012, #9138, #6992 ) ;
#23210=CARTESIAN_POINT ( 'NONE',  ( 102.4976396683250925, 117.6869444889999841, -47.97500000273119269 ) ) ;
#23211=CARTESIAN_POINT ( 'NONE',  ( 104.9999999999999858, 94.00000000000000000, -6.938893903907228378E-15 ) ) ;
#23213=CARTESIAN_POINT ( 'NONE',  ( 99.99999999999998579, 89.99899999999999523, -9.540979117872439019E-15 ) ) ;
#23227=CARTESIAN_POINT ( 'NONE',  ( 93.00000000000002842, 112.2744378736303474, -46.60000000546238397 ) ) ;
#23235=CARTESIAN_POINT ( 'NONE',  ( 99.99999999999998579, 101.5015231886685712, -52.87500000273119838 ) ) ;
#23238=SHAPE_DEFINITION_REPRESENTATION ( #18102, #26810 ) ;
#23243=CARTESIAN_POINT ( 'NONE',  ( 94.33688103937537051, 114.1144967660473242, -50.70000000546238539 ) ) ;
#23244=CARTESIAN_POINT ( 'NONE',  ( 99.99999999999998579, 94.31249999863440792, 4.458734124999981674 ) ) ;
#23252=CARTESIAN_POINT ( 'NONE',  ( 104.4587341249999923, 91.37499999863439371, -1.846868145590737198 ) ) ;
#23256=CYLINDRICAL_SURFACE ( 'NONE', #9502, 2.999999999999989786 ) ;
#23260=CARTESIAN_POINT ( 'NONE',  ( 104.9952793366501851, 103.1245878333314323, -46.67500000273118843 ) ) ;
#23265=CARTESIAN_POINT ( 'NONE',  ( 93.46109445667491400, 105.2492070361643215, -48.92500000273119554 ) ) ;
#23270=DIRECTION ( 'NONE',  ( 5.782411586589357392E-17, -0.000000000000000000, 1.000000000000000000 ) ) ;
#23283=CARTESIAN_POINT ( 'NONE',  ( 100.8561741729129437, 124.0000000010925021, 2.066987299999979655 ) ) ;
#23287=CARTESIAN_POINT ( 'NONE',  ( 96.46446609406726225, 93.62500000000000000, 3.535533905932723986 ) ) ;
#23293=CARTESIAN_POINT ( 'NONE',  ( 93.00000000000000000, 110.0000000000000000, -54.00000000000000711 ) ) ;
#23294=EDGE_CURVE ( 'NONE', #5694, #18097, #9791, .T. ) ;
#23297=EDGE_CURVE ( 'NONE', #11152, #8293, #919, .T. ) ;
#23307=CARTESIAN_POINT ( 'NONE',  ( 99.99999999999998579, 92.62499999726881583, 4.999999999999984013 ) ) ;
#23308=CARTESIAN_POINT ( 'NONE',  ( 107.0000000000000284, 107.7255621263696952, -51.60000000546238397 ) ) ;
#23309=DIRECTION ( 'NONE',  ( -5.782411586589357392E-17, 0.000000000000000000, -1.000000000000000000 ) ) ;
#23311=CARTESIAN_POINT ( 'NONE',  ( 102.2113248666666436, 122.8333333340616491, -9.811788309856265935E-15 ) ) ;
#23315=EDGE_LOOP ( 'NONE', ( #16195, #12013, #13153, #19155 ) ) ;
#23326=CARTESIAN_POINT ( 'NONE',  ( 97.50000000000000000, 125.0000000000000000, -9.540979117872439019E-15 ) ) ;
#23329=CARTESIAN_POINT ( 'NONE',  ( 97.50000000000000000, 123.3999999999999915, -9.540979117872439019E-15 ) ) ;
#23331=CARTESIAN_POINT ( 'NONE',  ( 101.4615807364564546, 124.2500000010924737, 1.461580736456455476 ) ) ;
#23345=CARTESIAN_POINT ( 'NONE',  ( 93.46109445667491400, 114.7507929638356785, -49.57500000273120122 ) ) ;
#23347=CARTESIAN_POINT ( 'NONE',  ( 102.0669872999999939, 123.6000000010924680, -0.8561741729129507261 ) ) ;
#23360=AXIS2_PLACEMENT_3D ( 'NONE', #23413, #25127, #10277 ) ;
#23362=CARTESIAN_POINT ( 'NONE',  ( 107.0000000000000142, 110.0000000000000000, -53.00000000000000711 ) ) ;
#23369=CARTESIAN_POINT ( 'NONE',  ( 103.1528011352953484, 93.43749999863440792, -3.152801135295366208 ) ) ;
#23379=CARTESIAN_POINT ( 'NONE',  ( 105.6631189606246295, 114.1144967660473242, -49.30000000546237970 ) ) ;
#23380=CARTESIAN_POINT ( 'NONE',  ( 95.54126587500000767, 95.06249999863440792, -7.484931351350258973E-15 ) ) ;
#23387=CARTESIAN_POINT ( 'NONE',  ( 95.54126587499999346, 90.74999999863439371, -1.846868145590737864 ) ) ;
#23398=CARTESIAN_POINT ( 'NONE',  ( 106.5389055433251002, 105.2492070361643215, -44.32500000273119412 ) ) ;
#23413=CARTESIAN_POINT ( 'NONE',  ( 100.0000000000000000, 110.0000000000000000, -55.00000000000000711 ) ) ;
#23418=CARTESIAN_POINT ( 'NONE',  ( 95.54126587499999346, 93.99999999863439371, -1.846868145590737864 ) ) ;
#23425=EDGE_CURVE ( 'NONE', #14663, #24847, #14886, .T. ) ;
#23428=CARTESIAN_POINT ( 'NONE',  ( 95.00000000000000000, 92.50000000000000000, -7.551217303480904118E-15 ) ) ;
#23430=CARTESIAN_POINT ( 'NONE',  ( 84.99999999999998579, 97.00000000000000000, 14.99999999999999467 ) ) ;
#23431=CARTESIAN_POINT ( 'NONE',  ( 98.53841926354351699, 124.0500000010924708, 1.461580736456455920 ) ) ;
#23434=CARTESIAN_POINT ( 'NONE',  ( 87.00000000000000000, 95.00000000000000000, 12.99999999999999467 ) ) ;
#23443=CARTESIAN_POINT ( 'NONE',  ( 102.0669872999999797, 122.6833333344258108, -9.794112055954758880E-15 ) ) ;
#23448=CARTESIAN_POINT ( 'NONE',  ( 102.0710678118654187, 94.06249999726881583, -5.000000000000031974 ) ) ;
#23468=CARTESIAN_POINT ( 'NONE',  ( 97.50000000000000000, 123.3499999999999943, -1.035533905932742416 ) ) ;
#23470=CARTESIAN_POINT ( 'NONE',  ( 102.0669873000000081, 123.6000000010924680, -0.8561741729129508371 ) ) ;
#23481=CARTESIAN_POINT ( 'NONE',  ( 108.0825317500000153, 110.0000000000000000, -50.37500000273119127 ) ) ;
#23487=EDGE_CURVE ( 'NONE', #4009, #22191, #27884, .T. ) ;
#23496=AXIS2_PLACEMENT_3D ( 'NONE', #4702, #27977, #10427 ) ;
#23499=ORIENTED_EDGE ( 'NONE', *, *, #13831, .T. ) ;
#23506=CARTESIAN_POINT ( 'NONE',  ( 99.99999999999998579, 94.56249999863440792, -4.458734124999994997 ) ) ;
#23507=CARTESIAN_POINT ( 'NONE',  ( 107.0000000000000142, 110.0000000000000000, -55.00000000000000711 ) ) ;
#23508=AXIS2_PLACEMENT_3D ( 'NONE', #11710, #3184, #1335 ) ;
#23517=CARTESIAN_POINT ( 'NONE',  ( 104.4587341249999781, 91.31249999863440792, -6.938893903907228378E-15 ) ) ;
#23548=CARTESIAN_POINT ( 'NONE',  ( 91.91746824999999887, 110.0000000000000000, -53.12500000273119838 ) ) ;
#23555=ORIENTED_EDGE ( 'NONE', *, *, #18000, .T. ) ;
#23557=CARTESIAN_POINT ( 'NONE',  ( 99.14382582708708469, 124.4000000010924794, -2.066987299999998751 ) ) ;
#23566=ORIENTED_EDGE ( 'NONE', *, *, #3941, .T. ) ;
#23567=CARTESIAN_POINT ( 'NONE',  ( 95.67376207875072680, 104.0454443415356991, -51.70000000000001705 ) ) ;
#23569=CARTESIAN_POINT ( 'NONE',  ( 101.4615807364564546, 123.6500000010924651, -1.461580736456474794 ) ) ;
#23576=ORIENTED_EDGE ( 'NONE', *, *, #6126, .T. ) ;
#23602=DIRECTION ( 'NONE',  ( 0.000000000000000000, -1.000000000000000000, 0.000000000000000000 ) ) ;
#23603=CARTESIAN_POINT ( 'NONE',  ( 102.4999999999999858, 123.9000000021849530, -9.847140817659276890E-15 ) ) ;
#23604=EDGE_CURVE ( 'NONE', #17147, #24017, #15596, .T. ) ;
#23607=CARTESIAN_POINT ( 'NONE',  ( 97.93301270000000613, 123.1500000010924651, -9.540979117872439019E-15 ) ) ;
#23608=DIRECTION ( 'NONE',  ( 1.000000000000000000, 0.000000000000000000, 0.000000000000000000 ) ) ;
#23611=CARTESIAN_POINT ( 'NONE',  ( 94.33688103937537051, 105.8855032339526758, -48.30000000546237970 ) ) ;
#23613=CARTESIAN_POINT ( 'NONE',  ( 94.33688103937537051, 105.8855032339526758, -53.80000000000000426 ) ) ;
#23621=CARTESIAN_POINT ( 'NONE',  ( 102.4976396683250925, 102.3130555110000159, -50.77500000273119696 ) ) ;
#23622=DIRECTION ( 'NONE',  ( 1.000000000000000000, 0.000000000000000000, 0.000000000000000000 ) ) ;
#23645=CARTESIAN_POINT ( 'NONE',  ( 99.99999999999998579, 122.5000000021849615, -2.499999999999997780 ) ) ;
#23657=CARTESIAN_POINT ( 'NONE',  ( 103.1528011352953484, 92.43749999863440792, -3.152801135295366208 ) ) ;
#23664=CARTESIAN_POINT ( 'NONE',  ( 98.15313185440925281, 90.62499999863439371, -4.458734124999994997 ) ) ;
#23669=ORIENTED_EDGE ( 'NONE', *, *, #15132, .F. ) ;
#23670=CARTESIAN_POINT ( 'NONE',  ( 84.99999999999998579, 100.0000000000000000, -15.00000000000000533 ) ) ;
#23687=FACE_OUTER_BOUND ( 'NONE', #15081, .T. ) ;
#23690=DIRECTION ( 'NONE',  ( 5.782411586589357392E-17, -0.000000000000000000, 1.000000000000000000 ) ) ;
#23695=ORIENTED_EDGE ( 'NONE', *, *, #20668, .F. ) ;
#23698=CARTESIAN_POINT ( 'NONE',  ( 107.0000000000000142, 110.0000000000000000, -54.25000000273119838 ) ) ;
#23706=CARTESIAN_POINT ( 'NONE',  ( 94.33688103937537051, 105.8855032339526758, -47.80000000000001137 ) ) ;
#23710=( BOUNDED_CURVE ( )  B_SPLINE_CURVE ( 2, ( #5395, #14064, #22784, #20643, #3254, #9795, #7661, #16354, #5539, #14202, #10897 ),
 .UNSPECIFIED., .F., .F. ) 
 B_SPLINE_CURVE_WITH_KNOTS ( ( 3, 2, 2, 2, 2, 3 ),
 ( 0.6999999999999998446, 0.7199999999999998623, 0.7399999999999998801, 0.7600000000000000089, 0.7800000000000000266, 0.8000000000000000444 ),
 .UNSPECIFIED. ) 
 CURVE ( )  GEOMETRIC_REPRESENTATION_ITEM ( )  RATIONAL_B_SPLINE_CURVE ( ( 1.000000000000000222, 0.9510565162951533091, 1.000000000000000000, 0.9510565162951535312, 1.000000000000000000, 0.9510565162951535312, 1.000000000000000000, 0.9510565162951535312, 1.000000000000000000, 0.9510565162951535312, 1.000000000000000000 ) ) 
 REPRESENTATION_ITEM ( '' )  );
#23711=CARTESIAN_POINT ( 'NONE',  ( 107.0000000000000142, 107.7255621263696526, -43.60000000546237686 ) ) ;
#23716=ORIENTED_EDGE ( 'NONE', *, *, #19539, .F. ) ;
#23726=DIRECTION ( 'NONE',  ( 0.000000000000000000, 0.000000000000000000, 1.000000000000000000 ) ) ;
#23738=CARTESIAN_POINT ( 'NONE',  ( 94.33688103937537051, 105.8855032339526758, -46.30000000546237970 ) ) ;
#23749=CARTESIAN_POINT ( 'NONE',  ( 108.0825317500000153, 110.0000000000000000, -44.25000000273119838 ) ) ;
#23756=CARTESIAN_POINT ( 'NONE',  ( 104.9952793366501851, 103.1245878333314323, -50.42500000273119554 ) ) ;
#23773=EDGE_CURVE ( 'NONE', #13309, #13582, #26885, .T. ) ;
#23774=CARTESIAN_POINT ( 'NONE',  ( 104.3262379212492590, 115.9545556584642867, -47.20000000546237828 ) ) ;
#23777=CARTESIAN_POINT ( 'NONE',  ( 100.0000000000000000, 110.0000000000000000, -45.00000000000000711 ) ) ;
#23787=CARTESIAN_POINT ( 'NONE',  ( 104.9952793366501709, 103.1245878333314465, -44.67500000273118843 ) ) ;
#23792=CARTESIAN_POINT ( 'NONE',  ( 99.99999999999998579, 94.56249999863440792, -4.458734124999994997 ) ) ;
#23796=ORIENTED_EDGE ( 'NONE', *, *, #26568, .F. ) ;
#23798=CARTESIAN_POINT ( 'NONE',  ( 99.99999999999998579, 92.06249999863440792, 4.458734124999981674 ) ) ;
#23799=VERTEX_POINT ( 'NONE', #26595 ) ;
#23820=CARTESIAN_POINT ( 'NONE',  ( 99.99999999999998579, 90.00000000000000000, 4.999999999999983125 ) ) ;
#23823=CARTESIAN_POINT ( 'NONE',  ( 97.83688103937538472, 116.6573956140660897, -46.40000000000001279 ) ) ;
#23825=CARTESIAN_POINT ( 'NONE',  ( 102.4976396683250925, 117.6869444889999841, -53.72500000273119980 ) ) ;
#23826=CARTESIAN_POINT ( 'NONE',  ( 101.7677669529663547, 123.8999999999999915, -1.767766952966370209 ) ) ;
#23833=CARTESIAN_POINT ( 'NONE',  ( 100.8561741729129295, 122.7000000010924765, -2.066987299999998751 ) ) ;
#23844=CARTESIAN_POINT ( 'NONE',  ( 102.1631189606246295, 116.6573956140660897, -50.60000000000000853 ) ) ;
#23846=CARTESIAN_POINT ( 'NONE',  ( 99.14382582708707048, 124.1000000010924964, 2.066987299999979211 ) ) ;
#23874=DIRECTION ( 'NONE',  ( 1.000000000000000000, -0.000000000000000000, -5.782411586589357392E-17 ) ) ;
#23879=CARTESIAN_POINT ( 'NONE',  ( 99.99999999999998579, 90.00000000000000000, 4.999999999999983125 ) ) ;
#23884=DIRECTION ( 'NONE',  ( -1.000000000000000000, 0.000000000000000000, 0.000000000000000000 ) ) ;
#23889=CARTESIAN_POINT ( 'NONE',  ( 99.99999999999998579, 123.9500000010924765, 2.066987299999980099 ) ) ;
#23896=CARTESIAN_POINT ( 'NONE',  ( 91.91746824999998466, 112.6261737610028320, -49.22500000273119269 ) ) ;
#23897=FACE_OUTER_BOUND ( 'NONE', #10030, .T. ) ;
#23902=ORIENTED_EDGE ( 'NONE', *, *, #14212, .T. ) ;
#23903=LINE ( 'NONE', #245, #16375 ) ;
#23919=LINE ( 'NONE', #6116, #21440 ) ;
#23928=CARTESIAN_POINT ( 'NONE',  ( 112.9999999999999858, 118.0000000000000000, -15.00000000000000533 ) ) ;
#23933=CARTESIAN_POINT ( 'NONE',  ( 99.99999999999998579, 93.56249999863440792, -4.458734124999994997 ) ) ;
#23939=VECTOR ( 'NONE', #387, 1000.000000000000000 ) ;
#23940=CARTESIAN_POINT ( 'NONE',  ( 104.4587341249999781, 95.31249999863440792, -6.938893903907228378E-15 ) ) ;
#23941=CARTESIAN_POINT ( 'NONE',  ( 99.99999999999998579, 94.81249999863440792, -4.458734124999994997 ) ) ;
#23953=( BOUNDED_SURFACE ( )  B_SPLINE_SURFACE ( 1, 2, ( 
 ( #8401, #16951, #14665, #21108, #7855, #23664, #16550, #23387, #4140, #18693, #27808, #25241, #5732, #1595, #27533, #3859, #7990, #23252, #1730, #3727, #10394, #19100, #8264, #25652, #28081, #2145, #11232, #21523, #23798, #26366, #15662, #6680, #19949, #19660, #17377, #26511, #8971, #10807, #25936, #8545, #6826, #24362, #142, #286, #26221, #13075, #19522, #21814, #22093, #15516, #3, #4421, #4704, #9113, #2290, #24224, #10949, #13365, #8828, #8688, #2430, #17518, #6967, #15366, #26073, #17808, #6542, #2571, #4850, #4277, #427, #2003, #10669, #19378, #15222, #4558, #17234, #6411, #15080, #12935, #23940 ),
 ( #24082, #21668, #13220, #21952, #11091, #19802, #17659, #18379, #13795, #27084, #2984, #20233, #22664, #20380, #18524, #9538, #18087, #1150, #2846, #5418, #16374, #15803, #3275, #7537, #14087, #25075, #716, #24790, #22807, #22234, #16235, #20666, #22373, #11658, #5128, #7389, #11515, #13514, #2713, #27229, #9817, #7682, #7248, #22518, #865, #7106, #11374, #11944, #1008, #9391, #20096, #5272, #574, #9255, #17947, #24932, #26658, #24507, #18237, #4994, #13658, #26946, #16082, #26799, #15939, #24655, #13938, #9677, #3134, #11803, #20527, #21216, #5835, #27774, #8232, #20942, #25490, #1700, #25210, #5968, #14772 ) ),
 .UNSPECIFIED., .F., .F., .T. ) 
 B_SPLINE_SURFACE_WITH_KNOTS ( ( 2, 2 ),
 ( 3, 2, 2, 2, 2, 2, 2, 2, 2, 2, 2, 2, 2, 2, 2, 2, 2, 2, 2, 2, 2, 2, 2, 2, 2, 2, 2, 2, 2, 2, 2, 2, 2, 2, 2, 2, 2, 2, 2, 2, 3 ),
 ( 0.000000000000000000, 1.000000000000000000 ),
 ( 0.000000000000000000, 0.02500000000000000139, 0.05000000000000000278, 0.07499999999999999722, 0.1000000000000000056, 0.1250000000000000000, 0.1499999999999999944, 0.1749999999999999889, 0.2000000000000000111, 0.2250000000000000056, 0.2500000000000000000, 0.2750000000000000222, 0.2999999999999999889, 0.3250000000000000111, 0.3499999999999999778, 0.3750000000000000000, 0.4000000000000000222, 0.4249999999999999889, 0.4500000000000000111, 0.4749999999999999778, 0.5000000000000000000, 0.5250000000000000222, 0.5500000000000000444, 0.5749999999999999556, 0.5999999999999999778, 0.6250000000000000000, 0.6500000000000000222, 0.6750000000000000444, 0.6999999999999999556, 0.7249999999999999778, 0.7500000000000000000, 0.7750000000000000222, 0.8000000000000000444, 0.8249999999999999556, 0.8499999999999999778, 0.8750000000000000000, 0.9000000000000000222, 0.9250000000000000444, 0.9499999999999999556, 0.9749999999999999778, 1.000000000000000000 ),
 .UNSPECIFIED. ) 
 GEOMETRIC_REPRESENTATION_ITEM ( )  RATIONAL_B_SPLINE_SURFACE ( (
 ( 1.000000000000000000, 0.9238795325112867385, 1.000000000000000000, 0.9238795325112867385, 1.000000000000000000, 0.9238795325112867385, 1.000000000000000000, 0.9238795325112867385, 1.000000000000000000, 0.9238795325112867385, 1.000000000000000000, 0.9238795325112867385, 1.000000000000000000, 0.9238795325112867385, 1.000000000000000000, 0.9238795325112867385, 1.000000000000000000, 0.9238795325112867385, 1.000000000000000000, 0.9238795325112867385, 1.000000000000000000, 0.9238795325112867385, 1.000000000000000000, 0.9238795325112867385, 1.000000000000000000, 0.9238795325112867385, 1.000000000000000000, 0.9238795325112867385, 1.000000000000000000, 0.9238795325112867385, 1.000000000000000000, 0.9238795325112867385, 1.000000000000000000, 0.9238795325112867385, 1.000000000000000000, 0.9238795325112867385, 1.000000000000000000, 0.9238795325112867385, 1.000000000000000000, 0.9238795325112867385, 1.000000000000000000, 0.9238795325112867385, 1.000000000000000000, 0.9238795325112867385, 1.000000000000000000, 0.9238795325112867385, 1.000000000000000000, 0.9238795325112867385, 1.000000000000000000, 0.9238795325112867385, 1.000000000000000000, 0.9238795325112867385, 1.000000000000000000, 0.9238795325112867385, 1.000000000000000000, 0.9238795325112867385, 1.000000000000000000, 0.9238795325112867385, 1.000000000000000000, 0.9238795325112867385, 1.000000000000000000, 0.9238795325112867385, 1.000000000000000000, 0.9238795325112867385, 1.000000000000000000, 0.9238795325112867385, 1.000000000000000000, 0.9238795325112867385, 1.000000000000000000, 0.9238795325112867385, 1.000000000000000000, 0.9238795325112867385, 1.000000000000000000, 0.9238795325112867385, 1.000000000000000000, 0.9238795325112867385, 1.000000000000000000, 0.9238795325112867385, 1.000000000000000000, 0.9238795325112867385, 1.000000000000000000),
 ( 1.000000000000000000, 0.9238795325112867385, 1.000000000000000000, 0.9238795325112867385, 1.000000000000000000, 0.9238795325112867385, 1.000000000000000000, 0.9238795325112867385, 1.000000000000000000, 0.9238795325112867385, 1.000000000000000000, 0.9238795325112867385, 1.000000000000000000, 0.9238795325112867385, 1.000000000000000000, 0.9238795325112867385, 1.000000000000000000, 0.9238795325112867385, 1.000000000000000000, 0.9238795325112867385, 1.000000000000000000, 0.9238795325112867385, 1.000000000000000000, 0.9238795325112867385, 1.000000000000000000, 0.9238795325112867385, 1.000000000000000000, 0.9238795325112867385, 1.000000000000000000, 0.9238795325112867385, 1.000000000000000000, 0.9238795325112867385, 1.000000000000000000, 0.9238795325112867385, 1.000000000000000000, 0.9238795325112867385, 1.000000000000000000, 0.9238795325112867385, 1.000000000000000000, 0.9238795325112867385, 1.000000000000000000, 0.9238795325112867385, 1.000000000000000000, 0.9238795325112867385, 1.000000000000000000, 0.9238795325112867385, 1.000000000000000000, 0.9238795325112867385, 1.000000000000000000, 0.9238795325112867385, 1.000000000000000000, 0.9238795325112867385, 1.000000000000000000, 0.9238795325112867385, 1.000000000000000000, 0.9238795325112867385, 1.000000000000000000, 0.9238795325112867385, 1.000000000000000000, 0.9238795325112867385, 1.000000000000000000, 0.9238795325112867385, 1.000000000000000000, 0.9238795325112867385, 1.000000000000000000, 0.9238795325112867385, 1.000000000000000000, 0.9238795325112867385, 1.000000000000000000, 0.9238795325112867385, 1.000000000000000000, 0.9238795325112867385, 1.000000000000000000, 0.9238795325112867385, 1.000000000000000000, 0.9238795325112867385, 1.000000000000000000, 0.9238795325112867385, 1.000000000000000000, 0.9238795325112867385, 1.000000000000000000) ) ) 
 REPRESENTATION_ITEM ( '' )  SURFACE ( )  );
#23956=CARTESIAN_POINT ( 'NONE',  ( 108.0825317500000011, 107.3738262389971680, -44.22500000273119269 ) ) ;
#23958=ORIENTED_EDGE ( 'NONE', *, *, #25711, .F. ) ;
#23962=CARTESIAN_POINT ( 'NONE',  ( 112.9999999999999858, 125.0000000000000000, -13.00000000000001066 ) ) ;
#23963=EDGE_CURVE ( 'NONE', #12415, #3280, #26032, .T. ) ;
#23967=CARTESIAN_POINT ( 'NONE',  ( 97.50236033167492167, 102.3130555110000159, -52.72500000273119980 ) ) ;
#23968=CARTESIAN_POINT ( 'NONE',  ( 102.4999999999999858, 123.7999999999999972, -9.847140817659276890E-15 ) ) ;
#23972=ADVANCED_FACE ( 'NONE', ( #14164 ), #18736, .F. ) ;
#23975=CARTESIAN_POINT ( 'NONE',  ( 93.00000000000000000, 112.2744378736303190, -50.60000000546237686 ) ) ;
#23980=ORIENTED_EDGE ( 'NONE', *, *, #4292, .F. ) ;
#23985=CARTESIAN_POINT ( 'NONE',  ( 104.3262379212492590, 115.9545556584642867, -52.70000000000000284 ) ) ;
#23987=CARTESIAN_POINT ( 'NONE',  ( 99.99999999999998579, 92.62499999726881583, 4.999999999999984013 ) ) ;
#23990=CARTESIAN_POINT ( 'NONE',  ( 102.0710678118654613, 93.06249999726880162, -4.999999999999997335 ) ) ;
#23993=DIRECTION ( 'NONE',  ( 1.000000000000000000, 0.000000000000000000, -5.782411586589357392E-17 ) ) ;
#23994=ORIENTED_EDGE ( 'NONE', *, *, #16966, .F. ) ;
#24017=VERTEX_POINT ( 'NONE', #8036 ) ;
#24023=CARTESIAN_POINT ( 'NONE',  ( 91.91746824999999887, 110.0000000000000000, -53.12500000273119838 ) ) ;
#24028=DIRECTION ( 'NONE',  ( 0.000000000000000000, 0.000000000000000000, 1.000000000000000000 ) ) ;
#24030=CARTESIAN_POINT ( 'NONE',  ( 98.53841926354351699, 124.4500000010924765, -1.461580736456474794 ) ) ;
#24037=CARTESIAN_POINT ( 'NONE',  ( 104.9952793366501851, 116.8754121666685393, -53.82500000273119412 ) ) ;
#24040=( BOUNDED_CURVE ( )  B_SPLINE_CURVE ( 2, ( #882, #18255, #24947, #17823, #26528, #26819, #5434, #14101, #9269, #9406, #734 ),
 .UNSPECIFIED., .F., .F. ) 
 B_SPLINE_CURVE_WITH_KNOTS ( ( 3, 2, 2, 2, 2, 3 ),
 ( 0.3000000000000002109, 0.3200000000000001177, 0.3400000000000000244, 0.3599999999999998757, 0.3799999999999997824, 0.3999999999999996891 ),
 .UNSPECIFIED. ) 
 CURVE ( )  GEOMETRIC_REPRESENTATION_ITEM ( )  RATIONAL_B_SPLINE_CURVE ( ( 0.9999999999999994449, 0.9510565162951540863, 1.000000000000000000, 0.9510565162951535312, 1.000000000000000000, 0.9510565162951535312, 1.000000000000000000, 0.9510565162951535312, 1.000000000000000000, 0.9510565162951543083, 0.9999999999999992228 ) ) 
 REPRESENTATION_ITEM ( '' )  );
#24052=LINE ( 'NONE', #13189, #5244 ) ;
#24058=CYLINDRICAL_SURFACE ( 'NONE', #24743, 4.999999999999989342 ) ;
#24069=CARTESIAN_POINT ( 'NONE',  ( 102.4976396683250925, 117.6869444889999841, -45.97500000273119269 ) ) ;
#24073=CARTESIAN_POINT ( 'NONE',  ( 99.99999999999998579, 102.6397644303321215, -44.00000000546238255 ) ) ;
#24074=CARTESIAN_POINT ( 'NONE',  ( 103.1528011352953484, 95.18749999863440792, 3.152801135295352886 ) ) ;
#24082=CARTESIAN_POINT ( 'NONE',  ( 104.9999999999999858, 90.00000000000000000, -6.938893903907228378E-15 ) ) ;
#24101=CARTESIAN_POINT ( 'NONE',  ( 103.5355339059327235, 91.87500000000000000, 3.535533905932724874 ) ) ;
#24104=EDGE_CURVE ( 'NONE', #15121, #17145, #27872, .T. ) ;
#24106=CARTESIAN_POINT ( 'NONE',  ( 108.0825317500000153, 110.0000000000000000, -52.12500000273119838 ) ) ;
#24115=CARTESIAN_POINT ( 'NONE',  ( 101.4615807364564546, 123.2500000010924879, 1.461580736456455476 ) ) ;
#24127=CARTESIAN_POINT ( 'NONE',  ( 95.67376207875072680, 115.9545556584642867, -48.30000000000001137 ) ) ;
#24129=CARTESIAN_POINT ( 'NONE',  ( 98.23223304703363112, 124.2999999999999972, 1.767766952966351557 ) ) ;
#24132=CARTESIAN_POINT ( 'NONE',  ( 104.9999999999999858, 91.87499999726880162, -6.938893903907228378E-15 ) ) ;
#24144=AXIS2_PLACEMENT_3D ( 'NONE', #18919, #7949, #10074 ) ;
#24146=CARTESIAN_POINT ( 'NONE',  ( 84.99999999999998579, 125.0000000000000000, -13.00000000000000888 ) ) ;
#24148=CARTESIAN_POINT ( 'NONE',  ( 112.9999999999999858, 118.0000000000000000, -43.00000000000000000 ) ) ;
#24150=ORIENTED_EDGE ( 'NONE', *, *, #6510, .T. ) ;
#24151=EDGE_CURVE ( 'NONE', #20470, #1287, #20049, .T. ) ;
#24160=CARTESIAN_POINT ( 'NONE',  ( 84.99999999999998579, 99.99999999999998579, -45.00000000000000711 ) ) ;
#24168=CARTESIAN_POINT ( 'NONE',  ( 101.7677669529663547, 123.2000000021849502, -1.767766952966370209 ) ) ;
#24171=VERTEX_POINT ( 'NONE', #12648 ) ;
#24174=CARTESIAN_POINT ( 'NONE',  ( 99.14382582708707048, 124.4000000010924794, -2.066987299999999195 ) ) ;
#24180=CARTESIAN_POINT ( 'NONE',  ( 93.46109445667491400, 114.7507929638356785, -53.32500000273119412 ) ) ;
#24187=ORIENTED_EDGE ( 'NONE', *, *, #13831, .F. ) ;
#24203=ORIENTED_EDGE ( 'NONE', *, *, #19414, .F. ) ;
#24204=CARTESIAN_POINT ( 'NONE',  ( 84.99999999999998579, 97.00000000000000000, 12.99999999999999467 ) ) ;
#24212=CARTESIAN_POINT ( 'NONE',  ( 108.0825317500000011, 107.3738262389971680, -44.47500000273118559 ) ) ;
#24216=CARTESIAN_POINT ( 'NONE',  ( 100.5280963304672923, 123.0000000000000000, 2.448276570249286799 ) ) ;
#24224=CARTESIAN_POINT ( 'NONE',  ( 95.54126587499999346, 93.74999999863439371, -1.846868145590737864 ) ) ;
#24225=CARTESIAN_POINT ( 'NONE',  ( 104.4587341249999923, 95.49999999863442213, 1.846868145590726318 ) ) ;
#24229=DIRECTION ( 'NONE',  ( -5.782411586589357392E-17, -1.156482317317871478E-16, -1.000000000000000000 ) ) ;
#24231=ORIENTED_EDGE ( 'NONE', *, *, #116, .T. ) ;
#24246=CARTESIAN_POINT ( 'NONE',  ( 102.1631189606246295, 116.6573956140660897, -53.10000000546238397 ) ) ;
#24248=DIRECTION ( 'NONE',  ( -0.8660254037844418162, -0.000000000000000000, -0.4999999999999947264 ) ) ;
#24256=CARTESIAN_POINT ( 'NONE',  ( 97.93301270000000613, 122.9500000010924765, -9.540979117872439019E-15 ) ) ;
#24257=CARTESIAN_POINT ( 'NONE',  ( 84.99999999999998579, 125.0000000000000000, -15.00000000000000888 ) ) ;
#24260=CARTESIAN_POINT ( 'NONE',  ( 99.99999999999998579, 90.00000000000000000, 4.999999999999983125 ) ) ;
#24264=CARTESIAN_POINT ( 'NONE',  ( 107.0000000000000142, 107.7255621263696526, -47.10000000000000853 ) ) ;
#24266=CARTESIAN_POINT ( 'NONE',  ( 99.99999999999998579, 124.3999999999999915, 2.499999999999978684 ) ) ;
#24270=CARTESIAN_POINT ( 'NONE',  ( 103.5355339059327235, 92.99999999726881583, -3.535533905932738197 ) ) ;
#24275=EDGE_CURVE ( 'NONE', #2287, #19200, #25226, .T. ) ;
#24281=CARTESIAN_POINT ( 'NONE',  ( 104.9999999999999858, 90.87499999726880162, -6.938893903907228378E-15 ) ) ;
#24306=ORIENTED_EDGE ( 'NONE', *, *, #8782, .T. ) ;
#24307=CARTESIAN_POINT ( 'NONE',  ( 99.14382582708707048, 123.1000000010924822, 2.066987299999979211 ) ) ;
#24315=CARTESIAN_POINT ( 'NONE',  ( 91.91746824999999887, 110.0000000000000000, -45.12500000273119838 ) ) ;
#24331=ORIENTED_EDGE ( 'NONE', *, *, #18185, .T. ) ;
#24348=CARTESIAN_POINT ( 'NONE',  ( 91.91746824999999887, 110.0000000000000000, -45.37500000273119838 ) ) ;
#24352=CARTESIAN_POINT ( 'NONE',  ( 102.5000695353236324, 123.0000000000000426, -0.2897305190755338211 ) ) ;
#24362=CARTESIAN_POINT ( 'NONE',  ( 95.54126587499999346, 92.87499999863440792, 1.846868145590722543 ) ) ;
#24363=CARTESIAN_POINT ( 'NONE',  ( 103.1528011352953484, 94.43749999863440792, 3.152801135295352886 ) ) ;
#24366=VECTOR ( 'NONE', #15706, 1000.000000000000000 ) ;
#24373=( BOUNDED_SURFACE ( )  B_SPLINE_SURFACE ( 1, 2, ( 
 ( #7528, #1275, #26793, #7674, #13788, #20517, #2839, #11650, #858, #20795, #17940, #24924, #20226, #20657, #13930, #25067, #18080, #1142, #20373, #5410, #14078, #3400, #26650, #12070, #7239, #7098, #24648, #15796, #5121, #15931, #22509, #14495, #5827, #1830, #17049, #8364, #16510, #21483, #14764, #10210, #25203 ),
 ( #10494, #25753, #18787, #8088, #1557, #3820, #27494, #12765, #18655, #21207, #21350, #5689, #12624, #10349, #19201, #18920, #1692, #23072, #10075, #12480, #16783, #27629, #3548, #23347, #25614, #19058, #20932, #27766, #1417, #14356, #3687, #9940, #27359, #7950, #25482, #12205, #5960, #14628, #8224, #27903, #16914 ) ),
 .UNSPECIFIED., .F., .F., .F. ) 
 B_SPLINE_SURFACE_WITH_KNOTS ( ( 2, 2 ),
 ( 3, 2, 2, 2, 2, 2, 2, 2, 2, 2, 2, 2, 2, 2, 2, 2, 2, 2, 2, 2, 3 ),
 ( 0.000000000000000000, 1.000000000000000000 ),
 ( 0.000000000000000000, 0.04166666666666666435, 0.08333333333333332871, 0.1250000000000000000, 0.1666666666666666574, 0.2083333333333333426, 0.2500000000000000000, 0.2916666666666666852, 0.3333333333333333148, 0.3750000000000000000, 0.4166666666666666852, 0.4583333333333333148, 0.5000000000000000000, 0.5416666666666666297, 0.5833333333333333703, 0.6250000000000000000, 0.6666666666666666297, 0.7083333333333333703, 0.7500000000000000000, 0.7916666666666666297, 0.8333333333333333703 ),
 .UNSPECIFIED. ) 
 GEOMETRIC_REPRESENTATION_ITEM ( )  RATIONAL_B_SPLINE_SURFACE ( (
 ( 1.000000000000000000, 0.9238795325112867385, 1.000000000000000000, 0.9238795325112867385, 1.000000000000000000, 0.9238795325112867385, 1.000000000000000000, 0.9238795325112867385, 1.000000000000000000, 0.9238795325112867385, 1.000000000000000000, 0.9238795325112867385, 1.000000000000000000, 0.9238795325112867385, 1.000000000000000000, 0.9238795325112867385, 1.000000000000000000, 0.9238795325112867385, 1.000000000000000000, 0.9238795325112867385, 1.000000000000000000, 0.9238795325112867385, 1.000000000000000000, 0.9238795325112867385, 1.000000000000000000, 0.9238795325112867385, 1.000000000000000000, 0.9238795325112867385, 1.000000000000000000, 0.9238795325112867385, 1.000000000000000000, 0.9238795325112867385, 1.000000000000000000, 0.9238795325112867385, 1.000000000000000000, 0.9238795325112867385, 1.000000000000000000, 0.9238795325112867385, 1.000000000000000000, 0.9238795325112867385, 1.000000000000000000),
 ( 1.000000000000000000, 0.9238795325112867385, 1.000000000000000000, 0.9238795325112867385, 1.000000000000000000, 0.9238795325112867385, 1.000000000000000000, 0.9238795325112867385, 1.000000000000000000, 0.9238795325112867385, 1.000000000000000000, 0.9238795325112867385, 1.000000000000000000, 0.9238795325112867385, 1.000000000000000000, 0.9238795325112867385, 1.000000000000000000, 0.9238795325112867385, 1.000000000000000000, 0.9238795325112867385, 1.000000000000000000, 0.9238795325112867385, 1.000000000000000000, 0.9238795325112867385, 1.000000000000000000, 0.9238795325112867385, 1.000000000000000000, 0.9238795325112867385, 1.000000000000000000, 0.9238795325112867385, 1.000000000000000000, 0.9238795325112867385, 1.000000000000000000, 0.9238795325112867385, 1.000000000000000000, 0.9238795325112867385, 1.000000000000000000, 0.9238795325112867385, 1.000000000000000000, 0.9238795325112867385, 1.000000000000000000) ) ) 
 REPRESENTATION_ITEM ( '' )  SURFACE ( )  );
#24386=CARTESIAN_POINT ( 'NONE',  ( 99.99999999999998579, 101.5015231886685854, -44.62500000273119838 ) ) ;
#24399=ORIENTED_EDGE ( 'NONE', *, *, #5130, .F. ) ;
#24403=CARTESIAN_POINT ( 'NONE',  ( 105.6631189606246295, 105.8855032339526758, -45.20000000000000284 ) ) ;
#24406=CARTESIAN_POINT ( 'NONE',  ( 102.4999999999999716, 124.6500000000000199, -1.035533905932742638 ) ) ;
#24409=CARTESIAN_POINT ( 'NONE',  ( 99.99999999999998579, 93.12499999726881583, -4.999999999999997335 ) ) ;
#24412=CARTESIAN_POINT ( 'NONE',  ( 93.46109445667491400, 114.7507929638356785, -49.57500000273120122 ) ) ;
#24428=VECTOR ( 'NONE', #17404, 1000.000000000000000 ) ;
#24447=ORIENTED_EDGE ( 'NONE', *, *, #21332, .T. ) ;
#24450=ORIENTED_EDGE ( 'NONE', *, *, #8283, .T. ) ;
#24451=CARTESIAN_POINT ( 'NONE',  ( 99.14382582708707048, 123.9000000010924794, 2.066987299999979211 ) ) ;
#24463=CARTESIAN_POINT ( 'NONE',  ( 99.99999999999998579, 117.3602355696678643, -49.00000000546238255 ) ) ;
#24465=CARTESIAN_POINT ( 'NONE',  ( 95.00000000000000000, 91.43749999726880162, 2.071067811865463959 ) ) ;
#24468=ORIENTED_EDGE ( 'NONE', *, *, #2338, .F. ) ;
#24484=EDGE_CURVE ( 'NONE', #9459, #14663, #24913, .T. ) ;
#24497=CARTESIAN_POINT ( 'NONE',  ( 99.99999999999998579, 101.5015231886685854, -52.87500000273119838 ) ) ;
#24498=CARTESIAN_POINT ( 'NONE',  ( 97.51692799888628826, 122.9999999999999716, -0.4114429061860825354 ) ) ;
#24507=CARTESIAN_POINT ( 'NONE',  ( 95.00000000000000000, 93.56249999999998579, 2.071067811865463959 ) ) ;
#24508=CARTESIAN_POINT ( 'NONE',  ( 104.4587341249999781, 94.56249999863440792, -6.938893903907228378E-15 ) ) ;
#24513=VERTEX_POINT ( 'NONE', #7368 ) ;
#24522=DIRECTION ( 'NONE',  ( 0.000000000000000000, 0.000000000000000000, -1.000000000000000000 ) ) ;
#24526=CARTESIAN_POINT ( 'NONE',  ( 98.15313185440923860, 91.62499999863439371, -4.458734124999994997 ) ) ;
#24531=CARTESIAN_POINT ( 'NONE',  ( 108.0825317500000011, 112.6261737610028320, -46.02500000273120406 ) ) ;
#24533=FACE_OUTER_BOUND ( 'NONE', #27869, .T. ) ;
#24539=( BOUNDED_CURVE ( )  B_SPLINE_CURVE ( 2, ( #19470, #14754, #23613, #21339, #16905, #25473, #25602, #17183, #19328, #14619, #27755 ),
 .UNSPECIFIED., .F., .T. ) 
 B_SPLINE_CURVE_WITH_KNOTS ( ( 3, 2, 2, 2, 2, 3 ),
 ( 0.1000000000000000056, 0.1200000000000000233, 0.1400000000000000688, 0.1600000000000001144, 0.1800000000000001044, 0.2000000000000001776 ),
 .UNSPECIFIED. ) 
 CURVE ( )  GEOMETRIC_REPRESENTATION_ITEM ( )  RATIONAL_B_SPLINE_CURVE ( ( 1.000000000000000000, 0.9510565162951535312, 1.000000000000000000, 0.9510565162951535312, 1.000000000000000000, 0.9510565162951535312, 1.000000000000000000, 0.9510565162951535312, 1.000000000000000000, 0.9510565162951530871, 1.000000000000000444 ) ) 
 REPRESENTATION_ITEM ( '' )  );
#24542=EDGE_CURVE ( 'NONE', #4950, #20336, #13637, .T. ) ;
#24545=( BOUNDED_CURVE ( )  B_SPLINE_CURVE ( 2, ( #5805, #18895, #18632, #27605, #8064, #3375, #16758, #5939, #3244, #3104, #7505 ),
 .UNSPECIFIED., .F., .F. ) 
 B_SPLINE_CURVE_WITH_KNOTS ( ( 3, 2, 2, 2, 2, 3 ),
 ( 0.5999999999999998668, 0.6199999999999998845, 0.6399999999999999023, 0.6599999999999999201, 0.6799999999999999378, 0.6999999999999998446 ),
 .UNSPECIFIED. ) 
 CURVE ( )  GEOMETRIC_REPRESENTATION_ITEM ( )  RATIONAL_B_SPLINE_CURVE ( ( 1.000000000000000222, 0.9510565162951533091, 1.000000000000000000, 0.9510565162951535312, 1.000000000000000000, 0.9510565162951535312, 1.000000000000000000, 0.9510565162951535312, 1.000000000000000000, 0.9510565162951537532, 0.9999999999999997780 ) ) 
 REPRESENTATION_ITEM ( '' )  );
#24549=CARTESIAN_POINT ( 'NONE',  ( 104.3262379212492590, 104.0454443415356991, -47.30000000000000426 ) ) ;
#24557=CARTESIAN_POINT ( 'NONE',  ( 95.00000000000000000, 93.37499999726881583, -7.551217303480904118E-15 ) ) ;
#24560=CARTESIAN_POINT ( 'NONE',  ( 106.5389055433251002, 114.7507929638356785, -50.17500000273119554 ) ) ;
#24578=ORIENTED_EDGE ( 'NONE', *, *, #2702, .T. ) ;
#24587=CARTESIAN_POINT ( 'NONE',  ( 104.9952793366501709, 116.8754121666685393, -47.82500000273119412 ) ) ;
#24595=ADVANCED_FACE ( 'NONE', ( #22496 ), #26781, .T. ) ;
#24605=CARTESIAN_POINT ( 'NONE',  ( 105.0000000000000000, 110.0000000000000000, -45.00000000000000711 ) ) ;
#24606=CARTESIAN_POINT ( 'NONE',  ( 104.4587341249999923, 92.37499999863440792, -1.846868145590737198 ) ) ;
#24607=CARTESIAN_POINT ( 'NONE',  ( 99.99999999999998579, 101.5015231886685854, -48.62500000273119838 ) ) ;
#24620=CIRCLE ( 'NONE', #12301, 7.000000000000006217 ) ;
#24630=LINE ( 'NONE', #5107, #27344 ) ;
#24633=CARTESIAN_POINT ( 'NONE',  ( 99.99999999999998579, 89.99899999999999523, -9.540979117872439019E-15 ) ) ;
#24645=ADVANCED_FACE ( 'NONE', ( #7663 ), #18357, .F. ) ;
#24646=CARTESIAN_POINT ( 'NONE',  ( 104.9952793366501851, 116.8754121666685393, -52.07500000273120122 ) ) ;
#24647=CARTESIAN_POINT ( 'NONE',  ( 101.7406320503887684, 123.0000000000000000, -1.800178865752367408 ) ) ;
#24648=CARTESIAN_POINT ( 'NONE',  ( 101.4615807364564546, 123.2500000010924879, 1.461580736456455476 ) ) ;
#24655=CARTESIAN_POINT ( 'NONE',  ( 104.9999999999999716, 94.06249999999998579, -2.071067811865478170 ) ) ;
#24672=CARTESIAN_POINT ( 'NONE',  ( 96.84719886470463734, 90.68749999863440792, -3.152801135295366208 ) ) ;
#24679=CARTESIAN_POINT ( 'NONE',  ( 97.50236033167492167, 117.6869444889999841, -45.52500000273119696 ) ) ;
#24680=CARTESIAN_POINT ( 'NONE',  ( 96.84719886470463734, 90.93749999863440792, -3.152801135295366208 ) ) ;
#24694=CARTESIAN_POINT ( 'NONE',  ( 104.3262379212492590, 115.9545556584642867, -46.69999999999999574 ) ) ;
#24701=CARTESIAN_POINT ( 'NONE',  ( 95.54126587500000767, 93.06249999863440792, -7.484931351350258973E-15 ) ) ;
#24703=CARTESIAN_POINT ( 'NONE',  ( 108.0825317500000153, 110.0000000000000000, -50.37500000273119127 ) ) ;
#24704=AXIS2_PLACEMENT_3D ( 'NONE', #24633, #22352, #16355 ) ;
#24708=( BOUNDED_CURVE ( )  B_SPLINE_CURVE ( 2, ( #12340, #5044, #13708, #2477, #486, #22428, #12883 ),
 .UNSPECIFIED., .F., .F. ) 
 B_SPLINE_CURVE_WITH_KNOTS ( ( 3, 2, 2, 3 ),
 ( 0.4166666666666666297, 0.4583333333333332593, 0.5000000000000000000, 0.5416666676520737189 ),
 .UNSPECIFIED. ) 
 CURVE ( )  GEOMETRIC_REPRESENTATION_ITEM ( )  RATIONAL_B_SPLINE_CURVE ( ( 1.000000000000000000, 0.9238795325112866275, 1.000000000000000000, 0.9238795325112867385, 1.000000000000000000, 0.9238795325112867385, 1.000000000000000000 ) ) 
 REPRESENTATION_ITEM ( '' )  );
#24722=VERTEX_POINT ( 'NONE', #13353 ) ;
#24731=CARTESIAN_POINT ( 'NONE',  ( 95.00472066334981491, 103.1245878333314465, -44.82500000273118701 ) ) ;
#24743=AXIS2_PLACEMENT_3D ( 'NONE', #2406, #21930, #11066 ) ;
#24745=CARTESIAN_POINT ( 'NONE',  ( 106.5389055433251002, 114.7507929638356785, -47.92500000273120264 ) ) ;
#24758=( BOUNDED_CURVE ( )  B_SPLINE_CURVE ( 2, ( #23507, #8530, #15785, #20213, #4687, #125, #18067, #13639, #9372, #8951, #15645 ),
 .UNSPECIFIED., .F., .F. ) 
 B_SPLINE_CURVE_WITH_KNOTS ( ( 3, 2, 2, 2, 2, 3 ),
 ( 0.000000000000000000, 0.02000000000000000042, 0.04000000000000000083, 0.05999999999999999778, 0.08000000000000000167, 0.1000000000000000194 ),
 .UNSPECIFIED. ) 
 CURVE ( )  GEOMETRIC_REPRESENTATION_ITEM ( )  RATIONAL_B_SPLINE_CURVE ( ( 1.000000000000000000, 0.9510565162951535312, 1.000000000000000000, 0.9510565162951535312, 1.000000000000000000, 0.9510565162951535312, 1.000000000000000000, 0.9510565162951535312, 1.000000000000000000, 0.9510565162951535312, 1.000000000000000000 ) ) 
 REPRESENTATION_ITEM ( '' )  );
#24767=CARTESIAN_POINT ( 'NONE',  ( 98.23223304703363112, 124.1069999999781572, -1.767766952966370209 ) ) ;
#24771=CARTESIAN_POINT ( 'NONE',  ( 87.00000000000000000, 118.0000000000000000, -15.00000000000000533 ) ) ;
#24787=CARTESIAN_POINT ( 'NONE',  ( 94.99999999999998579, 110.0000000000000000, -45.00000000000000711 ) ) ;
#24788=CARTESIAN_POINT ( 'NONE',  ( 95.00000000000000000, 94.43750000000001421, -2.071067811865479058 ) ) ;
#24790=CARTESIAN_POINT ( 'NONE',  ( 97.92893218813452449, 91.68749999999998579, 4.999999999999983125 ) ) ;
#24808=CARTESIAN_POINT ( 'NONE',  ( 99.99999999999998579, 91.56249999863440792, -4.458734124999994997 ) ) ;
#24810=LINE ( 'NONE', #13678, #1382 ) ;
#24812=CARTESIAN_POINT ( 'NONE',  ( 99.99999999999998579, 123.6000000000000085, 2.499999999999978684 ) ) ;
#24815=CARTESIAN_POINT ( 'NONE',  ( 91.91746824999998466, 112.6261737610028320, -45.22500000273119980 ) ) ;
#24816=CARTESIAN_POINT ( 'NONE',  ( 104.4587341249999923, 92.62499999863439371, -1.846868145590737198 ) ) ;
#24818=CARTESIAN_POINT ( 'NONE',  ( 102.2113248666666436, 122.4666666681233096, -9.811788309856265935E-15 ) ) ;
#24820=ORIENTED_EDGE ( 'NONE', *, *, #4627, .T. ) ;
#24824=CARTESIAN_POINT ( 'NONE',  ( 98.96446609406724804, 123.6500000021849672, 2.499999999999969802 ) ) ;
#24826=VERTEX_POINT ( 'NONE', #20084 ) ;
#24827=EDGE_CURVE ( 'NONE', #24826, #15121, #18218, .T. ) ;
#24831=VERTEX_POINT ( 'NONE', #26355 ) ;
#24832=CARTESIAN_POINT ( 'NONE',  ( 108.0825317500000153, 110.0000000000000000, -52.37500000273119838 ) ) ;
#24835=LINE ( 'NONE', #25114, #7684 ) ;
#24841=CARTESIAN_POINT ( 'NONE',  ( 98.15313185440925281, 92.87499999863440792, -4.458734124999994997 ) ) ;
#24843=VECTOR ( 'NONE', #8258, 1000.000000000000000 ) ;
#24845=CARTESIAN_POINT ( 'NONE',  ( 106.5389055433251002, 114.7507929638356785, -52.17500000273119554 ) ) ;
#24846=EDGE_CURVE ( 'NONE', #20844, #9430, #13501, .T. ) ;
#24847=VERTEX_POINT ( 'NONE', #12924 ) ;
#24867=ORIENTED_EDGE ( 'NONE', *, *, #16054, .T. ) ;
#24872=CARTESIAN_POINT ( 'NONE',  ( 102.4976396683250925, 102.3130555110000159, -48.52500000273119696 ) ) ;
#24873=( BOUNDED_CURVE ( )  B_SPLINE_CURVE ( 2, ( #607, #24824, #3165, #22408, #13970, #751, #3020, #22271, #4885 ),
 .UNSPECIFIED., .F., .T. ) 
 B_SPLINE_CURVE_WITH_KNOTS ( ( 3, 2, 2, 2, 3 ),
 ( 0.2500000000000004441, 0.2916666666666670182, 0.3333333333333334814, 0.3750000000000000555, 0.4166666666666666297 ),
 .UNSPECIFIED. ) 
 CURVE ( )  GEOMETRIC_REPRESENTATION_ITEM ( )  RATIONAL_B_SPLINE_CURVE ( ( 0.9999999999999992228, 0.9238795325112875156, 1.000000000000000000, 0.9238795325112867385, 1.000000000000000000, 0.9238795325112867385, 1.000000000000000000, 0.9238795325112868495, 0.9999999999999998890 ) ) 
 REPRESENTATION_ITEM ( '' )  );
#24875=CARTESIAN_POINT ( 'NONE',  ( 102.0710678118654471, 90.18749999999997158, -5.000000000000000000 ) ) ;
#24878=ORIENTED_EDGE ( 'NONE', *, *, #12640, .F. ) ;
#24888=CARTESIAN_POINT ( 'NONE',  ( 93.46109445667491400, 105.2492070361643215, -46.92500000273119554 ) ) ;
#24890=CARTESIAN_POINT ( 'NONE',  ( 114.9999999999999858, 120.0000000000000000, -45.00000000000000711 ) ) ;
#24894=ORIENTED_EDGE ( 'NONE', *, *, #25008, .T. ) ;
#24898=AXIS2_PLACEMENT_3D ( 'NONE', #8324, #23309, #10306 ) ;
#24913=LINE ( 'NONE', #5252, #5136 ) ;
#24923=LINE ( 'NONE', #14077, #471 ) ;
#24924=CARTESIAN_POINT ( 'NONE',  ( 100.8561741729129295, 124.0000000010925021, 2.066987299999979211 ) ) ;
#24928=ORIENTED_EDGE ( 'NONE', *, *, #850, .T. ) ;
#24930=CARTESIAN_POINT ( 'NONE',  ( 99.99999999999998579, 92.75000000000000000, 4.999999999999984013 ) ) ;
#24932=CARTESIAN_POINT ( 'NONE',  ( 95.00000000000000000, 93.43750000000001421, -2.071067811865479058 ) ) ;
#24947=CARTESIAN_POINT ( 'NONE',  ( 94.33688103937537051, 105.8855032339526758, -50.30000000546237970 ) ) ;
#24948=CARTESIAN_POINT ( 'NONE',  ( 101.8468681455907330, 90.49999999863440792, -4.458734124999994997 ) ) ;
#24953=CARTESIAN_POINT ( 'NONE',  ( 97.93301270000000613, 124.5500000010924850, -9.540979117872439019E-15 ) ) ;
#24956=CARTESIAN_POINT ( 'NONE',  ( 107.0000000000000142, 110.0000000000000000, -49.50000000546238255 ) ) ;
#24957=CARTESIAN_POINT ( 'NONE',  ( 101.8468681455907330, 91.37499999863439371, 4.458734124999979898 ) ) ;
#24967=VERTEX_POINT ( 'NONE', #20513 ) ;
#24970=ORIENTED_EDGE ( 'NONE', *, *, #1505, .T. ) ;
#24971=CARTESIAN_POINT ( 'NONE',  ( 91.91746824999998466, 112.6261737610028320, -45.47500000273119980 ) ) ;
#24973=DIRECTION ( 'NONE',  ( -0.000000000000000000, 1.000000000000000000, -0.000000000000000000 ) ) ;
#24980=EDGE_CURVE ( 'NONE', #4858, #8561, #2407, .T. ) ;
#24982=CARTESIAN_POINT ( 'NONE',  ( 104.4587341249999923, 92.62499999863439371, -1.846868145590737198 ) ) ;
#24983=DIRECTION ( 'NONE',  ( -2.674902700537828060E-32, 1.000000000000000000, -4.625929269271485914E-16 ) ) ;
#24984=CARTESIAN_POINT ( 'NONE',  ( 91.91746824999998466, 107.3738262389971680, -49.27500000273118985 ) ) ;
#25003=PLANE ( 'NONE',  #18428 ) ;
#25006=ORIENTED_EDGE ( 'NONE', *, *, #8987, .F. ) ;
#25008=EDGE_CURVE ( 'NONE', #9430, #7349, #22652, .T. ) ;
#25013=CARTESIAN_POINT ( 'NONE',  ( 96.46446609406726225, 91.24999999726880162, -3.535533905932738197 ) ) ;
#25033=AXIS2_PLACEMENT_3D ( 'NONE', #21280, #12279, #22866 ) ;
#25044=CARTESIAN_POINT ( 'NONE',  ( 84.99999999999998579, 0.000000000000000000, 8.673617379884035472E-16 ) ) ;
#25049=CARTESIAN_POINT ( 'NONE',  ( 98.23223304703363112, 124.2999999999999972, 1.767766952966351557 ) ) ;
#25050=CARTESIAN_POINT ( 'NONE',  ( 98.96446609406727646, 124.8569999999781714, -2.499999999999997780 ) ) ;
#25061=EDGE_CURVE ( 'NONE', #20470, #12415, #4514, .T. ) ;
#25063=DIRECTION ( 'NONE',  ( 1.000000000000000000, 0.000000000000000000, -5.782411586589357392E-17 ) ) ;
#25066=CARTESIAN_POINT ( 'NONE',  ( 91.91746824999998466, 107.3738262389971538, -53.27500000273119696 ) ) ;
#25067=CARTESIAN_POINT ( 'NONE',  ( 97.93301269999999192, 123.8000000010924850, 0.8561741729129329626 ) ) ;
#25071=ORIENTED_EDGE ( 'NONE', *, *, #14212, .F. ) ;
#25072=CARTESIAN_POINT ( 'NONE',  ( 114.9999999999999858, 120.0000000000000000, -45.00000000000000711 ) ) ;
#25073=LINE ( 'NONE', #5561, #22154 ) ;
#25075=CARTESIAN_POINT ( 'NONE',  ( 95.00000000000000000, 91.56249999999998579, 2.071067811865463959 ) ) ;
#25076=STYLED_ITEM ( 'NONE', ( #11491 ), #17619 ) ;
#25088=LINE ( 'NONE', #22678, #9348 ) ;
#25091=CARTESIAN_POINT ( 'NONE',  ( 104.4587341249999781, 90.31249999863440792, -6.938893903907228378E-15 ) ) ;
#25100=CARTESIAN_POINT ( 'NONE',  ( 105.6631189606246295, 105.8855032339526758, -51.70000000546237828 ) ) ;
#25101=CARTESIAN_POINT ( 'NONE',  ( 95.54126587499999346, 94.99999999863439371, -1.846868145590737864 ) ) ;
#25111=ORIENTED_EDGE ( 'NONE', *, *, #1653, .F. ) ;
#25112=CARTESIAN_POINT ( 'NONE',  ( 97.50236033167492167, 102.3130555110000159, -44.97500000273119980 ) ) ;
#25114=CARTESIAN_POINT ( 'NONE',  ( 93.00000000000000000, 110.0000000000000000, -55.00000000000000711 ) ) ;
#25118=CARTESIAN_POINT ( 'NONE',  ( 101.8468681455907330, 91.74999999863439371, -4.458734124999994997 ) ) ;
#25127=DIRECTION ( 'NONE',  ( -5.782411586589357392E-17, 0.000000000000000000, -1.000000000000000000 ) ) ;
#25131=CARTESIAN_POINT ( 'NONE',  ( 104.4587341249999923, 95.49999999863440792, 1.846868145590726318 ) ) ;
#25135=ORIENTED_EDGE ( 'NONE', *, *, #4796, .F. ) ;
#25138=DIRECTION ( 'NONE',  ( 0.000000000000000000, 0.000000000000000000, 1.000000000000000000 ) ) ;
#25140=EDGE_LOOP ( 'NONE', ( #11298, #24578, #21866, #7185 ) ) ;
#25141=CARTESIAN_POINT ( 'NONE',  ( 95.00000000000000000, 92.56249999999998579, 2.071067811865463959 ) ) ;
#25146=EDGE_CURVE ( 'NONE', #4009, #923, #4395, .T. ) ;
#25162=ORIENTED_EDGE ( 'NONE', *, *, #20148, .T. ) ;
#25166=( BOUNDED_SURFACE ( )  B_SPLINE_SURFACE ( 1, 2, ( 
 ( #19425, #8871, #1916, #17563, #10581, #14991, #6181, #26267, #14848, #6727, #10718, #28126, #17422, #23846, #23431, #3905, #2191, #49, #19147, #12565, #27990, #21717, #23569, #8451, #27852, #4184, #26121, #21291, #17139, #12845, #21574, #17280, #25983, #6453, #15124, #4323, #15414, #9158, #332, #9433, #4893 ),
 ( #13408, #13261, #22280, #20137, #2886, #15704, #18132, #24406, #21993, #7008, #18282, #2470, #24266, #5174, #24129, #17711, #20274, #9578, #616, #13837, #13556, #11275, #2613, #2755, #22417, #11131, #19846, #760, #26988, #11418, #22135, #26845, #9018, #4748, #17850, #19996, #3030, #475, #4602, #26413, #26553 ) ),
 .UNSPECIFIED., .F., .F., .T. ) 
 B_SPLINE_SURFACE_WITH_KNOTS ( ( 2, 2 ),
 ( 3, 2, 2, 2, 2, 2, 2, 2, 2, 2, 2, 2, 2, 2, 2, 2, 2, 2, 2, 2, 3 ),
 ( 0.000000000000000000, 1.000000000000000000 ),
 ( 0.000000000000000000, 0.04166666666666666435, 0.08333333333333332871, 0.1250000000000000000, 0.1666666666666666574, 0.2083333333333333426, 0.2500000000000000000, 0.2916666666666666852, 0.3333333333333333148, 0.3750000000000000000, 0.4166666666666666852, 0.4583333333333333148, 0.5000000000000000000, 0.5416666666666666297, 0.5833333333333333703, 0.6250000000000000000, 0.6666666666666666297, 0.7083333333333333703, 0.7500000000000000000, 0.7916666666666666297, 0.8333333333333333703 ),
 .UNSPECIFIED. ) 
 GEOMETRIC_REPRESENTATION_ITEM ( )  RATIONAL_B_SPLINE_SURFACE ( (
 ( 1.000000000000000000, 0.9238795325112867385, 1.000000000000000000, 0.9238795325112867385, 1.000000000000000000, 0.9238795325112867385, 1.000000000000000000, 0.9238795325112867385, 1.000000000000000000, 0.9238795325112867385, 1.000000000000000000, 0.9238795325112867385, 1.000000000000000000, 0.9238795325112867385, 1.000000000000000000, 0.9238795325112867385, 1.000000000000000000, 0.9238795325112867385, 1.000000000000000000, 0.9238795325112867385, 1.000000000000000000, 0.9238795325112867385, 1.000000000000000000, 0.9238795325112867385, 1.000000000000000000, 0.9238795325112867385, 1.000000000000000000, 0.9238795325112867385, 1.000000000000000000, 0.9238795325112867385, 1.000000000000000000, 0.9238795325112867385, 1.000000000000000000, 0.9238795325112867385, 1.000000000000000000, 0.9238795325112867385, 1.000000000000000000, 0.9238795325112867385, 1.000000000000000000, 0.9238795325112867385, 1.000000000000000000),
 ( 1.000000000000000000, 0.9238795325112867385, 1.000000000000000000, 0.9238795325112867385, 1.000000000000000000, 0.9238795325112867385, 1.000000000000000000, 0.9238795325112867385, 1.000000000000000000, 0.9238795325112867385, 1.000000000000000000, 0.9238795325112867385, 1.000000000000000000, 0.9238795325112867385, 1.000000000000000000, 0.9238795325112867385, 1.000000000000000000, 0.9238795325112867385, 1.000000000000000000, 0.9238795325112867385, 1.000000000000000000, 0.9238795325112867385, 1.000000000000000000, 0.9238795325112867385, 1.000000000000000000, 0.9238795325112867385, 1.000000000000000000, 0.9238795325112867385, 1.000000000000000000, 0.9238795325112867385, 1.000000000000000000, 0.9238795325112867385, 1.000000000000000000, 0.9238795325112867385, 1.000000000000000000, 0.9238795325112867385, 1.000000000000000000, 0.9238795325112867385, 1.000000000000000000, 0.9238795325112867385, 1.000000000000000000) ) ) 
 REPRESENTATION_ITEM ( '' )  SURFACE ( )  );
#25183=CARTESIAN_POINT ( 'NONE',  ( 98.23223304703363112, 124.2999999999999972, 1.767766952966351557 ) ) ;
#25189=CARTESIAN_POINT ( 'NONE',  ( 107.0000000000000142, 110.0000000000000000, -47.50000000546238255 ) ) ;
#25198=CYLINDRICAL_SURFACE ( 'NONE', #15368, 4.999999999999989342 ) ;
#25201=CARTESIAN_POINT ( 'NONE',  ( 93.46109445667491400, 114.7507929638356785, -51.57500000273120122 ) ) ;
#25203=CARTESIAN_POINT ( 'NONE',  ( 102.0669872999999797, 122.5500000010924850, -9.794112055954760458E-15 ) ) ;
#25210=CARTESIAN_POINT ( 'NONE',  ( 103.5355339059327235, 94.87500000000000000, 3.535533905932724874 ) ) ;
#25217=ORIENTED_EDGE ( 'NONE', *, *, #21122, .F. ) ;
#25226=LINE ( 'NONE', #10789, #21062 ) ;
#25229=DIRECTION ( 'NONE',  ( 0.000000000000000000, 0.000000000000000000, -1.000000000000000000 ) ) ;
#25231=CARTESIAN_POINT ( 'NONE',  ( 95.67376207875072680, 115.9545556584642867, -52.80000000546237260 ) ) ;
#25233=CARTESIAN_POINT ( 'NONE',  ( 104.3262379212492590, 115.9545556584642867, -47.20000000546238539 ) ) ;
#25234=CARTESIAN_POINT ( 'NONE',  ( 99.99999999999998579, 95.31249999863440792, 4.458734124999981674 ) ) ;
#25241=CARTESIAN_POINT ( 'NONE',  ( 98.15313185440925281, 90.99999999863439371, 4.458734124999979898 ) ) ;
#25248=CARTESIAN_POINT ( 'NONE',  ( 106.5389055433251002, 105.2492070361643215, -50.57500000273120122 ) ) ;
#25255=CARTESIAN_POINT ( 'NONE',  ( 98.15313185440925281, 93.87499999863439371, -4.458734124999994997 ) ) ;
#25267=CARTESIAN_POINT ( 'NONE',  ( 102.0669873000000081, 124.1000000010924822, 0.8561741729129311862 ) ) ;
#25268=CARTESIAN_POINT ( 'NONE',  ( 96.84719886470463734, 93.18749999863440792, 3.152801135295351997 ) ) ;
#25287=CARTESIAN_POINT ( 'NONE',  ( 94.33688103937537051, 105.8855032339526758, -44.30000000546237970 ) ) ;
#25290=ORIENTED_EDGE ( 'NONE', *, *, #24275, .F. ) ;
#25296=CARTESIAN_POINT ( 'NONE',  ( 99.99999999999998579, 91.62499999726880162, 4.999999999999984013 ) ) ;
#25297=EDGE_CURVE ( 'NONE', #370, #20441, #21130, .T. ) ;
#25302=CARTESIAN_POINT ( 'NONE',  ( 99.99999999999998579, 90.00000000000000000, -6.938893903907228378E-15 ) ) ;
#25320=VECTOR ( 'NONE', #16052, 1000.000000000000000 ) ;
#25322=CARTESIAN_POINT ( 'NONE',  ( 102.4999999999999716, 123.8500000000000085, -1.035533905932742638 ) ) ;
#25330=CARTESIAN_POINT ( 'NONE',  ( 97.50000000000000000, 124.3000000021849587, -9.540979117872439019E-15 ) ) ;
#25338=CARTESIAN_POINT ( 'NONE',  ( 104.9952793366501851, 116.8754121666685393, -50.07500000273120122 ) ) ;
#25358=ORIENTED_EDGE ( 'NONE', *, *, #5693, .T. ) ;
#25361=CARTESIAN_POINT ( 'NONE',  ( 93.00000000000000000, 110.0000000000000000, -52.00000000000000711 ) ) ;
#25374=CARTESIAN_POINT ( 'NONE',  ( 99.99999999999998579, 93.25000000000000000, -4.999999999999997335 ) ) ;
#25378=CARTESIAN_POINT ( 'NONE',  ( 107.0000000000000142, 107.7255621263696526, -51.60000000546238397 ) ) ;
#25379=CARTESIAN_POINT ( 'NONE',  ( 95.54126587500000767, 94.06249999863440792, -7.484931351350258973E-15 ) ) ;
#25387=VECTOR ( 'NONE', #21451, 1000.000000000000000 ) ;
#25389=EDGE_CURVE ( 'NONE', #4172, #25694, #11974, .T. ) ;
#25390=VERTEX_POINT ( 'NONE', #22722 ) ;
#25394=CARTESIAN_POINT ( 'NONE',  ( 108.0825317500000011, 107.3738262389971538, -48.47500000273118559 ) ) ;
#25399=CARTESIAN_POINT ( 'NONE',  ( 97.50236033167492167, 102.3130555110000159, -46.72500000273119269 ) ) ;
#25414=EDGE_LOOP ( 'NONE', ( #213, #12516, #4768, #13286 ) ) ;
#25417=CARTESIAN_POINT ( 'NONE',  ( 96.84719886470463734, 95.18749999863440792, 3.152801135295351997 ) ) ;
#25426=ORIENTED_EDGE ( 'NONE', *, *, #20253, .F. ) ;
#25428=CARTESIAN_POINT ( 'NONE',  ( 100.0000000000000000, 110.0000000000000000, -55.00000000000000711 ) ) ;
#25432=CARTESIAN_POINT ( 'NONE',  ( 99.99999988184244160, 117.0000000000000000, -45.00000000000000711 ) ) ;
#25433=FACE_BOUND ( 'NONE', #14672, .T. ) ;
#25437=CARTESIAN_POINT ( 'NONE',  ( 87.00000000000000000, 123.0000000000000000, 12.99999999999999112 ) ) ;
#25443=CYLINDRICAL_SURFACE ( 'NONE', #10341, 2.499999999999995115 ) ;
#25458=( BOUNDED_CURVE ( )  B_SPLINE_CURVE ( 2, ( #9106, #13068, #15508, #12929, #6406, #15075, #19515, #26212, #17800 ),
 .UNSPECIFIED., .F., .F. ) 
 B_SPLINE_CURVE_WITH_KNOTS ( ( 3, 2, 2, 2, 3 ),
 ( 0.4500000000000003997, 0.4750000000000003664, 0.5000000000000004441, 0.5250000000000004663, 0.5500000000000004885 ),
 .UNSPECIFIED. ) 
 CURVE ( )  GEOMETRIC_REPRESENTATION_ITEM ( )  RATIONAL_B_SPLINE_CURVE ( ( 0.9999999999999987788, 0.9238795325112879597, 1.000000000000000000, 0.9238795325112867385, 1.000000000000000000, 0.9238795325112867385, 1.000000000000000000, 0.9238795325112854062, 1.000000000000001332 ) ) 
 REPRESENTATION_ITEM ( '' )  );
#25466=CARTESIAN_POINT ( 'NONE',  ( 102.4999999999999858, 123.7999999999999972, -9.847140817659276890E-15 ) ) ;
#25468=CARTESIAN_POINT ( 'NONE',  ( 98.53841926354351699, 123.8500000010924680, -1.461580736456474794 ) ) ;
#25473=CARTESIAN_POINT ( 'NONE',  ( 99.99999999999998579, 102.6397644303321215, -53.50000000000000711 ) ) ;
#25477=CARTESIAN_POINT ( 'NONE',  ( 112.9999999999999858, 97.00000000000000000, -13.00000000000000711 ) ) ;
#25480=CARTESIAN_POINT ( 'NONE',  ( 93.46109445667491400, 114.7507929638356785, -47.57500000273119412 ) ) ;
#25482=CARTESIAN_POINT ( 'NONE',  ( 98.53841926354351699, 123.0500000010924850, -1.461580736456474794 ) ) ;
#25490=CARTESIAN_POINT ( 'NONE',  ( 99.99999999999998579, 94.75000000000000000, 4.999999999999984013 ) ) ;
#25496=CARTESIAN_POINT ( 'NONE',  ( 102.1631189606246295, 116.6573956140660897, -47.10000000546237686 ) ) ;
#25499=EDGE_CURVE ( 'NONE', #13519, #5360, #7308, .T. ) ;
#25502=EDGE_CURVE ( 'NONE', #756, #12986, #26570, .T. ) ;
#25505=CARTESIAN_POINT ( 'NONE',  ( 101.8468681455907330, 95.12499999863439371, 4.458734124999980786 ) ) ;
#25514=CARTESIAN_POINT ( 'NONE',  ( 93.00000000000001421, 107.7255621263696668, -48.40000000546238113 ) ) ;
#25515=CARTESIAN_POINT ( 'NONE',  ( 96.84719886470463734, 90.93749999863440792, 3.152801135295351997 ) ) ;
#25516=CARTESIAN_POINT ( 'NONE',  ( 104.4587341249999781, 90.43749999863440792, -6.938893903907228378E-15 ) ) ;
#25519=ADVANCED_FACE ( 'NONE', ( #7022 ), #15717, .F. ) ;
#25523=ORIENTED_EDGE ( 'NONE', *, *, #17696, .T. ) ;
#25529=CARTESIAN_POINT ( 'NONE',  ( 95.00472066334982912, 116.8754121666685393, -49.67500000273118843 ) ) ;
#25532=EDGE_CURVE ( 'NONE', #11020, #10899, #749, .T. ) ;
#25534=LINE ( 'NONE', #8276, #2584 ) ;
#25540=CARTESIAN_POINT ( 'NONE',  ( 84.99999999999998579, 125.0000000000000000, -15.00000000000000888 ) ) ;
#25541=EDGE_CURVE ( 'NONE', #28082, #26002, #13714, .T. ) ;
#25549=EDGE_CURVE ( 'NONE', #24847, #1889, #11290, .T. ) ;
#25553=CARTESIAN_POINT ( 'NONE',  ( 100.8561741729129295, 123.5000000010924879, -2.066987299999998751 ) ) ;
#25554=CARTESIAN_POINT ( 'NONE',  ( 84.99999999999998579, 123.0000000000000000, 12.99999999999999112 ) ) ;
#25558=ORIENTED_EDGE ( 'NONE', *, *, #16966, .T. ) ;
#25568=EDGE_CURVE ( 'NONE', #27080, #11152, #27714, .T. ) ;
#25596=CARTESIAN_POINT ( 'NONE',  ( 98.96446609406727646, 123.5499999999999972, 2.499999999999977796 ) ) ;
#25598=CARTESIAN_POINT ( 'NONE',  ( 102.0669873000000081, 124.4000000010924651, -0.8561741729129508371 ) ) ;
#25602=CARTESIAN_POINT ( 'NONE',  ( 102.1631189606246295, 103.3426043859339103, -53.40000000000001279 ) ) ;
#25610=CARTESIAN_POINT ( 'NONE',  ( 93.46109445667491400, 105.2492070361643215, -51.17500000273119554 ) ) ;
#25613=EDGE_LOOP ( 'NONE', ( #12387, #19833, #27547, #25217 ) ) ;
#25614=CARTESIAN_POINT ( 'NONE',  ( 102.0669872999999797, 123.5500000010924708, -9.794112055954760458E-15 ) ) ;
#25620=EDGE_CURVE ( 'NONE', #13072, #6002, #19704, .T. ) ;
#25628=VECTOR ( 'NONE', #9734, 1000.000000000000000 ) ;
#25630=CARTESIAN_POINT ( 'NONE',  ( 102.1631189606246295, 116.6573956140660897, -52.60000000000000853 ) ) ;
#25635=CARTESIAN_POINT ( 'NONE',  ( 101.8468681455907330, 93.49999999863440792, -4.458734124999994997 ) ) ;
#25645=CARTESIAN_POINT ( 'NONE',  ( 95.54126587499999346, 94.12499999863439371, 1.846868145590722543 ) ) ;
#25652=CARTESIAN_POINT ( 'NONE',  ( 95.54126587499999346, 91.74999999863439371, -1.846868145590737864 ) ) ;
#25660=VERTEX_POINT ( 'NONE', #11997 ) ;
#25673=CARTESIAN_POINT ( 'NONE',  ( 100.0000000000000000, 110.0000000000000000, -55.00000000000000711 ) ) ;
#25682=ORIENTED_EDGE ( 'NONE', *, *, #18560, .T. ) ;
#25685=DIRECTION ( 'NONE',  ( 0.000000000000000000, 0.000000000000000000, -1.000000000000000000 ) ) ;
#25688=EDGE_CURVE ( 'NONE', #14776, #25390, #7600, .T. ) ;
#25694=VERTEX_POINT ( 'NONE', #10423 ) ;
#25695=CARTESIAN_POINT ( 'NONE',  ( 102.1631189606246295, 116.6573956140660897, -52.60000000000000853 ) ) ;
#25708=ORIENTED_EDGE ( 'NONE', *, *, #7065, .F. ) ;
#25711=EDGE_CURVE ( 'NONE', #14663, #19205, #21000, .T. ) ;
#25713=CYLINDRICAL_SURFACE ( 'NONE', #18068, 2.999999999999989786 ) ;
#25714=DIRECTION ( 'NONE',  ( -1.000000000000000000, 0.000000000000000000, -0.000000000000000000 ) ) ;
#25735=CARTESIAN_POINT ( 'NONE',  ( 97.50000000000000000, 123.3569999999781572, -1.035533905932742416 ) ) ;
#25737=CARTESIAN_POINT ( 'NONE',  ( 97.93301270000000613, 124.7000000010924765, -0.8561741729129506151 ) ) ;
#25751=CARTESIAN_POINT ( 'NONE',  ( 97.50236033167492167, 117.6869444889999841, -49.77500000273119696 ) ) ;
#25753=CARTESIAN_POINT ( 'NONE',  ( 97.93301269999999192, 124.7000000010924623, -0.8561741729129505041 ) ) ;
#25754=FACE_OUTER_BOUND ( 'NONE', #7421, .T. ) ;
#25773=LINE ( 'NONE', #26196, #7687 ) ;
#25774=CARTESIAN_POINT ( 'NONE',  ( 104.4587341249999923, 94.37499999863440792, -1.846868145590737198 ) ) ;
#25777=VECTOR ( 'NONE', #12816, 1000.000000000000000 ) ;
#25785=CARTESIAN_POINT ( 'NONE',  ( 96.84719886470463734, 94.68749999863440792, -3.152801135295366208 ) ) ;
#25797=VECTOR ( 'NONE', #21267, 999.9999999999997726 ) ;
#25816=CARTESIAN_POINT ( 'NONE',  ( 104.3262379212492590, 115.9545556584642867, -46.69999999999999574 ) ) ;
#25818=CARTESIAN_POINT ( 'NONE',  ( 104.9952793366501851, 103.1245878333314323, -52.42500000273119554 ) ) ;
#25821=CARTESIAN_POINT ( 'NONE',  ( 112.9999999999999858, 100.0000000000000000, -13.00000000000000711 ) ) ;
#25837=ORIENTED_EDGE ( 'NONE', *, *, #24542, .F. ) ;
#25838=CARTESIAN_POINT ( 'NONE',  ( 104.3262379212492590, 104.0454443415356991, -49.30000000000000426 ) ) ;
#25840=CARTESIAN_POINT ( 'NONE',  ( 104.9999999999999858, 92.87499999726881583, -6.938893903907228378E-15 ) ) ;
#25860=CARTESIAN_POINT ( 'NONE',  ( 107.0000000000000142, 110.0000000000000000, -55.00000000000000711 ) ) ;
#25864=ORIENTED_EDGE ( 'NONE', *, *, #21145, .F. ) ;
#25882=CARTESIAN_POINT ( 'NONE',  ( 98.96446609406727646, 122.5500000021849587, -2.499999999999997780 ) ) ;
#25891=DIRECTION ( 'NONE',  ( 0.000000000000000000, 0.000000000000000000, 1.000000000000000000 ) ) ;
#25894=DIRECTION ( 'NONE',  ( 0.000000000000000000, -0.000000000000000000, -1.000000000000000000 ) ) ;
#25897=CARTESIAN_POINT ( 'NONE',  ( 93.46109445667491400, 105.2492070361643215, -52.92500000273119554 ) ) ;
#25911=AXIS2_PLACEMENT_3D ( 'NONE', #4062, #18876, #3782 ) ;
#25929=CYLINDRICAL_SURFACE ( 'NONE', #25954, 7.000000000000006217 ) ;
#25930=CARTESIAN_POINT ( 'NONE',  ( 101.8468681455907330, 92.12499999863437949, 4.458734124999979898 ) ) ;
#25933=CARTESIAN_POINT ( 'NONE',  ( 107.0000000000000142, 107.7255621263696526, -45.10000000000000853 ) ) ;
#25934=ORIENTED_EDGE ( 'NONE', *, *, #18560, .F. ) ;
#25936=CARTESIAN_POINT ( 'NONE',  ( 96.84719886470463734, 92.68749999863440792, -3.152801135295366208 ) ) ;
#25937=ORIENTED_EDGE ( 'NONE', *, *, #11586, .F. ) ;
#25938=AXIS2_PLACEMENT_3D ( 'NONE', #3477, #20867, #1351 ) ;
#25951=CARTESIAN_POINT ( 'NONE',  ( 107.0000000000000142, 110.0000000000000000, -51.00000000000000711 ) ) ;
#25954=AXIS2_PLACEMENT_3D ( 'NONE', #27934, #2135, #6404 ) ;
#25960=AXIS2_PLACEMENT_3D ( 'NONE', #21757, #19604, #23884 ) ;
#25962=CARTESIAN_POINT ( 'NONE',  ( 91.91746824999998466, 112.6261737610028320, -51.22500000273119980 ) ) ;
#25970=CARTESIAN_POINT ( 'NONE',  ( 97.93301270000000613, 123.0000000010925021, 0.8561741729129328515 ) ) ;
#25971=FACE_OUTER_BOUND ( 'NONE', #7532, .T. ) ;
#25976=CYLINDRICAL_SURFACE ( 'NONE', #14684, 7.000000000000006217 ) ;
#25980=CARTESIAN_POINT ( 'NONE',  ( 104.3262379212492590, 115.9545556584642867, -50.70000000000000284 ) ) ;
#25983=CARTESIAN_POINT ( 'NONE',  ( 97.93301270000000613, 123.1500000010924651, -9.540979117872439019E-15 ) ) ;
#25991=ORIENTED_EDGE ( 'NONE', *, *, #12644, .F. ) ;
#25998=DIRECTION ( 'NONE',  ( 0.000000000000000000, 0.000000000000000000, -1.000000000000000000 ) ) ;
#26002=VERTEX_POINT ( 'NONE', #18042 ) ;
#26010=CARTESIAN_POINT ( 'NONE',  ( 107.0000000000000142, 107.7255621263696526, -45.60000000546237686 ) ) ;
#26015=DIRECTION ( 'NONE',  ( 0.000000000000000000, 0.000000000000000000, -1.000000000000000000 ) ) ;
#26023=CARTESIAN_POINT ( 'NONE',  ( 102.0669872999999939, 124.2000000010924907, -0.8561741729129507261 ) ) ;
#26025=DIRECTION ( 'NONE',  ( -0.000000000000000000, 1.000000000000000000, -0.000000000000000000 ) ) ;
#26030=CARTESIAN_POINT ( 'NONE',  ( 99.99999999999998579, 118.4984768113314004, -51.62500000273119127 ) ) ;
#26031=CYLINDRICAL_SURFACE ( 'NONE', #20524, 9.000000000000007105 ) ;
#26032=( BOUNDED_CURVE ( )  B_SPLINE_CURVE ( 2, ( #5494, #1502, #10155, #24875, #3349 ),
 .UNSPECIFIED., .F., .F. ) 
 B_SPLINE_CURVE_WITH_KNOTS ( ( 3, 2, 3 ),
 ( 0.000000000000000000, 0.02500000000000002220, 0.05000000000000004441 ),
 .UNSPECIFIED. ) 
 CURVE ( )  GEOMETRIC_REPRESENTATION_ITEM ( )  RATIONAL_B_SPLINE_CURVE ( ( 1.000000000000000000, 0.9238795325112867385, 1.000000000000000000, 0.9238795325112866275, 1.000000000000000222 ) ) 
 REPRESENTATION_ITEM ( '' )  );
#26062=CARTESIAN_POINT ( 'NONE',  ( 93.46109445667491400, 105.2492070361643215, -45.17500000273119554 ) ) ;
#26067=CARTESIAN_POINT ( 'NONE',  ( 101.8468681455907330, 91.49999999863440792, -4.458734124999994997 ) ) ;
#26071=ORIENTED_EDGE ( 'NONE', *, *, #24275, .T. ) ;
#26073=CARTESIAN_POINT ( 'NONE',  ( 104.4587341249999781, 94.31249999863440792, -6.938893903907228378E-15 ) ) ;
#26076=AXIS2_PLACEMENT_3D ( 'NONE', #5048, #2903, #18441 ) ;
#26080=ORIENTED_EDGE ( 'NONE', *, *, #20686, .F. ) ;
#26108=VERTEX_POINT ( 'NONE', #22763 ) ;
#26111=DIRECTION ( 'NONE',  ( 1.000000000000000000, 0.000000000000000000, 0.000000000000000000 ) ) ;
#26113=( BOUNDED_CURVE ( )  B_SPLINE_CURVE ( 2, ( #14918, #8105, #4115, #23774, #25496, #1847, #8239, #10783, #10509, #23227, #19215 ),
 .UNSPECIFIED., .F., .T. ) 
 B_SPLINE_CURVE_WITH_KNOTS ( ( 3, 2, 2, 2, 2, 3 ),
 ( 0.5999999999999998668, 0.6199999999999998845, 0.6399999999999999023, 0.6599999999999999201, 0.6799999999999999378, 0.6999999999999998446 ),
 .UNSPECIFIED. ) 
 CURVE ( )  GEOMETRIC_REPRESENTATION_ITEM ( )  RATIONAL_B_SPLINE_CURVE ( ( 1.000000000000000222, 0.9510565162951533091, 1.000000000000000000, 0.9510565162951535312, 1.000000000000000000, 0.9510565162951535312, 1.000000000000000000, 0.9510565162951535312, 1.000000000000000000, 0.9510565162951537532, 0.9999999999999997780 ) ) 
 REPRESENTATION_ITEM ( '' )  );
#26118=ORIENTED_EDGE ( 'NONE', *, *, #13074, .F. ) ;
#26119=CARTESIAN_POINT ( 'NONE',  ( 107.0000000000000142, 112.2744378736303332, -48.90000000000000568 ) ) ;
#26121=CARTESIAN_POINT ( 'NONE',  ( 101.4615807364564546, 123.4500000010924765, 1.461580736456455476 ) ) ;
#26124=CARTESIAN_POINT ( 'NONE',  ( 102.0710678118654613, 92.68749999726883004, 4.999999999999983125 ) ) ;
#26126=CARTESIAN_POINT ( 'NONE',  ( 84.99999999999998579, 118.0000000000000000, -13.00000000000000711 ) ) ;
#26127=ORIENTED_EDGE ( 'NONE', *, *, #23963, .T. ) ;
#26130=ADVANCED_FACE ( 'NONE', ( #7638 ), #6388, .T. ) ;
#26142=ORIENTED_EDGE ( 'NONE', *, *, #4985, .F. ) ;
#26155=CARTESIAN_POINT ( 'NONE',  ( 91.91746824999999887, 110.0000000000000000, -51.12500000273119127 ) ) ;
#26165=CARTESIAN_POINT ( 'NONE',  ( 98.96446609406727646, 123.3500000021849701, -2.499999999999997780 ) ) ;
#26167=CYLINDRICAL_SURFACE ( 'NONE', #12291, 4.999999999999989342 ) ;
#26172=CARTESIAN_POINT ( 'NONE',  ( 106.5389055433251002, 105.2492070361643215, -52.32500000273119412 ) ) ;
#26184=VECTOR ( 'NONE', #5984, 1000.000000000000000 ) ;
#26185=DIRECTION ( 'NONE',  ( -1.000000000000000000, 0.000000000000000000, 0.000000000000000000 ) ) ;
#26196=CARTESIAN_POINT ( 'NONE',  ( 87.00000000000000000, 100.0000000000000000, -13.00000000000000533 ) ) ;
#26205=CARTESIAN_POINT ( 'NONE',  ( 102.4976396683250925, 102.3130555110000159, -46.77500000273119696 ) ) ;
#26206=CARTESIAN_POINT ( 'NONE',  ( 99.99999988184244160, 117.0000000000000000, -45.00000000000000711 ) ) ;
#26208=EDGE_CURVE ( 'NONE', #20844, #5424, #18088, .T. ) ;
#26210=LINE ( 'NONE', #12512, #21 ) ;
#26211=CARTESIAN_POINT ( 'NONE',  ( 99.99999999999998579, 91.56249999863440792, -4.458734124999994997 ) ) ;
#26212=CARTESIAN_POINT ( 'NONE',  ( 97.92893218813455292, 93.56249999726884425, 5.000000000000011546 ) ) ;
#26221=CARTESIAN_POINT ( 'NONE',  ( 99.99999999999998579, 93.06249999863440792, 4.458734124999981674 ) ) ;
#26247=CARTESIAN_POINT ( 'NONE',  ( 108.0825317500000011, 112.6261737610028320, -50.02500000273118275 ) ) ;
#26248=CARTESIAN_POINT ( 'NONE',  ( 102.4999999999999858, 123.8500000000000085, -1.035533905932742638 ) ) ;
#26258=DIRECTION ( 'NONE',  ( 0.000000000000000000, -1.000000000000000000, 0.000000000000000000 ) ) ;
#26261=ORIENTED_EDGE ( 'NONE', *, *, #18000, .F. ) ;
#26264=ORIENTED_EDGE ( 'NONE', *, *, #23963, .F. ) ;
#26265=CARTESIAN_POINT ( 'NONE',  ( 105.6631189606246295, 114.1144967660473242, -52.80000000000000426 ) ) ;
#26267=CARTESIAN_POINT ( 'NONE',  ( 102.0669872999999939, 124.4000000010924651, -0.8561741729129507261 ) ) ;
#26270=CARTESIAN_POINT ( 'NONE',  ( 102.0710678118654613, 92.06249999726880162, -4.999999999999997335 ) ) ;
#26286=DIRECTION ( 'NONE',  ( 5.782411586589357392E-17, 3.469446951953611231E-16, 1.000000000000000000 ) ) ;
#26288=CARTESIAN_POINT ( 'NONE',  ( 97.83688103937537051, 103.3426043859339103, -49.60000000000000853 ) ) ;
#26306=CARTESIAN_POINT ( 'NONE',  ( 97.50000000000000000, 123.5000000021849615, -9.540979117872439019E-15 ) ) ;
#26312=CARTESIAN_POINT ( 'NONE',  ( 97.93301269999999192, 124.5000000010924879, -0.8561741729129505041 ) ) ;
#26320=CARTESIAN_POINT ( 'NONE',  ( 93.46109445667491400, 105.2492070361643215, -45.17500000273119554 ) ) ;
#26328=CARTESIAN_POINT ( 'NONE',  ( 99.99999999999998579, 124.0000000000000000, -2.499999999999997780 ) ) ;
#26338=VECTOR ( 'NONE', #19247, 1000.000000000000000 ) ;
#26344=PLANE ( 'NONE',  #7759 ) ;
#26355=CARTESIAN_POINT ( 'NONE',  ( 104.4587341249999781, 95.56249999863440792, -6.938893903907228378E-15 ) ) ;
#26358=CARTESIAN_POINT ( 'NONE',  ( 99.95774716806533888, 123.0000000000000426, 2.503702194450118323 ) ) ;
#26366=CARTESIAN_POINT ( 'NONE',  ( 101.8468681455907330, 92.12499999863437949, 4.458734124999979898 ) ) ;
#26377=ORIENTED_EDGE ( 'NONE', *, *, #19400, .T. ) ;
#26395=CARTESIAN_POINT ( 'NONE',  ( 108.0825317500000011, 107.3738262389971538, -44.22500000273118559 ) ) ;
#26396=DIRECTION ( 'NONE',  ( 0.000000000000000000, -1.000000000000000000, 0.000000000000000000 ) ) ;
#26401=CARTESIAN_POINT ( 'NONE',  ( 93.00000000000000000, 110.0000000000000000, -46.50000000546238255 ) ) ;
#26403=DIRECTION ( 'NONE',  ( 5.782411586589357392E-17, -0.000000000000000000, 1.000000000000000000 ) ) ;
#26407=DIRECTION ( 'NONE',  ( 5.782411586589357392E-17, -0.000000000000000000, 1.000000000000000000 ) ) ;
#26411=CARTESIAN_POINT ( 'NONE',  ( 91.91746824999998466, 107.3738262389971538, -51.27500000273119696 ) ) ;
#26413=CARTESIAN_POINT ( 'NONE',  ( 102.4999999999999716, 123.0500000000000114, -1.035533905932742638 ) ) ;
#26414=EDGE_CURVE ( 'NONE', #19519, #21081, #11125, .T. ) ;
#26417=CARTESIAN_POINT ( 'NONE',  ( 104.9999999999999716, 93.93749999726881583, -2.071067811865478170 ) ) ;
#26424=ORIENTED_EDGE ( 'NONE', *, *, #24827, .T. ) ;
#26432=CARTESIAN_POINT ( 'NONE',  ( 96.84719886470463734, 91.18749999863440792, 3.152801135295351997 ) ) ;
#26442=ORIENTED_EDGE ( 'NONE', *, *, #9550, .T. ) ;
#26449=CARTESIAN_POINT ( 'NONE',  ( 108.0825317500000011, 112.6261737610028320, -54.02500000273118985 ) ) ;
#26451=CARTESIAN_POINT ( 'NONE',  ( 98.23223304703363112, 124.2000000021849502, -1.767766952966370209 ) ) ;
#26459=CARTESIAN_POINT ( 'NONE',  ( 99.14382582708707048, 123.6000000010924680, -2.066987299999999195 ) ) ;
#26466=CARTESIAN_POINT ( 'NONE',  ( 104.9952793366501851, 116.8754121666685393, -51.82500000273120122 ) ) ;
#26502=CARTESIAN_POINT ( 'NONE',  ( 100.7645585624018025, 123.0000000000000426, -2.384778589250489578 ) ) ;
#26503=VERTEX_POINT ( 'NONE', #13114 ) ;
#26511=CARTESIAN_POINT ( 'NONE',  ( 101.8468681455907330, 92.49999999863442213, -4.458734124999994997 ) ) ;
#26512=CARTESIAN_POINT ( 'NONE',  ( 101.8468681455907330, 95.37499999863440792, 4.458734124999979898 ) ) ;
#26522=ORIENTED_EDGE ( 'NONE', *, *, #21332, .F. ) ;
#26528=CARTESIAN_POINT ( 'NONE',  ( 97.83688103937537051, 103.3426043859339103, -50.10000000546237686 ) ) ;
#26534=CARTESIAN_POINT ( 'NONE',  ( 93.46109445667491400, 114.7507929638356785, -45.32500000273119412 ) ) ;
#26545=DIRECTION ( 'NONE',  ( -0.000000000000000000, 1.000000000000000000, -0.000000000000000000 ) ) ;
#26547=ORIENTED_EDGE ( 'NONE', *, *, #20938, .T. ) ;
#26551=CARTESIAN_POINT ( 'NONE',  ( 97.83688103937538472, 116.6573956140660897, -46.40000000000001279 ) ) ;
#26553=CARTESIAN_POINT ( 'NONE',  ( 102.4999999999999858, 123.0000000000000000, -9.847140817659276890E-15 ) ) ;
#26557=ADVANCED_FACE ( 'NONE', ( #12975 ), #25976, .T. ) ;
#26559=CARTESIAN_POINT ( 'NONE',  ( 97.92893218813452449, 93.56249999726883004, 4.999999999999983125 ) ) ;
#26562=CARTESIAN_POINT ( 'NONE',  ( 99.99999999999998579, 118.4984768113314146, -53.87500000273119127 ) ) ;
#26568=EDGE_CURVE ( 'NONE', #1189, #28194, #6447, .T. ) ;
#26570=LINE ( 'NONE', #18148, #21525 ) ;
#26593=CARTESIAN_POINT ( 'NONE',  ( 108.0825317500000011, 112.6261737610028320, -52.02500000273118985 ) ) ;
#26595=CARTESIAN_POINT ( 'NONE',  ( 99.99999999999998579, 93.62499999726881583, 4.999999999999984013 ) ) ;
#26599=VERTEX_POINT ( 'NONE', #20310 ) ;
#26602=CARTESIAN_POINT ( 'NONE',  ( 100.8561741729129153, 122.7000000010924623, -2.066987299999999195 ) ) ;
#26610=CARTESIAN_POINT ( 'NONE',  ( 93.46109445667491400, 114.7507929638356785, -47.32500000273119412 ) ) ;
#26612=EDGE_CURVE ( 'NONE', #10899, #26599, #26806, .T. ) ;
#26613=CARTESIAN_POINT ( 'NONE',  ( 107.0000000000000284, 112.2744378736302906, -49.40000000546238113 ) ) ;
#26633=CARTESIAN_POINT ( 'NONE',  ( 114.9999999999999858, 125.0000000000000000, -15.00000000000001066 ) ) ;
#26634=CARTESIAN_POINT ( 'NONE',  ( 97.50000000000000000, 125.0254775906283697, 0.3826834323650784575 ) ) ;
#26648=CARTESIAN_POINT ( 'NONE',  ( 108.0825317500000011, 112.6261737610028320, -54.27500000273118275 ) ) ;
#26649=CARTESIAN_POINT ( 'NONE',  ( 98.07597603534063069, 122.9999999999999858, 1.603032847902431612 ) ) ;
#26650=CARTESIAN_POINT ( 'NONE',  ( 101.4615807364564546, 123.4500000010924765, -1.461580736456474794 ) ) ;
#26658=CARTESIAN_POINT ( 'NONE',  ( 95.00000000000000000, 93.50000000000000000, -7.551217303480904118E-15 ) ) ;
#26664=CARTESIAN_POINT ( 'NONE',  ( 93.00000000000000000, 110.0000000000000000, -50.50000000546237544 ) ) ;
#26669=EDGE_LOOP ( 'NONE', ( #8160, #7791, #3213, #11519 ) ) ;
#26674=DIRECTION ( 'NONE',  ( 5.782411586589357392E-17, -0.000000000000000000, 1.000000000000000000 ) ) ;
#26676=CARTESIAN_POINT ( 'NONE',  ( 102.0710678118654755, 91.81250000000000000, 4.999999999999961808 ) ) ;
#26679=CARTESIAN_POINT ( 'NONE',  ( 99.99999999999998579, 95.00000000000000000, -6.938893903907228378E-15 ) ) ;
#26681=CARTESIAN_POINT ( 'NONE',  ( 93.46109445667491400, 105.2492070361643215, -48.92500000273119554 ) ) ;
#26682=CARTESIAN_POINT ( 'NONE',  ( 98.15313185440925281, 91.87499999863439371, -4.458734124999994997 ) ) ;
#26689=CARTESIAN_POINT ( 'NONE',  ( 97.92893218813455292, 91.68749999999997158, 5.000000000000003553 ) ) ;
#26696=CARTESIAN_POINT ( 'NONE',  ( 91.91746824999998466, 107.3738262389971538, -53.27500000273119696 ) ) ;
#26703=CARTESIAN_POINT ( 'NONE',  ( 99.99999999999998579, 92.62499999726881583, 4.999999999999984013 ) ) ;
#26706=CARTESIAN_POINT ( 'NONE',  ( 93.46109445667491400, 105.2492070361643215, -49.17500000273119554 ) ) ;
#26714=DIRECTION ( 'NONE',  ( -0.000000000000000000, 1.000000000000000000, -0.000000000000000000 ) ) ;
#26719=CARTESIAN_POINT ( 'NONE',  ( 98.15313185440923860, 90.87499999863439371, -4.458734124999994997 ) ) ;
#26734=ADVANCED_FACE ( 'NONE', ( #10294, #27851 ), #16997, .T. ) ;
#26736=CARTESIAN_POINT ( 'NONE',  ( 91.91746824999999887, 110.0000000000000000, -49.12500000273119838 ) ) ;
#26737=ADVANCED_FACE ( 'NONE', ( #10024 ), #18733, .F. ) ;
#26751=CARTESIAN_POINT ( 'NONE',  ( 98.15313185440925281, 91.99999999863439371, 4.458734124999979898 ) ) ;
#26755=CARTESIAN_POINT ( 'NONE',  ( 95.67376207875072680, 115.9545556584642867, -48.80000000546237260 ) ) ;
#26768=( BOUNDED_CURVE ( )  B_SPLINE_CURVE ( 2, ( #15401, #13250, #21982, #2458, #10703, #19409, #13396, #11120, #6574, #23975, #19834 ),
 .UNSPECIFIED., .F., .F. ) 
 B_SPLINE_CURVE_WITH_KNOTS ( ( 3, 2, 2, 2, 2, 3 ),
 ( 0.2000000000000001776, 0.2200000000000001676, 0.2400000000000001854, 0.2600000000000002309, 0.2800000000000002487, 0.3000000000000002109 ),
 .UNSPECIFIED. ) 
 CURVE ( )  GEOMETRIC_REPRESENTATION_ITEM ( )  RATIONAL_B_SPLINE_CURVE ( ( 0.9999999999999995559, 0.9510565162951539753, 1.000000000000000000, 0.9510565162951535312, 1.000000000000000000, 0.9510565162951535312, 1.000000000000000000, 0.9510565162951535312, 1.000000000000000000, 0.9510565162951529761, 1.000000000000000444 ) ) 
 REPRESENTATION_ITEM ( '' )  );
#26771=CARTESIAN_POINT ( 'NONE',  ( 102.4999999999999858, 123.8500000021849416, 1.035533905932722876 ) ) ;
#26781=PLANE ( 'NONE',  #11475 ) ;
#26791=CARTESIAN_POINT ( 'NONE',  ( 108.0825317500000011, 112.6261737610028320, -52.27500000273118985 ) ) ;
#26792=CARTESIAN_POINT ( 'NONE',  ( 99.53100023034451738, 122.9999999999999716, 2.460289198665830401 ) ) ;
#26793=CARTESIAN_POINT ( 'NONE',  ( 98.53841926354351699, 124.4500000010924765, -1.461580736456474794 ) ) ;
#26799=CARTESIAN_POINT ( 'NONE',  ( 104.9999999999999716, 93.93749999999998579, 2.071067811865467956 ) ) ;
#26806=( BOUNDED_CURVE ( )  B_SPLINE_CURVE ( 2, ( #27022, #22878, #25013, #11590, #1082, #7177, #3205, #14298, #796 ),
 .UNSPECIFIED., .F., .F. ) 
 B_SPLINE_CURVE_WITH_KNOTS ( ( 3, 2, 2, 2, 3 ),
 ( 0.05000000000000004441, 0.07500000000000006661, 0.1000000000000000888, 0.1250000000000001110, 0.1500000000000001332 ),
 .UNSPECIFIED. ) 
 CURVE ( )  GEOMETRIC_REPRESENTATION_ITEM ( )  RATIONAL_B_SPLINE_CURVE ( ( 0.9999999999999998890, 0.9238795325112868495, 1.000000000000000000, 0.9238795325112867385, 1.000000000000000000, 0.9238795325112867385, 1.000000000000000000, 0.9238795325112862944, 1.000000000000000444 ) ) 
 REPRESENTATION_ITEM ( '' )  );
#26810=SHAPE_REPRESENTATION ( 'vaccum generator', ( #26844 ), #4064 ) ;
#26819=CARTESIAN_POINT ( 'NONE',  ( 99.99999999999998579, 102.6397644303321215, -50.00000000546236834 ) ) ;
#26821=CARTESIAN_POINT ( 'NONE',  ( 100.0000000000000000, 110.0000000000000000, -55.00000000000000711 ) ) ;
#26826=LINE ( 'NONE', #2313, #27194 ) ;
#26828=CARTESIAN_POINT ( 'NONE',  ( 94.33688103937537051, 105.8855032339526758, -52.30000000546237970 ) ) ;
#26829=VECTOR ( 'NONE', #17787, 1000.000000000000000 ) ;
#26830=CARTESIAN_POINT ( 'NONE',  ( 101.8468681455907330, 90.74999999863439371, -4.458734124999994997 ) ) ;
#26831=CARTESIAN_POINT ( 'NONE',  ( 99.99999999999998579, 95.00000000000000000, -6.938893903907228378E-15 ) ) ;
#26842=CARTESIAN_POINT ( 'NONE',  ( 102.4976396683250925, 102.3130555110000159, -50.77500000273119696 ) ) ;
#26844=AXIS2_PLACEMENT_3D ( 'NONE', #8635, #24028, #23608 ) ;
#26845=CARTESIAN_POINT ( 'NONE',  ( 97.50000000000000000, 123.4500000000000028, 1.035533905932725096 ) ) ;
#26852=CARTESIAN_POINT ( 'NONE',  ( 103.1528011352953484, 91.68749999863440792, -3.152801135295366208 ) ) ;
#26854=CARTESIAN_POINT ( 'NONE',  ( 102.4976396683250925, 102.3130555110000159, -52.77500000273119696 ) ) ;
#26862=CARTESIAN_POINT ( 'NONE',  ( 101.0355339059327378, 124.7500000000000284, -2.499999999999988010 ) ) ;
#26883=CARTESIAN_POINT ( 'NONE',  ( 95.00472066334981491, 116.8754121666685393, -49.42500000273118843 ) ) ;
#26885=LINE ( 'NONE', #16019, #21500 ) ;
#26896=CARTESIAN_POINT ( 'NONE',  ( 97.50236033167492167, 102.3130555110000159, -44.72500000273119980 ) ) ;
#26897=LINE ( 'NONE', #1239, #15936 ) ;
#26914=CARTESIAN_POINT ( 'NONE',  ( 101.0355339059327093, 124.0500000021849445, -2.500000000000002665 ) ) ;
#26916=AXIS2_PLACEMENT_3D ( 'NONE', #19741, #11031, #13446 ) ;
#26936=CARTESIAN_POINT ( 'NONE',  ( 95.00000000000000000, 90.43750000000000000, -2.071067811865479058 ) ) ;
#26937=CARTESIAN_POINT ( 'NONE',  ( 98.38094258238263023, 122.9999999999999716, 1.910582039389197684 ) ) ;
#26946=CARTESIAN_POINT ( 'NONE',  ( 102.0710678118654613, 93.81250000000000000, 4.999999999999983125 ) ) ;
#26952=EDGE_LOOP ( 'NONE', ( #3145, #26127, #22976, #14296, #9774, #1208, #21630, #1454, #24447, #22984, #17881, #9756, #4225, #9958 ) ) ;
#26964=CARTESIAN_POINT ( 'NONE',  ( 98.15313185440923860, 90.62499999863439371, -4.458734124999994997 ) ) ;
#26965=DIRECTION ( 'NONE',  ( -1.000000000000000000, 0.000000000000000000, 0.000000000000000000 ) ) ;
#26969=CARTESIAN_POINT ( 'NONE',  ( 94.33688103937537051, 114.1144967660473242, -52.70000000546237828 ) ) ;
#26971=CARTESIAN_POINT ( 'NONE',  ( 95.00472066334982912, 116.8754121666685393, -47.42500000273118843 ) ) ;
#26979=DIRECTION ( 'NONE',  ( -0.000000000000000000, -1.000000000000000000, -0.000000000000000000 ) ) ;
#26986=CARTESIAN_POINT ( 'NONE',  ( 94.33688103937537051, 105.8855032339526758, -45.80000000000000426 ) ) ;
#26988=CARTESIAN_POINT ( 'NONE',  ( 99.99999999999998579, 123.6000000000000085, 2.499999999999978684 ) ) ;
#26993=CARTESIAN_POINT ( 'NONE',  ( 96.84719886470463734, 90.93749999863440792, -3.152801135295366208 ) ) ;
#26995=CARTESIAN_POINT ( 'NONE',  ( 102.4976396683250925, 102.3130555110000159, -48.77500000273119696 ) ) ;
#27002=CARTESIAN_POINT ( 'NONE',  ( 101.7677669529663547, 124.7000000000000028, -1.767766952966370209 ) ) ;
#27007=CARTESIAN_POINT ( 'NONE',  ( 103.1528011352953484, 92.43749999863440792, 3.152801135295352886 ) ) ;
#27017=VECTOR ( 'NONE', #8443, 1000.000000000000000 ) ;
#27022=CARTESIAN_POINT ( 'NONE',  ( 99.99999999999998579, 91.12499999726880162, -4.999999999999997335 ) ) ;
#27025=CARTESIAN_POINT ( 'NONE',  ( 102.4976396683250925, 117.6869444889999841, -45.72500000273119269 ) ) ;
#27026=CARTESIAN_POINT ( 'NONE',  ( 84.99999999999998579, 95.00000000000000000, 14.99999999999999467 ) ) ;
#27030=SURFACE_SIDE_STYLE ('',( #14169 ) ) ;
#27035=DIRECTION ( 'NONE',  ( 5.782411586589357392E-17, -0.000000000000000000, 1.000000000000000000 ) ) ;
#27038=CARTESIAN_POINT ( 'NONE',  ( 104.9999999999999716, 91.81249999726880162, 2.071067811865467956 ) ) ;
#27039=CARTESIAN_POINT ( 'NONE',  ( 104.9952793366501851, 103.1245878333314323, -48.42500000273120264 ) ) ;
#27061=CARTESIAN_POINT ( 'NONE',  ( 102.4999999999999716, 123.8569999999781572, -1.035533905932742638 ) ) ;
#27075=DIRECTION ( 'NONE',  ( 0.000000000000000000, 0.000000000000000000, -1.000000000000000000 ) ) ;
#27080=VERTEX_POINT ( 'NONE', #2504 ) ;
#27084=CARTESIAN_POINT ( 'NONE',  ( 95.00000000000000000, 90.56250000000000000, 2.071067811865463959 ) ) ;
#27087=AXIS2_PLACEMENT_3D ( 'NONE', #897, #22407, #15832 ) ;
#27091=ORIENTED_EDGE ( 'NONE', *, *, #27721, .T. ) ;
#27102=EDGE_CURVE ( 'NONE', #14776, #19120, #24040, .T. ) ;
#27104=CARTESIAN_POINT ( 'NONE',  ( 101.8468681455907330, 92.49999999863440792, -4.458734124999994997 ) ) ;
#27112=CARTESIAN_POINT ( 'NONE',  ( 107.0000000000000142, 112.2744378736303332, -51.40000000546237402 ) ) ;
#27113=CARTESIAN_POINT ( 'NONE',  ( 99.99999999999998579, 90.81249999863440792, -4.458734124999994997 ) ) ;
#27117=ADVANCED_FACE ( 'NONE', ( #11394 ), #7407, .F. ) ;
#27120=PLANE ( 'NONE',  #27087 ) ;
#27121=LINE ( 'NONE', #9284, #7487 ) ;
#27126=ADVANCED_FACE ( 'NONE', ( #18106, #7266 ), #15956, .T. ) ;
#27128=CARTESIAN_POINT ( 'NONE',  ( 99.99999999999998579, 118.4984768113314004, -45.87500000273118417 ) ) ;
#27132=CARTESIAN_POINT ( 'NONE',  ( 100.0000000000000000, 110.0000000000000000, -55.00000000000000711 ) ) ;
#27137=CARTESIAN_POINT ( 'NONE',  ( 95.54126587500000767, 94.06249999863440792, -7.484931351350258973E-15 ) ) ;
#27139=CARTESIAN_POINT ( 'NONE',  ( 108.0825317500000011, 112.6261737610028320, -50.27500000273119696 ) ) ;
#27141=ORIENTED_EDGE ( 'NONE', *, *, #2547, .T. ) ;
#27153=CARTESIAN_POINT ( 'NONE',  ( 101.8468681455907330, 93.74999999863439371, -4.458734124999994997 ) ) ;
#27158=VECTOR ( 'NONE', #926, 1000.000000000000000 ) ;
#27160=DIRECTION ( 'NONE',  ( 0.000000000000000000, 0.000000000000000000, 1.000000000000000000 ) ) ;
#27162=CYLINDRICAL_SURFACE ( 'NONE', #510, 4.999999999999989342 ) ;
#27171=CARTESIAN_POINT ( 'NONE',  ( 98.89130886013153088, 116.9999999812857112, -44.94874572125286250 ) ) ;
#27172=PLANE ( 'NONE',  #3698 ) ;
#27175=PRESENTATION_STYLE_ASSIGNMENT (( #11742 ) ) ;
#27182=CARTESIAN_POINT ( 'NONE',  ( 103.5355339059327235, 91.99999999726880162, -3.535533905932738197 ) ) ;
#27183=CARTESIAN_POINT ( 'NONE',  ( 97.50236033167492167, 117.6869444889999841, -45.52500000273119696 ) ) ;
#27187=CARTESIAN_POINT ( 'NONE',  ( 95.00000000000000000, 91.31249999726878741, -2.071067811865479058 ) ) ;
#27194=VECTOR ( 'NONE', #4444, 1000.000000000000000 ) ;
#27215=DIRECTION ( 'NONE',  ( -1.000000000000000000, 0.000000000000000000, 0.000000000000000000 ) ) ;
#27218=CARTESIAN_POINT ( 'NONE',  ( 96.46446609406726225, 90.37500000000000000, -3.535533905932738197 ) ) ;
#27229=CARTESIAN_POINT ( 'NONE',  ( 95.00000000000000000, 92.43750000000001421, -2.071067811865479058 ) ) ;
#27251=CARTESIAN_POINT ( 'NONE',  ( 94.33688103937537051, 114.1144967660473242, -46.70000000546237828 ) ) ;
#27252=CARTESIAN_POINT ( 'NONE',  ( 103.1528011352953484, 94.43749999863440792, 3.152801135295352886 ) ) ;
#27267=CARTESIAN_POINT ( 'NONE',  ( 102.4976396683250925, 117.6869444889999841, -45.97500000273119269 ) ) ;
#27275=CARTESIAN_POINT ( 'NONE',  ( 104.4587341249999923, 90.62499999863439371, -1.846868145590737198 ) ) ;
#27276=CARTESIAN_POINT ( 'NONE',  ( 104.9999999999999858, 90.00000000000000000, -6.938893903907228378E-15 ) ) ;
#27288=CARTESIAN_POINT ( 'NONE',  ( 95.54126587499999346, 94.99999999863439371, -1.846868145590737864 ) ) ;
#27292=CARTESIAN_POINT ( 'NONE',  ( 97.92893218813455292, 93.68749999999998579, 5.000000000000023981 ) ) ;
#27303=CARTESIAN_POINT ( 'NONE',  ( 114.9999999999999858, 0.000000000000000000, -8.673617379884035472E-16 ) ) ;
#27307=CARTESIAN_POINT ( 'NONE',  ( 99.99999999999998579, 90.00000000000000000, -6.938893903907228378E-15 ) ) ;
#27311=FILL_AREA_STYLE ('',( #18323 ) ) ;
#27321=CARTESIAN_POINT ( 'NONE',  ( 93.00000000000000000, 110.0000000000000000, -48.50000000546238255 ) ) ;
#27332=CARTESIAN_POINT ( 'NONE',  ( 99.99999999999998579, 91.25000000000000000, -4.999999999999997335 ) ) ;
#27334=DIRECTION ( 'NONE',  ( 0.000000000000000000, 0.000000000000000000, -1.000000000000000000 ) ) ;
#27341=CARTESIAN_POINT ( 'NONE',  ( 101.0355339059327378, 123.1499999999999915, -2.499999999999997780 ) ) ;
#27344=VECTOR ( 'NONE', #18501, 1000.000000000000000 ) ;
#27349=DIRECTION ( 'NONE',  ( -0.000000000000000000, 1.000000000000000000, -0.000000000000000000 ) ) ;
#27358=CARTESIAN_POINT ( 'NONE',  ( 106.5389055433251002, 105.2492070361643215, -46.57500000273119412 ) ) ;
#27359=CARTESIAN_POINT ( 'NONE',  ( 97.93301270000000613, 123.1500000010924651, -9.540979117872439019E-15 ) ) ;
#27375=DIRECTION ( 'NONE',  ( -0.8660254037844392627, 0.000000000000000000, 0.4999999999999987788 ) ) ;
#27381=CARTESIAN_POINT ( 'NONE',  ( 104.4587341249999781, 95.31249999863440792, -6.938893903907228378E-15 ) ) ;
#27387=CARTESIAN_POINT ( 'NONE',  ( 97.83688103937538472, 116.6573956140660897, -52.90000000546237402 ) ) ;
#27389=CARTESIAN_POINT ( 'NONE',  ( 107.0000000000000142, 112.2744378736303332, -47.40000000546237402 ) ) ;
#27390=CARTESIAN_POINT ( 'NONE',  ( 99.99999999999998579, 93.31249999863440792, 4.458734124999981674 ) ) ;
#27392=CARTESIAN_POINT ( 'NONE',  ( 102.0669872999999797, 122.5500000010924850, -9.794112055954760458E-15 ) ) ;
#27396=FACE_OUTER_BOUND ( 'NONE', #26952, .T. ) ;
#27398=ORIENTED_EDGE ( 'NONE', *, *, #9167, .F. ) ;
#27402=CARTESIAN_POINT ( 'NONE',  ( 95.00472066334982912, 103.1245878333314323, -47.07500000273119412 ) ) ;
#27408=CARTESIAN_POINT ( 'NONE',  ( 103.1528011352953484, 92.43749999863440792, 3.152801135295352886 ) ) ;
#27419=CARTESIAN_POINT ( 'NONE',  ( 103.1528011352953484, 94.43749999863440792, 3.152801135295352886 ) ) ;
#27422=CARTESIAN_POINT ( 'NONE',  ( 95.00000000000000000, 93.50000000000000000, -7.551217303480904118E-15 ) ) ;
#27429=VERTEX_POINT ( 'NONE', #17070 ) ;
#27430=CARTESIAN_POINT ( 'NONE',  ( 102.1631189606246295, 116.6573956140660897, -54.60000000000000853 ) ) ;
#27434=CARTESIAN_POINT ( 'NONE',  ( 94.33688103937537051, 114.1144967660473242, -44.70000000546237828 ) ) ;
#27436=LINE ( 'NONE', #23434, #12309 ) ;
#27438=ORIENTED_EDGE ( 'NONE', *, *, #27513, .F. ) ;
#27441=( NAMED_UNIT ( * ) SI_UNIT ( $, .STERADIAN. ) SOLID_ANGLE_UNIT ( ) );
#27445=EDGE_CURVE ( 'NONE', #5424, #5694, #25773, .T. ) ;
#27447=DIRECTION ( 'NONE',  ( 0.000000000000000000, 0.000000000000000000, 1.000000000000000000 ) ) ;
#27452=CARTESIAN_POINT ( 'NONE',  ( 104.9999999999999716, 93.93749999726880162, -2.071067811865478170 ) ) ;
#27457=EDGE_LOOP ( 'NONE', ( #15400, #2034, #15133, #9354 ) ) ;
#27459=PRODUCT_DEFINITION_CONTEXT ( 'detailed design', #12763, 'design' ) ;
#27462=( BOUNDED_CURVE ( )  B_SPLINE_CURVE ( 2, ( #25296, #1375, #11752, #27038, #22471, #16462, #27182, #16327, #3223 ),
 .UNSPECIFIED., .F., .T. ) 
 B_SPLINE_CURVE_WITH_KNOTS ( ( 3, 2, 2, 2, 3 ),
 ( 0.1500000000000001332, 0.1750000000000001554, 0.2000000000000001776, 0.2250000000000001998, 0.2500000000000002220 ),
 .UNSPECIFIED. ) 
 CURVE ( )  GEOMETRIC_REPRESENTATION_ITEM ( )  RATIONAL_B_SPLINE_CURVE ( ( 0.9999999999999995559, 0.9238795325112871826, 1.000000000000000000, 0.9238795325112867385, 1.000000000000000000, 0.9238795325112867385, 1.000000000000000000, 0.9238795325112860723, 1.000000000000000666 ) ) 
 REPRESENTATION_ITEM ( '' )  );
#27470=DIRECTION ( 'NONE',  ( 0.000000000000000000, 0.000000000000000000, 1.000000000000000000 ) ) ;
#27476=CARTESIAN_POINT ( 'NONE',  ( 102.4999999999999858, 122.9883376334214091, 0.3865102666887284544 ) ) ;
#27489=FACE_OUTER_BOUND ( 'NONE', #2654, .T. ) ;
#27492=CARTESIAN_POINT ( 'NONE',  ( 99.99999999999998579, 101.5015231886685854, -50.87500000273119127 ) ) ;
#27493=CARTESIAN_POINT ( 'NONE',  ( 103.5355339059327235, 93.87500000000000000, 3.535533905932724874 ) ) ;
#27494=CARTESIAN_POINT ( 'NONE',  ( 101.4615807364564546, 124.4500000010924765, -1.461580736456474794 ) ) ;
#27498=EDGE_LOOP ( 'NONE', ( #3691, #3952 ) ) ;
#27513=EDGE_CURVE ( 'NONE', #2259, #3615, #1775, .T. ) ;
#27517=CARTESIAN_POINT ( 'NONE',  ( 99.99999999999998579, 94.06249999863440792, 4.458734124999981674 ) ) ;
#27523=CARTESIAN_POINT ( 'NONE',  ( 97.50000000000000000, 123.3499999999999943, -1.035533905932742416 ) ) ;
#27525=CARTESIAN_POINT ( 'NONE',  ( 102.1631189606246295, 103.3426043859339103, -47.90000000546238113 ) ) ;
#27526=CARTESIAN_POINT ( 'NONE',  ( 96.84719886470463734, 92.93749999863440792, -3.152801135295366208 ) ) ;
#27533=CARTESIAN_POINT ( 'NONE',  ( 103.1528011352953484, 91.18749999863440792, 3.152801135295352886 ) ) ;
#27539=CARTESIAN_POINT ( 'NONE',  ( 93.46109445667491400, 114.7507929638356785, -49.57500000273120122 ) ) ;
#27543=CARTESIAN_POINT ( 'NONE',  ( 108.0825317500000153, 110.0000000000000000, -48.12500000273119838 ) ) ;
#27547=ORIENTED_EDGE ( 'NONE', *, *, #23487, .T. ) ;
#27560=CARTESIAN_POINT ( 'NONE',  ( 104.4587341249999781, 94.56249999863440792, -6.938893903907228378E-15 ) ) ;
#27571=CARTESIAN_POINT ( 'NONE',  ( 99.99999999999998579, 117.3602355696678501, -54.50000000000000000 ) ) ;
#27581=VERTEX_POINT ( 'NONE', #2270 ) ;
#27605=CARTESIAN_POINT ( 'NONE',  ( 104.3262379212492590, 115.9545556584642867, -48.70000000000000284 ) ) ;
#27610=VECTOR ( 'NONE', #1214, 1000.000000000000000 ) ;
#27612=CARTESIAN_POINT ( 'NONE',  ( 99.99999999999998579, 123.2069999999781515, -2.499999999999997780 ) ) ;
#27615=CARTESIAN_POINT ( 'NONE',  ( 97.93301270000000613, 123.9500000010924765, -9.540979117872439019E-15 ) ) ;
#27620=CARTESIAN_POINT ( 'NONE',  ( 99.99999999999998579, 124.1000000021849416, -2.499999999999997780 ) ) ;
#27627=CARTESIAN_POINT ( 'NONE',  ( 95.00472066334982912, 116.8754121666685393, -47.67500000273120264 ) ) ;
#27629=CARTESIAN_POINT ( 'NONE',  ( 100.8561741729129153, 123.7000000010924765, -2.066987299999999195 ) ) ;
#27652=CARTESIAN_POINT ( 'NONE',  ( 96.84719886470463734, 94.68749999863440792, -3.152801135295366208 ) ) ;
#27656=PLANE ( 'NONE',  #8176 ) ;
#27660=CARTESIAN_POINT ( 'NONE',  ( 95.67376207875072680, 104.0454443415356991, -50.20000000546238539 ) ) ;
#27661=CARTESIAN_POINT ( 'NONE',  ( 99.99999999999998579, 94.81249999863440792, -4.458734124999994997 ) ) ;
#27675=CARTESIAN_POINT ( 'NONE',  ( 104.9952793366501851, 116.8754121666685393, -48.07500000273119412 ) ) ;
#27676=( BOUNDED_CURVE ( )  B_SPLINE_CURVE ( 2, ( #5442, #9705, #20553, #22544, #20693 ),
 .UNSPECIFIED., .F., .T. ) 
 B_SPLINE_CURVE_WITH_KNOTS ( ( 3, 2, 3 ),
 ( 0.000000000000000000, 0.04166666666666653945, 0.08333333333333307891 ),
 .UNSPECIFIED. ) 
 CURVE ( )  GEOMETRIC_REPRESENTATION_ITEM ( )  RATIONAL_B_SPLINE_CURVE ( ( 1.000000000000000000, 0.9238795325112867385, 1.000000000000000000, 0.9238795325112871826, 0.9999999999999995559 ) ) 
 REPRESENTATION_ITEM ( '' )  );
#27680=CARTESIAN_POINT ( 'NONE',  ( 108.0825317500000011, 107.3738262389971680, -48.22500000273118559 ) ) ;
#27681=CARTESIAN_POINT ( 'NONE',  ( 102.1631189606246295, 103.3426043859339103, -51.40000000000000568 ) ) ;
#27687=CIRCLE ( 'NONE', #27707, 5.000000000000004441 ) ;
#27699=CARTESIAN_POINT ( 'NONE',  ( 98.53841926354351699, 123.6500000010924794, -1.461580736456474794 ) ) ;
#27700=CARTESIAN_POINT ( 'NONE',  ( 99.99999999999998579, 94.81249999863440792, -4.458734124999994997 ) ) ;
#27703=CARTESIAN_POINT ( 'NONE',  ( 95.00000000000000000, 93.43749999999998579, -2.071067811865479058 ) ) ;
#27707=AXIS2_PLACEMENT_3D ( 'NONE', #7092, #9662, #27215 ) ;
#27709=EDGE_LOOP ( 'NONE', ( #20372, #24203, #25006, #25864 ) ) ;
#27714=( BOUNDED_CURVE ( )  B_SPLINE_CURVE ( 2, ( #776, #26862, #27002, #5189, #13852, #22577, #3046, #11715, #9591 ),
 .UNSPECIFIED., .F., .F. ) 
 B_SPLINE_CURVE_WITH_KNOTS ( ( 3, 2, 2, 2, 3 ),
 ( 0.08333333333333389770, 0.1250000000000003886, 0.1666666666666668517, 0.2083333333333333426, 0.2499999999999998335 ),
 .UNSPECIFIED. ) 
 CURVE ( )  GEOMETRIC_REPRESENTATION_ITEM ( )  RATIONAL_B_SPLINE_CURVE ( ( 0.9999999999999990008, 0.9238795325112877377, 1.000000000000000000, 0.9238795325112867385, 1.000000000000000000, 0.9238795325112867385, 1.000000000000000000, 0.9238795325112870716, 0.9999999999999996669 ) ) 
 REPRESENTATION_ITEM ( '' )  );
#27721=EDGE_CURVE ( 'NONE', #18097, #28082, #986, .T. ) ;
#27726=FACE_OUTER_BOUND ( 'NONE', #22926, .T. ) ;
#27731=FACE_OUTER_BOUND ( 'NONE', #6548, .T. ) ;
#27749=CARTESIAN_POINT ( 'NONE',  ( 97.50000000000000000, 125.0000000000000000, -9.540979117872439019E-15 ) ) ;
#27751=CARTESIAN_POINT ( 'NONE',  ( 99.99999999999998579, 124.1500000010924651, 2.066987299999980099 ) ) ;
#27755=CARTESIAN_POINT ( 'NONE',  ( 107.0000000000000142, 110.0000000000000000, -53.00000000000000711 ) ) ;
#27764=CARTESIAN_POINT ( 'NONE',  ( 102.4976396683250925, 117.6869444889999841, -45.97500000273119269 ) ) ;
#27765=CARTESIAN_POINT ( 'NONE',  ( 100.0000000000000000, 110.0000000000000000, -55.00000000000000711 ) ) ;
#27766=CARTESIAN_POINT ( 'NONE',  ( 100.8561741729129295, 123.4000000010924794, 2.066987299999979211 ) ) ;
#27774=CARTESIAN_POINT ( 'NONE',  ( 95.00000000000000000, 94.56250000000000000, 2.071067811865463959 ) ) ;
#27788=CARTESIAN_POINT ( 'NONE',  ( 95.54126587499999346, 94.87499999863440792, 1.846868145590722543 ) ) ;
#27789=( BOUNDED_SURFACE ( )  B_SPLINE_SURFACE ( 1, 2, ( 
 ( #14076, #26648, #11791, #20515, #16221, #997, #9665, #18369, #4982, #9806, #22796, #25066, #7096, #15794, #22363, #24497, #11505, #20223, #706, #9380, #18077, #26791, #7236, #24646, #5119, #13784, #22506, #20370, #25201, #1414, #7815, #6094, #25610, #1555, #10208, #27492, #23621, #23069, #3546, #14493, #23481, #27901, #12349, #25338, #18785, #12621, #25751, #16645, #23345, #20930, #16781, #3818, #12203, #21205, #14900, #12478, #5824, #18918, #9937, #12068, #7948, #3961, #1688, #21347, #23210, #20792, #1273, #27627, #25480, #10073, #3685, #1825, #19198, #21067, #10491, #8085, #10347, #5687, #27358, #14626, #5958, #16912, #19054, #14761, #27764, #18652, #16507, #8361, #8222, #17047, #6233, #14353, #26320, #4516, #15466, #12761, #11045, #8924, #28038, #2521, #17612 ),
 ( #19755, #12892, #19900, #24037, #4658, #384, #9068, #6781, #24180, #15039, #13031, #13320, #25897, #21768, #19616, #8505, #22045, #11182, #26172, #21622, #6920, #21481, #17763, #26466, #15613, #26030, #2245, #10907, #6367, #1961, #4098, #237, #2098, #10630, #13173, #19336, #17190, #23756, #4234, #10766, #19477, #101, #28176, #8647, #8783, #17470, #17337, #6501, #15177, #23896, #4375, #6639, #15324, #21912, #2387, #24607, #18332, #27039, #7485, #16180, #671, #18475, #24745, #5367, #11753, #816, #9345, #9484, #26610, #5085, #11606, #11891, #24888, #22616, #14034, #957, #7195, #22759, #18186, #22330, #526, #22472, #15755, #13747, #2665, #15891, #27183, #11326, #4943, #3224, #24315, #7056, #9627, #7634, #26896, #20615, #2935, #20187, #22185, #9766, #20329 ) ),
 .UNSPECIFIED., .F., .F., .F. ) 
 B_SPLINE_SURFACE_WITH_KNOTS ( ( 2, 2 ),
 ( 3, 2, 2, 2, 2, 2, 2, 2, 2, 2, 2, 2, 2, 2, 2, 2, 2, 2, 2, 2, 2, 2, 2, 2, 2, 2, 2, 2, 2, 2, 2, 2, 2, 2, 2, 2, 2, 2, 2, 2, 2, 2, 2, 2, 2, 2, 2, 2, 2, 2, 3 ),
 ( 0.000000000000000000, 1.000000000000000000 ),
 ( 0.000000000000000000, 0.02000000000000000042, 0.04000000000000000083, 0.05999999999999999778, 0.08000000000000000167, 0.1000000000000000056, 0.1199999999999999956, 0.1400000000000000133, 0.1600000000000000033, 0.1799999999999999933, 0.2000000000000000111, 0.2200000000000000011, 0.2399999999999999911, 0.2600000000000000089, 0.2800000000000000266, 0.2999999999999999889, 0.3200000000000000067, 0.3400000000000000244, 0.3599999999999999867, 0.3800000000000000044, 0.4000000000000000222, 0.4199999999999999845, 0.4400000000000000022, 0.4600000000000000200, 0.4799999999999999822, 0.5000000000000000000, 0.5200000000000000178, 0.5400000000000000355, 0.5600000000000000533, 0.5799999999999999600, 0.5999999999999999778, 0.6199999999999999956, 0.6400000000000000133, 0.6600000000000000311, 0.6800000000000000488, 0.6999999999999999556, 0.7199999999999999734, 0.7399999999999999911, 0.7600000000000000089, 0.7800000000000000266, 0.8000000000000000444, 0.8199999999999999512, 0.8399999999999999689, 0.8599999999999999867, 0.8800000000000000044, 0.9000000000000000222, 0.9200000000000000400, 0.9399999999999999467, 0.9599999999999999645, 0.9799999999999999822, 1.000000000000000000 ),
 .UNSPECIFIED. ) 
 GEOMETRIC_REPRESENTATION_ITEM ( )  RATIONAL_B_SPLINE_SURFACE ( (
 ( 1.000000000000000000, 0.9510565162951535312, 1.000000000000000000, 0.9510565162951535312, 1.000000000000000000, 0.9510565162951535312, 1.000000000000000000, 0.9510565162951535312, 1.000000000000000000, 0.9510565162951535312, 1.000000000000000000, 0.9510565162951535312, 1.000000000000000000, 0.9510565162951535312, 1.000000000000000000, 0.9510565162951535312, 1.000000000000000000, 0.9510565162951535312, 1.000000000000000000, 0.9510565162951535312, 1.000000000000000000, 0.9510565162951535312, 1.000000000000000000, 0.9510565162951535312, 1.000000000000000000, 0.9510565162951535312, 1.000000000000000000, 0.9510565162951535312, 1.000000000000000000, 0.9510565162951535312, 1.000000000000000000, 0.9510565162951535312, 1.000000000000000000, 0.9510565162951535312, 1.000000000000000000, 0.9510565162951535312, 1.000000000000000000, 0.9510565162951535312, 1.000000000000000000, 0.9510565162951535312, 1.000000000000000000, 0.9510565162951535312, 1.000000000000000000, 0.9510565162951535312, 1.000000000000000000, 0.9510565162951535312, 1.000000000000000000, 0.9510565162951535312, 1.000000000000000000, 0.9510565162951535312, 1.000000000000000000, 0.9510565162951535312, 1.000000000000000000, 0.9510565162951535312, 1.000000000000000000, 0.9510565162951535312, 1.000000000000000000, 0.9510565162951535312, 1.000000000000000000, 0.9510565162951535312, 1.000000000000000000, 0.9510565162951535312, 1.000000000000000000, 0.9510565162951535312, 1.000000000000000000, 0.9510565162951535312, 1.000000000000000000, 0.9510565162951535312, 1.000000000000000000, 0.9510565162951535312, 1.000000000000000000, 0.9510565162951535312, 1.000000000000000000, 0.9510565162951535312, 1.000000000000000000, 0.9510565162951535312, 1.000000000000000000, 0.9510565162951535312, 1.000000000000000000, 0.9510565162951535312, 1.000000000000000000, 0.9510565162951535312, 1.000000000000000000, 0.9510565162951535312, 1.000000000000000000, 0.9510565162951535312, 1.000000000000000000, 0.9510565162951535312, 1.000000000000000000, 0.9510565162951535312, 1.000000000000000000, 0.9510565162951535312, 1.000000000000000000, 0.9510565162951535312, 1.000000000000000000, 0.9510565162951535312, 1.000000000000000000, 0.9510565162951535312, 1.000000000000000000, 0.9510565162951535312, 1.000000000000000000),
 ( 1.000000000000000000, 0.9510565162951535312, 1.000000000000000000, 0.9510565162951535312, 1.000000000000000000, 0.9510565162951535312, 1.000000000000000000, 0.9510565162951535312, 1.000000000000000000, 0.9510565162951535312, 1.000000000000000000, 0.9510565162951535312, 1.000000000000000000, 0.9510565162951535312, 1.000000000000000000, 0.9510565162951535312, 1.000000000000000000, 0.9510565162951535312, 1.000000000000000000, 0.9510565162951535312, 1.000000000000000000, 0.9510565162951535312, 1.000000000000000000, 0.9510565162951535312, 1.000000000000000000, 0.9510565162951535312, 1.000000000000000000, 0.9510565162951535312, 1.000000000000000000, 0.9510565162951535312, 1.000000000000000000, 0.9510565162951535312, 1.000000000000000000, 0.9510565162951535312, 1.000000000000000000, 0.9510565162951535312, 1.000000000000000000, 0.9510565162951535312, 1.000000000000000000, 0.9510565162951535312, 1.000000000000000000, 0.9510565162951535312, 1.000000000000000000, 0.9510565162951535312, 1.000000000000000000, 0.9510565162951535312, 1.000000000000000000, 0.9510565162951535312, 1.000000000000000000, 0.9510565162951535312, 1.000000000000000000, 0.9510565162951535312, 1.000000000000000000, 0.9510565162951535312, 1.000000000000000000, 0.9510565162951535312, 1.000000000000000000, 0.9510565162951535312, 1.000000000000000000, 0.9510565162951535312, 1.000000000000000000, 0.9510565162951535312, 1.000000000000000000, 0.9510565162951535312, 1.000000000000000000, 0.9510565162951535312, 1.000000000000000000, 0.9510565162951535312, 1.000000000000000000, 0.9510565162951535312, 1.000000000000000000, 0.9510565162951535312, 1.000000000000000000, 0.9510565162951535312, 1.000000000000000000, 0.9510565162951535312, 1.000000000000000000, 0.9510565162951535312, 1.000000000000000000, 0.9510565162951535312, 1.000000000000000000, 0.9510565162951535312, 1.000000000000000000, 0.9510565162951535312, 1.000000000000000000, 0.9510565162951535312, 1.000000000000000000, 0.9510565162951535312, 1.000000000000000000, 0.9510565162951535312, 1.000000000000000000, 0.9510565162951535312, 1.000000000000000000, 0.9510565162951535312, 1.000000000000000000, 0.9510565162951535312, 1.000000000000000000, 0.9510565162951535312, 1.000000000000000000, 0.9510565162951535312, 1.000000000000000000) ) ) 
 REPRESENTATION_ITEM ( '' )  SURFACE ( )  );
#27801=CARTESIAN_POINT ( 'NONE',  ( 101.8468681455907330, 92.74999999863439371, -4.458734124999994997 ) ) ;
#27804=CARTESIAN_POINT ( 'NONE',  ( 97.83688103937537051, 103.3426043859339103, -45.60000000000000853 ) ) ;
#27808=CARTESIAN_POINT ( 'NONE',  ( 96.84719886470463734, 90.93749999863440792, 3.152801135295351997 ) ) ;
#27841=LINE ( 'NONE', #23698, #21667 ) ;
#27850=CARTESIAN_POINT ( 'NONE',  ( 94.33688103937537051, 105.8855032339526758, -49.80000000000000426 ) ) ;
#27851=FACE_OUTER_BOUND ( 'NONE', #17213, .T. ) ;
#27852=CARTESIAN_POINT ( 'NONE',  ( 102.0669872999999797, 123.5500000010924708, -9.794112055954760458E-15 ) ) ;
#27862=CARTESIAN_POINT ( 'NONE',  ( 99.99999999999998579, 92.12499999726880162, -4.999999999999997335 ) ) ;
#27866=FACE_OUTER_BOUND ( 'NONE', #25414, .T. ) ;
#27868=CARTESIAN_POINT ( 'NONE',  ( 102.0710678118654897, 93.68749999726880162, 4.999999999999953815 ) ) ;
#27869=EDGE_LOOP ( 'NONE', ( #19798, #19309, #11622, #26080 ) ) ;
#27872=( BOUNDED_CURVE ( )  B_SPLINE_CURVE ( 2, ( #25432, #27171, #14301, #12154, #27434, #7624, #7899, #16593, #25287, #5915, #5772, #14443, #4186, #6456, #12715, #23711, #16869 ),
 .UNSPECIFIED., .F., .F. ) 
 B_SPLINE_CURVE_WITH_KNOTS ( ( 3, 2, 2, 2, 2, 2, 2, 2, 3 ),
 ( 0.8500000005328695041, 0.8599999999999999867, 0.8800000000000000044, 0.9000000000000000222, 0.9200000000000000400, 0.9399999999999999467, 0.9599999999999999645, 0.9799999999999999822, 1.000000000000000000 ),
 .UNSPECIFIED. ) 
 CURVE ( )  GEOMETRIC_REPRESENTATION_ITEM ( )  RATIONAL_B_SPLINE_CURVE ( ( 0.9755282581475768211, 0.9755282594516012651, 1.000000000000000000, 0.9510565162951535312, 1.000000000000000000, 0.9510565162951535312, 1.000000000000000000, 0.9510565162951535312, 1.000000000000000000, 0.9510565162951535312, 1.000000000000000000, 0.9510565162951535312, 1.000000000000000000, 0.9510565162951535312, 1.000000000000000000, 0.9510565162951535312, 1.000000000000000000 ) ) 
 REPRESENTATION_ITEM ( '' )  );
#27884=LINE ( 'NONE', #17031, #11536 ) ;
#27885=CARTESIAN_POINT ( 'NONE',  ( 102.4999999999999716, 124.6500000000000199, -1.035533905932742638 ) ) ;
#27887=CARTESIAN_POINT ( 'NONE',  ( 101.4615807364564546, 123.4500000010924765, 1.461580736456455476 ) ) ;
#27889=ORIENTED_EDGE ( 'NONE', *, *, #12602, .F. ) ;
#27891=CARTESIAN_POINT ( 'NONE',  ( 93.00000000000000000, 110.0000000000000000, -48.50000000546238255 ) ) ;
#27893=CARTESIAN_POINT ( 'NONE',  ( 101.7677669529663547, 124.0000000021849615, -1.767766952966370209 ) ) ;
#27901=CARTESIAN_POINT ( 'NONE',  ( 108.0825317500000011, 112.6261737610028320, -50.27500000273119696 ) ) ;
#27903=CARTESIAN_POINT ( 'NONE',  ( 102.0669872999999939, 122.8000000010924708, -0.8561741729129507261 ) ) ;
#27907=ORIENTED_EDGE ( 'NONE', *, *, #8942, .F. ) ;
#27930=CARTESIAN_POINT ( 'NONE',  ( 84.99999999999998579, 118.0000000000000000, -15.00000000000000533 ) ) ;
#27934=CARTESIAN_POINT ( 'NONE',  ( 100.0000000000000000, 110.0000000000000000, -55.00000000000000711 ) ) ;
#27935=CARTESIAN_POINT ( 'NONE',  ( 95.54126587500000767, 92.81249999863440792, -7.484931351350258973E-15 ) ) ;
#27968=CARTESIAN_POINT ( 'NONE',  ( 97.50236033167492167, 117.6869444889999841, -49.52500000273119696 ) ) ;
#27977=DIRECTION ( 'NONE',  ( 5.782411586589357392E-17, -0.000000000000000000, 1.000000000000000000 ) ) ;
#27986=ORIENTED_EDGE ( 'NONE', *, *, #2022, .F. ) ;
#27987=CARTESIAN_POINT ( 'NONE',  ( 93.00000000000000000, 110.0000000000000000, -50.00000000000000711 ) ) ;
#27988=VECTOR ( 'NONE', #20908, 1000.000000000000000 ) ;
#27990=CARTESIAN_POINT ( 'NONE',  ( 99.99999999999998579, 123.7500000010924737, -2.066987299999998751 ) ) ;
#28004=LINE ( 'NONE', #21031, #12614 ) ;
#28006=CARTESIAN_POINT ( 'NONE',  ( 107.0000000000000142, 110.0000000000000000, -51.50000000546237544 ) ) ;
#28007=CARTESIAN_POINT ( 'NONE',  ( 107.0000000000000142, 110.0000000000000000, -49.00000000000000711 ) ) ;
#28012=VECTOR ( 'NONE', #11390, 1000.000000000000000 ) ;
#28017=LINE ( 'NONE', #24160, #21167 ) ;
#28020=FACE_OUTER_BOUND ( 'NONE', #1322, .T. ) ;
#28025=CARTESIAN_POINT ( 'NONE',  ( 101.0355339059327378, 123.2500000021849758, -2.499999999999997780 ) ) ;
#28038=CARTESIAN_POINT ( 'NONE',  ( 106.5389055433251002, 105.2492070361643215, -44.57500000273119412 ) ) ;
#28068=CARTESIAN_POINT ( 'NONE',  ( 91.91746824999998466, 112.6261737610028320, -47.47500000273119269 ) ) ;
#28073=CARTESIAN_POINT ( 'NONE',  ( 93.00000000000001421, 107.7255621263696668, -44.40000000546238113 ) ) ;
#28074=CARTESIAN_POINT ( 'NONE',  ( 95.54126587500000767, 91.81249999863440792, -7.484931351350258973E-15 ) ) ;
#28081=CARTESIAN_POINT ( 'NONE',  ( 95.54126587500000767, 91.81249999863440792, -7.484931351350258973E-15 ) ) ;
#28082=VERTEX_POINT ( 'NONE', #11921 ) ;
#28095=CARTESIAN_POINT ( 'NONE',  ( 93.00000000000000000, 110.0000000000000000, -48.50000000546238255 ) ) ;
#28106=CARTESIAN_POINT ( 'NONE',  ( 95.00472066334982912, 116.8754121666685393, -53.42500000273118843 ) ) ;
#28113=EDGE_CURVE ( 'NONE', #12986, #5360, #23710, .T. ) ;
#28116=FACE_OUTER_BOUND ( 'NONE', #10266, .T. ) ;
#28123=ORIENTED_EDGE ( 'NONE', *, *, #8313, .F. ) ;
#28124=CARTESIAN_POINT ( 'NONE',  ( 97.83688103937537051, 103.3426043859339103, -53.60000000000000853 ) ) ;
#28126=CARTESIAN_POINT ( 'NONE',  ( 100.8561741729129295, 124.2000000010924907, 2.066987299999979211 ) ) ;
#28141=CARTESIAN_POINT ( 'NONE',  ( 84.99999999999998579, 123.0000000000000000, 14.99999999999999112 ) ) ;
#28146=VECTOR ( 'NONE', #15354, 1000.000000000000000 ) ;
#28155=CARTESIAN_POINT ( 'NONE',  ( 105.6631189606246295, 105.8855032339526758, -45.70000000546237828 ) ) ;
#28160=CARTESIAN_POINT ( 'NONE',  ( 102.4976396683250925, 117.6869444889999841, -51.72500000273119980 ) ) ;
#28176=CARTESIAN_POINT ( 'NONE',  ( 106.5389055433251002, 114.7507929638356785, -49.92500000273119554 ) ) ;
#28177=DIRECTION ( 'NONE',  ( 5.782411586589357392E-17, -0.000000000000000000, 1.000000000000000000 ) ) ;
#28178=DIRECTION ( 'NONE',  ( 0.8660254037844418162, 0.000000000000000000, 0.4999999999999947264 ) ) ;
#28183=ORIENTED_EDGE ( 'NONE', *, *, #21706, .T. ) ;
#28194=VERTEX_POINT ( 'NONE', #15027 ) ;
ENDSEC;
END-ISO-10303-21;
